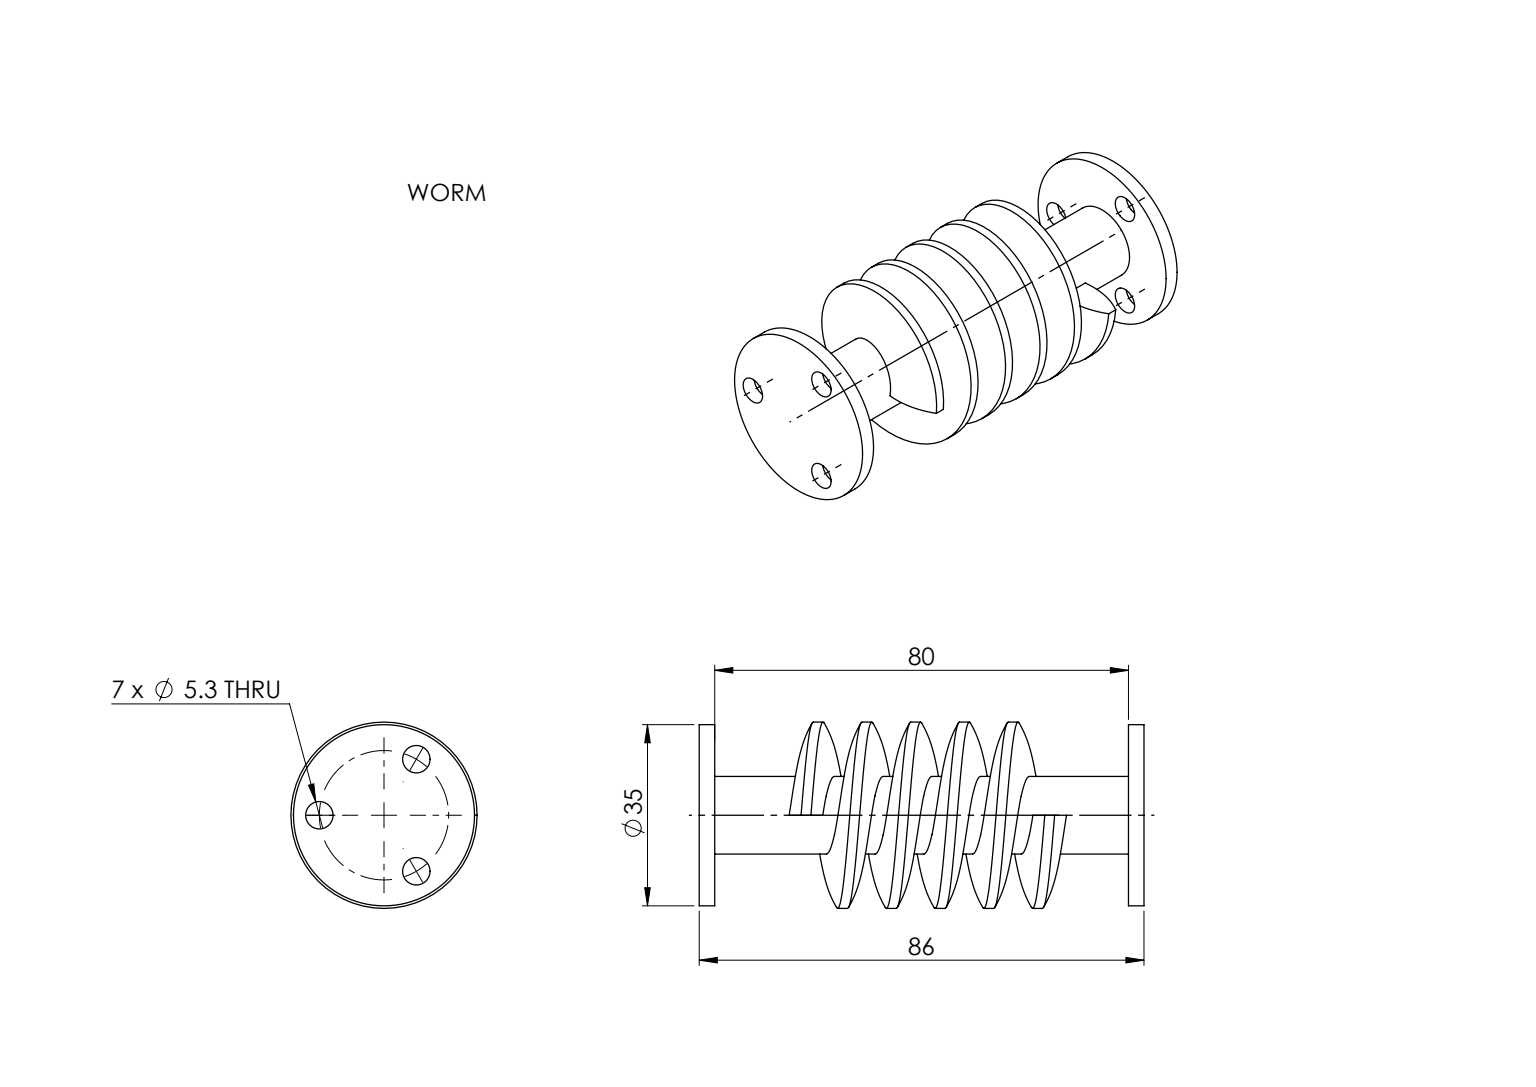
ISO-10303-21;
HEADER;
FILE_DESCRIPTION (('STEP AP214'),
    '1' );
FILE_NAME ('worm.step',
    '2026-10-03T12:29:21',
    ( '' ),
    ( '' ),
    'SwSTEP 2.0',
    'SolidWorks 2026',
    '' );
FILE_SCHEMA (( 'AUTOMOTIVE_DESIGN' ));
ENDSEC;

DATA;
#2=CARTESIAN_POINT ( 'NONE',  ( -6.358192987158596488, 4.248408730893249441, 12.23479375018031590 ) ) ;
#4=CARTESIAN_POINT ( 'NONE',  ( 11.17563879758427525, 2.222972768810836719, -0.3496410002868030609 ) ) ;
#8=DIRECTION ( 'NONE',  ( 0.000000000000000000, 0.000000000000000000, 1.000000000000000000 ) ) ;
#13=CARTESIAN_POINT ( 'NONE',  ( 16.62983158437509346, -6.888301784570739272, 14.47261250018031298 ) ) ;
#31=CARTESIAN_POINT ( 'NONE',  ( -6.358192987158591158, 4.248408730893245000, 5.969893750180312431 ) ) ;
#34=CARTESIAN_POINT ( 'NONE',  ( 6.358192987158596488, -4.248408730893249441, -1.902706249819686279 ) ) ;
#36=CARTESIAN_POINT ( 'NONE',  ( 0.000000000000000000, 0.000000000000000000, 40.00000000000000000 ) ) ;
#40=DIRECTION ( 'NONE',  ( -0.000000000000000000, -0.000000000000000000, -1.000000000000000000 ) ) ;
#43=PLANE ( 'NONE',  #3162 ) ;
#52=CARTESIAN_POINT ( 'NONE',  ( 14.79893867793684059, 2.943691925285398359, -12.82923933115845649 ) ) ;
#57=EDGE_LOOP ( 'NONE', ( #4970, #17934 ) ) ;
#61=CARTESIAN_POINT ( 'NONE',  ( -15.25966317163203279, -10.19618095047498052, 17.71245625018031689 ) ) ;
#69=ORIENTED_EDGE ( 'NONE', *, *, #783, .F. ) ;
#72=CARTESIAN_POINT ( 'NONE',  ( 1.491842756249030399, 7.499999999820669672, -4.848018749819687834 ) ) ;
#76=AXIS2_PLACEMENT_3D ( 'NONE', #4116, #10601, #17063 ) ;
#80=CARTESIAN_POINT ( 'NONE',  ( 3.580422614997669228, 17.99999999956958874, -7.028168749819693417 ) ) ;
#83=CARTESIAN_POINT ( 'NONE',  ( -13.67243654778935102, -5.663308646854334327, -4.604354418480926192 ) ) ;
#94=ORIENTED_EDGE ( 'NONE', *, *, #11160, .T. ) ;
#100=VERTEX_POINT ( 'NONE', #5055 ) ;
#108=CARTESIAN_POINT ( 'NONE',  ( 7.500000000000007994, -9.015933403756345817E-10, 16.06370000018031519 ) ) ;
#110=CARTESIAN_POINT ( 'NONE',  ( -7.902369976724391343, 7.902369978624323110, -3.589484750286802139 ) ) ;
#115=CARTESIAN_POINT ( 'NONE',  ( 3.580422614997668340, 17.99999999956958519, 21.24683125018031404 ) ) ;
#131=AXIS2_PLACEMENT_3D ( 'NONE', #20801, #1327, #6175 ) ;
#135=CARTESIAN_POINT ( 'NONE',  ( 6.358192988180013216, 4.248408729364577141, 8.915206250180313319 ) ) ;
#142=CARTESIAN_POINT ( 'NONE',  ( -10.19618095047498052, 15.25966317163203101, 18.16410625018031411 ) ) ;
#156=CARTESIAN_POINT ( 'NONE',  ( 14.79893867722910450, -2.943691928843438443, -21.66517683115846182 ) ) ;
#174=CARTESIAN_POINT ( 'NONE',  ( 3.580422610670019878, -18.00000000043040771, -23.65933124981969016 ) ) ;
#177=CARTESIAN_POINT ( 'NONE',  ( 7.500000000000005329, -1.491842755816077393, -11.91676874991220814 ) ) ;
#181=( BOUNDED_SURFACE ( )  B_SPLINE_SURFACE ( 3, 2, ( 
 ( #15242, #3787, #10269, #14938, #18223, #10163, #15145, #724, #8565, #15045, #7180, #2419, #20112, #5588, #10480, #8880, #15353, #840, #7288, #20223, #5698, #2009, #8458, #415, #19801, #11758, #3688, #525, #10588, #12389, #19166, #10700, #7396, #13983, #7499, #17264, #953, #20642, #4431, #1375, #14091, #20319, #7820, #14300, #10899, #18755, #20742, #2956, #17050, #20545, #11002, #18960, #15464, #13872, #17372, #6229, #17163, #6121, #6028, #4541, #2736, #2648, #4336, #12599, #20438, #15878, #5920, #12498, #9205, #19066, #10803, #4224, #17479, #5803, #2537, #18861, #9423, #15665, #1165, #2844, #7613, #9311, #9104, #15774, #12280, #15556, #1276, #12714, #7727, #8994, #1052, #14200, #1778, #4745, #13122, #17792, #9820, #6336, #4647, #14602, #19572, #12822, #16391, #80, #17688, #13019, #3358, #3456, #16196, #16092, #1878, #287, #1683, #5049, #19266, #9516, #3258, #6736, #8232, #9923, #14710, #4852, #20850, #11115, #182, #9728, #1583, #8130, #7931, #8037, #8336, #3157, #6430, #14732, #11212, #16287, #17985, #17586, #6534, #1483, #13219, #12913, #14814, #11512, #19365, #19471, #3054, #6637, #9629, #4953, #15981, #14408, #11323, #11423, #17896, #14513, #5561, #13532, #384, #608, #3977 ),
 ( #813, #3666, #5147, #8432, #501, #10348, #15327, #16915, #13325, #7052, #10457, #11621, #13635, #3757, #8752, #19976, #10138, #16590, #18095, #6840, #19779, #6949, #11829, #5261, #18201, #8536, #20082, #10239, #2079, #15218, #5456, #18293, #11928, #12042, #15017, #18513, #13434, #2395, #19887, #5361, #16701, #3560, #18402, #19667, #2186, #7259, #11730, #16505, #8643, #8852, #15121, #3869, #16813, #700, #2299, #7152, #10037, #14908, #1984, #9079, #2817, #5895, #2616, #7588, #15531, #1025, #5775, #20517, #15431, #8966, #17238, #2927, #2510, #4403, #20194, #10871, #12145, #17342, #4077, #1350, #12367, #15636, #921, #20616, #13847, #7370, #7471, #20291, #17454, #18833, #9397, #4307, #5674, #10777, #2710, #12248, #13953, #15857, #18723, #18614, #4197, #20408, #9287, #13740, #10978, #10675, #1136, #19036, #10557, #7700, #9177, #15748, #14066, #17133, #5999, #17023, #12471, #18935, #1247, #14176, #6092, #12569, #4512, #8205, #12891, #4722, #3337, #16172, #6407, #52, #14684, #11187, #1753, #9596, #19550, #19244, #17659, #16064, #14268, #8110, #7794, #1557, #16368, #7902, #4619, #3127, #8009, #14489, #19145, #17874, #1661, #5030, #11291, #17564, #11491, #17963, #14582, #15950, #3432, #156, #20713 ),
 ( #6506, #9900, #14384, #9797, #17766, #6609, #20929, #20825, #19339, #16266, #4822, #6203, #3232, #12688, #6307, #11091, #9703, #12992, #19445, #3031, #13094, #4926, #9491, #11395, #1450, #12798, #5539, #16678, #10008, #12017, #15197, #10434, #11807, #2272, #10215, #6715, #19644, #2167, #18484, #8411, #18375, #18270, #16784, #14991, #1960, #16568, #11902, #5237, #7127, #18175, #5339, #479, #3845, #2055, #16477, #8731, #18071, #8310, #3642, #10324, #6926, #11707, #8621, #10116, #8510, #14884, #15095, #3536, #361, #3735, #3951, #11596, #13512, #14785, #19955, #264, #5433, #13196, #1856, #13410, #583, #6814, #675, #13298, #19756, #19862, #7033, #5122, #13608, #20055, #1305, #8824, #7748, #9337, #15408, #18696, #19287, #894, #2371, #5650, #4169, #7848, #12843, #14436, #10535, #19097, #1512, #15297, #11138, #14221, #6259, #4570, #7348, #13829, #785, #18593, #16994, #10652, #15801, #2480, #20272, #5750, #17608, #20666, #12226, #12743, #11032, #6148, #9444, #3078, #17107, #9541, #2871, #7963, #12636, #17509, #2983, #7234, #15902, #1400, #19196, #14331, #20776, #4676, #16012, #20881, #6363, #4770, #16894, #13717, #20164, #12125, #4053, #8942, #11237, #13045, #19804, #11351, #8068, #14629, #8156 ),
 ( #19699, #3383, #16418, #12942, #17715, #212, #5180, #19393, #2012, #6669, #3294, #19602, #9954, #10066, #1809, #1707, #8461, #6871, #8261, #11650, #4882, #16123, #9849, #13357, #8369, #16528, #14841, #11455, #6457, #3188, #6767, #16314, #108, #14735, #14537, #6563, #14942, #9758, #19499, #4987, #17823, #1905, #3590, #9657, #13152, #2, #1615, #17923, #418, #18122, #5076, #11542, #16223, #315, #18013, #3480, #13248, #15359, #5486, #7077, #12076, #15047, #12173, #20116, #6975, #7183, #10591, #8571, #958, #528, #18226, #13667, #5700, #18546, #13777, #16624, #10379, #2321, #16844, #7398, #11965, #15244, #2216, #13464, #8674, #7294, #18435, #13556, #15147, #8775, #13876, #632, #5594, #4001, #20227, #10164, #3898, #18323, #15467, #727, #19908, #10483, #2421, #5386, #18639, #16939, #8882, #11855, #5288, #842, #4107, #3790, #17054, #2540, #10273, #8999, #11760, #3692, #2112, #16736, #20004, #15983, #10900, #20745, #13984, #4225, #12499, #1485, #17480, #19168, #2958, #20547, #15560, #20320, #15879, #18963, #10805, #17374, #2650, #17269, #11116, #12392, #1169, #15666, #20443, #11003, #12716, #5805, #9312, #17166, #7936, #7614, #3055, #7821, #14093, #4434, #4650, #9424, #5921, #2847, #1376 ) ),
 .UNSPECIFIED., .F., .F., .F. ) 
 B_SPLINE_SURFACE_WITH_KNOTS ( ( 4, 4 ),
 ( 3, 2, 2, 2, 2, 2, 2, 2, 2, 2, 2, 2, 2, 2, 2, 2, 2, 2, 2, 2, 2, 2, 2, 2, 2, 2, 2, 2, 2, 2, 2, 2, 2, 2, 2, 2, 2, 2, 2, 2, 2, 2, 2, 2, 2, 2, 2, 2, 2, 2, 2, 2, 2, 2, 2, 2, 2, 2, 2, 2, 2, 2, 2, 2, 2, 2, 2, 2, 2, 2, 2, 2, 2, 2, 2, 2, 2, 2, 2, 2, 3 ),
 ( 0.000000000000000000, 1.000000000000000000 ),
 ( 0.000000000000000000, 0.01250000000000000069, 0.02500000000000000139, 0.03749999999999999861, 0.05000000000000000278, 0.06250000000000000000, 0.07499999999999999722, 0.08749999999999999445, 0.1000000000000000056, 0.1125000000000000028, 0.1250000000000000000, 0.1375000000000000111, 0.1499999999999999944, 0.1625000000000000056, 0.1749999999999999889, 0.1875000000000000000, 0.2000000000000000111, 0.2124999999999999944, 0.2250000000000000056, 0.2374999999999999889, 0.2500000000000000000, 0.2625000000000000111, 0.2750000000000000222, 0.2874999999999999778, 0.2999999999999999889, 0.3125000000000000000, 0.3250000000000000111, 0.3375000000000000222, 0.3499999999999999778, 0.3624999999999999889, 0.3750000000000000000, 0.3875000000000000111, 0.4000000000000000222, 0.4124999999999999778, 0.4249999999999999889, 0.4375000000000000000, 0.4500000000000000111, 0.4625000000000000222, 0.4749999999999999778, 0.4874999999999999889, 0.5000000000000000000, 0.5124999999999999556, 0.5250000000000000222, 0.5374999999999999778, 0.5500000000000000444, 0.5625000000000000000, 0.5749999999999999556, 0.5875000000000000222, 0.5999999999999999778, 0.6125000000000000444, 0.6250000000000000000, 0.6374999999999999556, 0.6500000000000000222, 0.6624999999999999778, 0.6750000000000000444, 0.6875000000000000000, 0.6999999999999999556, 0.7125000000000000222, 0.7249999999999999778, 0.7375000000000000444, 0.7500000000000000000, 0.7624999999999999556, 0.7750000000000000222, 0.7874999999999999778, 0.8000000000000000444, 0.8125000000000000000, 0.8249999999999999556, 0.8375000000000000222, 0.8499999999999999778, 0.8625000000000000444, 0.8750000000000000000, 0.8874999999999999556, 0.9000000000000000222, 0.9124999999999999778, 0.9250000000000000444, 0.9375000000000000000, 0.9499999999999999556, 0.9625000000000000222, 0.9749999999999999778, 0.9875000000000000444, 1.000000000000000000 ),
 .UNSPECIFIED. ) 
 GEOMETRIC_REPRESENTATION_ITEM ( )  RATIONAL_B_SPLINE_SURFACE ( (
 ( 1.000000000000000000, 0.9807852804032304306, 1.000000000000000000, 0.9807852804032304306, 1.000000000000000000, 0.9807852804032304306, 1.000000000000000000, 0.9807852804032304306, 1.000000000000000000, 0.9807852804032304306, 1.000000000000000000, 0.9807852804032304306, 1.000000000000000000, 0.9807852804032304306, 1.000000000000000000, 0.9807852804032304306, 1.000000000000000000, 0.9807852804032304306, 1.000000000000000000, 0.9807852804032304306, 1.000000000000000000, 0.9807852804032304306, 1.000000000000000000, 0.9807852804032304306, 1.000000000000000000, 0.9807852804032304306, 1.000000000000000000, 0.9807852804032304306, 1.000000000000000000, 0.9807852804032304306, 1.000000000000000000, 0.9807852804032304306, 1.000000000000000000, 0.9807852804032304306, 1.000000000000000000, 0.9807852804032304306, 1.000000000000000000, 0.9807852804032304306, 1.000000000000000000, 0.9807852804032304306, 1.000000000000000000, 0.9807852804032304306, 1.000000000000000000, 0.9807852804032304306, 1.000000000000000000, 0.9807852804032304306, 1.000000000000000000, 0.9807852804032304306, 1.000000000000000000, 0.9807852804032304306, 1.000000000000000000, 0.9807852804032304306, 1.000000000000000000, 0.9807852804032304306, 1.000000000000000000, 0.9807852804032304306, 1.000000000000000000, 0.9807852804032304306, 1.000000000000000000, 0.9807852804032304306, 1.000000000000000000, 0.9807852804032304306, 1.000000000000000000, 0.9807852804032304306, 1.000000000000000000, 0.9807852804032304306, 1.000000000000000000, 0.9807852804032304306, 1.000000000000000000, 0.9807852804032304306, 1.000000000000000000, 0.9807852804032304306, 1.000000000000000000, 0.9807852804032304306, 1.000000000000000000, 0.9807852804032304306, 1.000000000000000000, 0.9807852804032304306, 1.000000000000000000, 0.9807852804032304306, 1.000000000000000000, 0.9807852804032304306, 1.000000000000000000, 0.9807852804032304306, 1.000000000000000000, 0.9807852804032304306, 1.000000000000000000, 0.9807852804032304306, 1.000000000000000000, 0.9807852804032304306, 1.000000000000000000, 0.9807852804032304306, 1.000000000000000000, 0.9807852804032304306, 1.000000000000000000, 0.9807852804032304306, 1.000000000000000000, 0.9807852804032304306, 1.000000000000000000, 0.9807852804032304306, 1.000000000000000000, 0.9807852804032304306, 1.000000000000000000, 0.9807852804032304306, 1.000000000000000000, 0.9807852804032304306, 1.000000000000000000, 0.9807852804032304306, 1.000000000000000000, 0.9807852804032304306, 1.000000000000000000, 0.9807852804032304306, 1.000000000000000000, 0.9807852804032304306, 1.000000000000000000, 0.9807852804032304306, 1.000000000000000000, 0.9807852804032304306, 1.000000000000000000, 0.9807852804032304306, 1.000000000000000000, 0.9807852804032304306, 1.000000000000000000, 0.9807852804032304306, 1.000000000000000000, 0.9807852804032304306, 1.000000000000000000, 0.9807852804032304306, 1.000000000000000000, 0.9807852804032304306, 1.000000000000000000, 0.9807852804032304306, 1.000000000000000000, 0.9807852804032304306, 1.000000000000000000, 0.9807852804032304306, 1.000000000000000000, 0.9807852804032304306, 1.000000000000000000, 0.9807852804032304306, 1.000000000000000000, 0.9807852804032304306, 1.000000000000000000, 0.9807852804032304306, 1.000000000000000000, 0.9807852804032304306, 1.000000000000000000, 0.9807852804032304306, 1.000000000000000000, 0.9807852804032304306, 1.000000000000000000, 0.9807852804032304306, 1.000000000000000000, 0.9807852804032304306, 1.000000000000000000, 0.9807852804032304306, 1.000000000000000000, 0.9807852804032304306, 1.000000000000000000, 0.9807852804032304306, 1.000000000000000000),
 ( 0.9659702800374152520, 0.9474094319676833464, 0.9659702800374152520, 0.9474094319676833464, 0.9659702800374152520, 0.9474094319676833464, 0.9659702800374152520, 0.9474094319676833464, 0.9659702800374152520, 0.9474094319676833464, 0.9659702800374152520, 0.9474094319676833464, 0.9659702800374152520, 0.9474094319676833464, 0.9659702800374152520, 0.9474094319676833464, 0.9659702800374152520, 0.9474094319676833464, 0.9659702800374152520, 0.9474094319676833464, 0.9659702800374152520, 0.9474094319676833464, 0.9659702800374152520, 0.9474094319676833464, 0.9659702800374152520, 0.9474094319676833464, 0.9659702800374152520, 0.9474094319676833464, 0.9659702800374152520, 0.9474094319676833464, 0.9659702800374152520, 0.9474094319676833464, 0.9659702800374152520, 0.9474094319676833464, 0.9659702800374152520, 0.9474094319676833464, 0.9659702800374152520, 0.9474094319676833464, 0.9659702800374152520, 0.9474094319676833464, 0.9659702800374152520, 0.9474094319676833464, 0.9659702800374152520, 0.9474094319676833464, 0.9659702800374152520, 0.9474094319676833464, 0.9659702800374152520, 0.9474094319676833464, 0.9659702800374152520, 0.9474094319676833464, 0.9659702800374152520, 0.9474094319676833464, 0.9659702800374152520, 0.9474094319676833464, 0.9659702800374152520, 0.9474094319676833464, 0.9659702800374152520, 0.9474094319676833464, 0.9659702800374152520, 0.9474094319676833464, 0.9659702800374152520, 0.9474094319676833464, 0.9659702800374152520, 0.9474094319676833464, 0.9659702800374152520, 0.9474094319676833464, 0.9659702800374152520, 0.9474094319676833464, 0.9659702800374152520, 0.9474094319676833464, 0.9659702800374152520, 0.9474094319676833464, 0.9659702800374152520, 0.9474094319676833464, 0.9659702800374152520, 0.9474094319676833464, 0.9659702800374152520, 0.9474094319676833464, 0.9659702800374152520, 0.9474094319676833464, 0.9659702800374152520, 0.9474094319676833464, 0.9659702800374152520, 0.9474094319676833464, 0.9659702800374152520, 0.9474094319676833464, 0.9659702800374152520, 0.9474094319676833464, 0.9659702800374152520, 0.9474094319676833464, 0.9659702800374152520, 0.9474094319676833464, 0.9659702800374152520, 0.9474094319676833464, 0.9659702800374152520, 0.9474094319676833464, 0.9659702800374152520, 0.9474094319676833464, 0.9659702800374152520, 0.9474094319676833464, 0.9659702800374152520, 0.9474094319676833464, 0.9659702800374152520, 0.9474094319676833464, 0.9659702800374152520, 0.9474094319676833464, 0.9659702800374152520, 0.9474094319676833464, 0.9659702800374152520, 0.9474094319676833464, 0.9659702800374152520, 0.9474094319676833464, 0.9659702800374152520, 0.9474094319676833464, 0.9659702800374152520, 0.9474094319676833464, 0.9659702800374152520, 0.9474094319676833464, 0.9659702800374152520, 0.9474094319676833464, 0.9659702800374152520, 0.9474094319676833464, 0.9659702800374152520, 0.9474094319676833464, 0.9659702800374152520, 0.9474094319676833464, 0.9659702800374152520, 0.9474094319676833464, 0.9659702800374152520, 0.9474094319676833464, 0.9659702800374152520, 0.9474094319676833464, 0.9659702800374152520, 0.9474094319676833464, 0.9659702800374152520, 0.9474094319676833464, 0.9659702800374152520, 0.9474094319676833464, 0.9659702800374152520, 0.9474094319676833464, 0.9659702800374152520, 0.9474094319676833464, 0.9659702800374152520, 0.9474094319676833464, 0.9659702800374152520, 0.9474094319676833464, 0.9659702800374152520, 0.9474094319676833464, 0.9659702800374152520, 0.9474094319676833464, 0.9659702800374152520, 0.9474094319676833464, 0.9659702800374152520, 0.9474094319676833464, 0.9659702800374152520, 0.9474094319676833464, 0.9659702800374152520, 0.9474094319676833464, 0.9659702800374152520, 0.9474094319676833464, 0.9659702800374152520),
 ( 0.9659702800374152520, 0.9474094319676833464, 0.9659702800374152520, 0.9474094319676833464, 0.9659702800374152520, 0.9474094319676833464, 0.9659702800374152520, 0.9474094319676833464, 0.9659702800374152520, 0.9474094319676833464, 0.9659702800374152520, 0.9474094319676833464, 0.9659702800374152520, 0.9474094319676833464, 0.9659702800374152520, 0.9474094319676833464, 0.9659702800374152520, 0.9474094319676833464, 0.9659702800374152520, 0.9474094319676833464, 0.9659702800374152520, 0.9474094319676833464, 0.9659702800374152520, 0.9474094319676833464, 0.9659702800374152520, 0.9474094319676833464, 0.9659702800374152520, 0.9474094319676833464, 0.9659702800374152520, 0.9474094319676833464, 0.9659702800374152520, 0.9474094319676833464, 0.9659702800374152520, 0.9474094319676833464, 0.9659702800374152520, 0.9474094319676833464, 0.9659702800374152520, 0.9474094319676833464, 0.9659702800374152520, 0.9474094319676833464, 0.9659702800374152520, 0.9474094319676833464, 0.9659702800374152520, 0.9474094319676833464, 0.9659702800374152520, 0.9474094319676833464, 0.9659702800374152520, 0.9474094319676833464, 0.9659702800374152520, 0.9474094319676833464, 0.9659702800374152520, 0.9474094319676833464, 0.9659702800374152520, 0.9474094319676833464, 0.9659702800374152520, 0.9474094319676833464, 0.9659702800374152520, 0.9474094319676833464, 0.9659702800374152520, 0.9474094319676833464, 0.9659702800374152520, 0.9474094319676833464, 0.9659702800374152520, 0.9474094319676833464, 0.9659702800374152520, 0.9474094319676833464, 0.9659702800374152520, 0.9474094319676833464, 0.9659702800374152520, 0.9474094319676833464, 0.9659702800374152520, 0.9474094319676833464, 0.9659702800374152520, 0.9474094319676833464, 0.9659702800374152520, 0.9474094319676833464, 0.9659702800374152520, 0.9474094319676833464, 0.9659702800374152520, 0.9474094319676833464, 0.9659702800374152520, 0.9474094319676833464, 0.9659702800374152520, 0.9474094319676833464, 0.9659702800374152520, 0.9474094319676833464, 0.9659702800374152520, 0.9474094319676833464, 0.9659702800374152520, 0.9474094319676833464, 0.9659702800374152520, 0.9474094319676833464, 0.9659702800374152520, 0.9474094319676833464, 0.9659702800374152520, 0.9474094319676833464, 0.9659702800374152520, 0.9474094319676833464, 0.9659702800374152520, 0.9474094319676833464, 0.9659702800374152520, 0.9474094319676833464, 0.9659702800374152520, 0.9474094319676833464, 0.9659702800374152520, 0.9474094319676833464, 0.9659702800374152520, 0.9474094319676833464, 0.9659702800374152520, 0.9474094319676833464, 0.9659702800374152520, 0.9474094319676833464, 0.9659702800374152520, 0.9474094319676833464, 0.9659702800374152520, 0.9474094319676833464, 0.9659702800374152520, 0.9474094319676833464, 0.9659702800374152520, 0.9474094319676833464, 0.9659702800374152520, 0.9474094319676833464, 0.9659702800374152520, 0.9474094319676833464, 0.9659702800374152520, 0.9474094319676833464, 0.9659702800374152520, 0.9474094319676833464, 0.9659702800374152520, 0.9474094319676833464, 0.9659702800374152520, 0.9474094319676833464, 0.9659702800374152520, 0.9474094319676833464, 0.9659702800374152520, 0.9474094319676833464, 0.9659702800374152520, 0.9474094319676833464, 0.9659702800374152520, 0.9474094319676833464, 0.9659702800374152520, 0.9474094319676833464, 0.9659702800374152520, 0.9474094319676833464, 0.9659702800374152520, 0.9474094319676833464, 0.9659702800374152520, 0.9474094319676833464, 0.9659702800374152520, 0.9474094319676833464, 0.9659702800374152520, 0.9474094319676833464, 0.9659702800374152520, 0.9474094319676833464, 0.9659702800374152520, 0.9474094319676833464, 0.9659702800374152520, 0.9474094319676833464, 0.9659702800374152520, 0.9474094319676833464, 0.9659702800374152520),
 ( 1.000000000000000000, 0.9807852804032304306, 1.000000000000000000, 0.9807852804032304306, 1.000000000000000000, 0.9807852804032304306, 1.000000000000000000, 0.9807852804032304306, 1.000000000000000000, 0.9807852804032304306, 1.000000000000000000, 0.9807852804032304306, 1.000000000000000000, 0.9807852804032304306, 1.000000000000000000, 0.9807852804032304306, 1.000000000000000000, 0.9807852804032304306, 1.000000000000000000, 0.9807852804032304306, 1.000000000000000000, 0.9807852804032304306, 1.000000000000000000, 0.9807852804032304306, 1.000000000000000000, 0.9807852804032304306, 1.000000000000000000, 0.9807852804032304306, 1.000000000000000000, 0.9807852804032304306, 1.000000000000000000, 0.9807852804032304306, 1.000000000000000000, 0.9807852804032304306, 1.000000000000000000, 0.9807852804032304306, 1.000000000000000000, 0.9807852804032304306, 1.000000000000000000, 0.9807852804032304306, 1.000000000000000000, 0.9807852804032304306, 1.000000000000000000, 0.9807852804032304306, 1.000000000000000000, 0.9807852804032304306, 1.000000000000000000, 0.9807852804032304306, 1.000000000000000000, 0.9807852804032304306, 1.000000000000000000, 0.9807852804032304306, 1.000000000000000000, 0.9807852804032304306, 1.000000000000000000, 0.9807852804032304306, 1.000000000000000000, 0.9807852804032304306, 1.000000000000000000, 0.9807852804032304306, 1.000000000000000000, 0.9807852804032304306, 1.000000000000000000, 0.9807852804032304306, 1.000000000000000000, 0.9807852804032304306, 1.000000000000000000, 0.9807852804032304306, 1.000000000000000000, 0.9807852804032304306, 1.000000000000000000, 0.9807852804032304306, 1.000000000000000000, 0.9807852804032304306, 1.000000000000000000, 0.9807852804032304306, 1.000000000000000000, 0.9807852804032304306, 1.000000000000000000, 0.9807852804032304306, 1.000000000000000000, 0.9807852804032304306, 1.000000000000000000, 0.9807852804032304306, 1.000000000000000000, 0.9807852804032304306, 1.000000000000000000, 0.9807852804032304306, 1.000000000000000000, 0.9807852804032304306, 1.000000000000000000, 0.9807852804032304306, 1.000000000000000000, 0.9807852804032304306, 1.000000000000000000, 0.9807852804032304306, 1.000000000000000000, 0.9807852804032304306, 1.000000000000000000, 0.9807852804032304306, 1.000000000000000000, 0.9807852804032304306, 1.000000000000000000, 0.9807852804032304306, 1.000000000000000000, 0.9807852804032304306, 1.000000000000000000, 0.9807852804032304306, 1.000000000000000000, 0.9807852804032304306, 1.000000000000000000, 0.9807852804032304306, 1.000000000000000000, 0.9807852804032304306, 1.000000000000000000, 0.9807852804032304306, 1.000000000000000000, 0.9807852804032304306, 1.000000000000000000, 0.9807852804032304306, 1.000000000000000000, 0.9807852804032304306, 1.000000000000000000, 0.9807852804032304306, 1.000000000000000000, 0.9807852804032304306, 1.000000000000000000, 0.9807852804032304306, 1.000000000000000000, 0.9807852804032304306, 1.000000000000000000, 0.9807852804032304306, 1.000000000000000000, 0.9807852804032304306, 1.000000000000000000, 0.9807852804032304306, 1.000000000000000000, 0.9807852804032304306, 1.000000000000000000, 0.9807852804032304306, 1.000000000000000000, 0.9807852804032304306, 1.000000000000000000, 0.9807852804032304306, 1.000000000000000000, 0.9807852804032304306, 1.000000000000000000, 0.9807852804032304306, 1.000000000000000000, 0.9807852804032304306, 1.000000000000000000, 0.9807852804032304306, 1.000000000000000000, 0.9807852804032304306, 1.000000000000000000, 0.9807852804032304306, 1.000000000000000000, 0.9807852804032304306, 1.000000000000000000, 0.9807852804032304306, 1.000000000000000000) ) ) 
 REPRESENTATION_ITEM ( '' )  SURFACE ( )  );
#182=CARTESIAN_POINT ( 'NONE',  ( 12.72792205982779912, -12.72792206288791483, -13.21332499981969022 ) ) ;
#185=DIRECTION ( 'NONE',  ( 1.000000000000000000, 0.000000000000000000, 0.000000000000000000 ) ) ;
#186=CARTESIAN_POINT ( 'NONE',  ( 1.779017513685135741E-09, 14.79893867758296544, -1.659041918480926858 ) ) ;
#197=VERTEX_POINT ( 'NONE', #8975 ) ;
#212=CARTESIAN_POINT ( 'NONE',  ( 4.248408730893249441, 6.358192987158595599, 24.01604375018031945 ) ) ;
#213=CARTESIAN_POINT ( 'NONE',  ( -2.222972771497743416, -11.17563879704981566, 12.02067149971319893 ) ) ;
#218=EDGE_LOOP ( 'NONE', ( #4264, #16407, #7924, #14163 ) ) ;
#221=CARTESIAN_POINT ( 'NONE',  ( 2.163825119083639534E-09, 18.00000000000000000, 11.52730000018031298 ) ) ;
#234=( LENGTH_UNIT ( ) NAMED_UNIT ( * ) SI_UNIT ( .MILLI., .METRE. ) );
#240=AXIS2_PLACEMENT_3D ( 'NONE', #14283, #9409, #6012 ) ;
#241=CARTESIAN_POINT ( 'NONE',  ( -7.499999999820661678, 1.491842756249031288, 14.80583125018031154 ) ) ;
#244=DIRECTION ( 'NONE',  ( 1.000000000000000000, 0.000000000000000000, 0.000000000000000000 ) ) ;
#264=CARTESIAN_POINT ( 'NONE',  ( -6.330490856366295382, 9.474249098604511587, 3.827766000647429667 ) ) ;
#271=DIRECTION ( 'NONE',  ( -0.000000000000000000, -0.000000000000000000, -1.000000000000000000 ) ) ;
#275=CARTESIAN_POINT ( 'NONE',  ( 10.19618095047497874, -15.25966317163203279, 15.35620625018031404 ) ) ;
#287=CARTESIAN_POINT ( 'NONE',  ( -17.99999999956958874, 3.580422614997675002, -9.384418749819689154 ) ) ;
#290=CARTESIAN_POINT ( 'NONE',  ( 1.491842756249029289, 7.499999999820664343, 7.737081250180308345 ) ) ;
#293=CARTESIAN_POINT ( 'NONE',  ( 14.79893867793683349, 2.943691925285396582, 0.4026768315190735747 ) ) ;
#294=EDGE_CURVE ( 'NONE', #19785, #7832, #9854, .T. ) ;
#300=CARTESIAN_POINT ( 'NONE',  ( 4.248408730893246776, 6.358192987158592047, 17.75114375018031154 ) ) ;
#315=CARTESIAN_POINT ( 'NONE',  ( -4.248408730893249441, -6.358192987158595599, 9.878543750180314831 ) ) ;
#317=CARTESIAN_POINT ( 'NONE',  ( 10.32494394706615637, -4.276731815070946574, 9.958952749713198216 ) ) ;
#322=CARTESIAN_POINT ( 'NONE',  ( 15.25966316918061416, -10.19618095414378622, 14.76714375018031333 ) ) ;
#330=ADVANCED_FACE ( 'NONE', ( #4521 ), #3038, .T. ) ;
#334=SURFACE_STYLE_USAGE ( .BOTH. , #6692 ) ;
#338=CARTESIAN_POINT ( 'NONE',  ( 7.500000000179339210, 1.491842754445841690, 9.504268750180312253 ) ) ;
#344=CARTESIAN_POINT ( 'NONE',  ( 2.870125743571140475, 6.929096493489632635, 4.871512500180315008 ) ) ;
#346=CARTESIAN_POINT ( 'NONE',  ( 2.163825119083639534E-09, 18.00000000000000000, 19.04770000018031340 ) ) ;
#355=EDGE_CURVE ( 'NONE', #16003, #19785, #20624, .T. ) ;
#357=AXIS2_PLACEMENT_3D ( 'NONE', #9156, #15411, #7774 ) ;
#358=CARTESIAN_POINT ( 'NONE',  ( 2.870125743571138255, 6.929096493489627306, -10.81838749981969450 ) ) ;
#361=CARTESIAN_POINT ( 'NONE',  ( 7.902369978624329327, 7.902369976724401113, 5.889484750647431710 ) ) ;
#362=ORIENTED_EDGE ( 'NONE', *, *, #16789, .T. ) ;
#369=CARTESIAN_POINT ( 'NONE',  ( 18.00000000043041126, 3.580422610670019434, 13.58901875018031369 ) ) ;
#370=CARTESIAN_POINT ( 'NONE',  ( -9.850000000000006750, 0.000000000000000000, -43.00000000000000000 ) ) ;
#384=CARTESIAN_POINT ( 'NONE',  ( 16.62983158437509701, -6.888301784570740161, -23.22738749981969519 ) ) ;
#388=EDGE_CURVE ( 'NONE', #1886, #2751, #11934, .T. ) ;
#392=CARTESIAN_POINT ( 'NONE',  ( 2.943691928843430450, 14.79893867722910095, -20.21451066848093703 ) ) ;
#403=CARTESIAN_POINT ( 'NONE',  ( 6.250000000000054179, 10.82531754730546147, 40.00000000000000000 ) ) ;
#404=CARTESIAN_POINT ( 'NONE',  ( 6.888301780572505528, -16.62983158603121581, 4.321137500180309843 ) ) ;
#415=CARTESIAN_POINT ( 'NONE',  ( -3.580422614997675890, -17.99999999956958519, 16.53433125018031191 ) ) ;
#418=CARTESIAN_POINT ( 'NONE',  ( -7.500000000000007994, 9.015942588607339023E-10, 11.35120000018031661 ) ) ;
#421=CARTESIAN_POINT ( 'NONE',  ( -4.276731815070945686, -10.32494394706615637, 2.890202749713199459 ) ) ;
#428=CARTESIAN_POINT ( 'NONE',  ( 3.580422610670020322, -18.00000000043041126, 15.94526875018031298 ) ) ;
#451=CARTESIAN_POINT ( 'NONE',  ( 4.248408730893245888, 6.358192987158590270, 17.75114375018031510 ) ) ;
#468=AXIS2_PLACEMENT_3D ( 'NONE', #13809, #3821, #7105 ) ;
#473=CARTESIAN_POINT ( 'NONE',  ( -10.19618095047497874, 15.25966317163202746, -10.11089374981968980 ) ) ;
#479=CARTESIAN_POINT ( 'NONE',  ( -9.474249098604513364, -6.330490856366295382, 10.89651600064742887 ) ) ;
#488=CARTESIAN_POINT ( 'NONE',  ( 15.25966317163202746, 10.19618095047498407, 12.99995625018031475 ) ) ;
#490=PLANE ( 'NONE',  #10357 ) ;
#498=CARTESIAN_POINT ( 'NONE',  ( 7.500000000000000000, 9.184850993605147944E-16, 40.00000000000000000 ) ) ;
#501=CARTESIAN_POINT ( 'NONE',  ( 10.46442989454075700, 10.46442989202484419, 23.98716691884155239 ) ) ;
#504=EDGE_CURVE ( 'NONE', #197, #10395, #14123, .T. ) ;
#506=( NAMED_UNIT ( * ) PLANE_ANGLE_UNIT ( ) SI_UNIT ( $, .RADIAN. ) );
#507=CARTESIAN_POINT ( 'NONE',  ( 18.00000000043040771, 3.580422610670018546, 21.10941875018031055 ) ) ;
#518=CARTESIAN_POINT ( 'NONE',  ( 17.99999999999999645, -2.163824016901520184E-09, 2.553950000180309932 ) ) ;
#522=EDGE_CURVE ( 'NONE', #9436, #1433, #1651, .T. ) ;
#523=LINE ( 'NONE', #11956, #5988 ) ;
#525=CARTESIAN_POINT ( 'NONE',  ( 10.19618095047498052, -15.25966317163203456, 15.35620625018031049 ) ) ;
#527=DIRECTION ( 'NONE',  ( -1.000000000000000000, 0.000000000000000000, 0.000000000000000000 ) ) ;
#528=CARTESIAN_POINT ( 'NONE',  ( 4.248408730893249441, 6.358192987158595599, 5.166043750180316252 ) ) ;
#530=CARTESIAN_POINT ( 'NONE',  ( -4.276731812588563386, 10.32494394809438987, -12.42542225028680214 ) ) ;
#538=CARTESIAN_POINT ( 'NONE',  ( 10.19618095414378800, 15.25966316918061416, 2.985893750180313333 ) ) ;
#555=CARTESIAN_POINT ( 'NONE',  ( -9.015947181032828388E-10, -7.500000000000000888, -6.694949999819691300 ) ) ;
#556=AXIS2_PLACEMENT_3D ( 'NONE', #16543, #2028, #19617 ) ;
#567=CARTESIAN_POINT ( 'NONE',  ( -3.580422610670018546, 18.00000000043041126, 9.328168750180314106 ) ) ;
#570=CARTESIAN_POINT ( 'NONE',  ( 0.000000000000000000, 0.000000000000000000, -40.00000000000000000 ) ) ;
#579=CARTESIAN_POINT ( 'NONE',  ( -12.72792205982779556, 12.72792206288790773, -0.9804249998196894467 ) ) ;
#583=CARTESIAN_POINT ( 'NONE',  ( -11.17563879731705789, 1.343452237168309506E-09, 2.355109750647427891 ) ) ;
#592=CARTESIAN_POINT ( 'NONE',  ( -6.888301784570738384, -16.62983158437509346, -2.021137499819688266 ) ) ;
#597=CARTESIAN_POINT ( 'NONE',  ( -6.929096493489632635, 2.870125743571140919, 11.94026250018031554 ) ) ;
#605=VECTOR ( 'NONE', #19751, 1000.000000000000000 ) ;
#608=CARTESIAN_POINT ( 'NONE',  ( 17.99999999956958519, -3.580422614997676778, -23.52191874981969733 ) ) ;
#614=CARTESIAN_POINT ( 'NONE',  ( 8.382925371439627682, 12.54593441562639988, -19.62544816848093276 ) ) ;
#623=CARTESIAN_POINT ( 'NONE',  ( 12.72792205982779379, -12.72792206288790950, 3.732075000180308688 ) ) ;
#626=ORIENTED_EDGE ( 'NONE', *, *, #13110, .T. ) ;
#632=CARTESIAN_POINT ( 'NONE',  ( 4.248408729364579806, -6.358192988180021210, -1.313643749819685347 ) ) ;
#633=CARTESIAN_POINT ( 'NONE',  ( 2.222972768810837163, -11.17563879758427525, -7.418391000286802317 ) ) ;
#637=CARTESIAN_POINT ( 'NONE',  ( -12.72792206288791128, -12.72792205982779912, -1.432074999819687333 ) ) ;
#651=CARTESIAN_POINT ( 'NONE',  ( -6.929096494179677101, -2.870125741905209527, -4.927762499819687392 ) ) ;
#660=CARTESIAN_POINT ( 'NONE',  ( -16.62983158437510056, 6.888301784570729502, -1.569487499819687049 ) ) ;
#664=ORIENTED_EDGE ( 'NONE', *, *, #16789, .F. ) ;
#667=ORIENTED_EDGE ( 'NONE', *, *, #13110, .F. ) ;
#670=CARTESIAN_POINT ( 'NONE',  ( 10.19618095047497697, -15.25966317163202923, -14.82339374981968838 ) ) ;
#675=CARTESIAN_POINT ( 'NONE',  ( -10.32494394809439875, -4.276731812588566051, 1.766047250647429845 ) ) ;
#684=CARTESIAN_POINT ( 'NONE',  ( 16.62983158437509346, -6.888301784570739272, 14.47261250018031298 ) ) ;
#693=EDGE_CURVE ( 'NONE', #6207, #18276, #2473, .T. ) ;
#696=DIRECTION ( 'NONE',  ( -1.000000000000000000, 0.000000000000000000, 0.000000000000000000 ) ) ;
#700=CARTESIAN_POINT ( 'NONE',  ( -8.382925371439629458, -12.54593441562640876, 9.555135668841547414 ) ) ;
#705=CARTESIAN_POINT ( 'NONE',  ( 13.67243654642774686, -5.663308650141536837, -17.56372941848092850 ) ) ;
#710=CARTESIAN_POINT ( 'NONE',  ( 7.500000000000000888, -9.015933403756337545E-10, 19.22380000018031154 ) ) ;
#716=CARTESIAN_POINT ( 'NONE',  ( -17.99999999956958163, 3.580422614997673669, -1.864018749819690957 ) ) ;
#724=CARTESIAN_POINT ( 'NONE',  ( 3.580422614997669228, 17.99999999956958874, 21.24683125018031049 ) ) ;
#726=CARTESIAN_POINT ( 'NONE',  ( 0.000000000000000000, 0.000000000000000000, 40.00000000000000000 ) ) ;
#727=CARTESIAN_POINT ( 'NONE',  ( 6.358192988180019434, 4.248408729364581582, -3.669893749819685969 ) ) ;
#731=CARTESIAN_POINT ( 'NONE',  ( 2.222972768810837163, -11.17563879758427525, -16.84339100028680036 ) ) ;
#733=( BOUNDED_CURVE ( )  B_SPLINE_CURVE ( 2, ( #13842, #9074, #18392, #5667, #18606, #12139, #17233, #13732, #10551, #18502, #2287, #16909, #20182, #8744, #597, #4067, #2499 ),
 .UNSPECIFIED., .F., .T. ) 
 B_SPLINE_CURVE_WITH_KNOTS ( ( 3, 2, 2, 2, 2, 2, 2, 2, 3 ),
 ( 0.2000000000038511805, 0.2125000000038511638, 0.2250000000038511749, 0.2375000000038511860, 0.2500000000038511971, 0.2625000000038512082, 0.2750000000038512193, 0.2875000000038511749, 0.3000000000038511860 ),
 .UNSPECIFIED. ) 
 CURVE ( )  GEOMETRIC_REPRESENTATION_ITEM ( )  RATIONAL_B_SPLINE_CURVE ( ( 0.9999999999940800688, 0.9807852804091503618, 1.000000000000000000, 0.9807852804032304306, 1.000000000000000000, 0.9807852804032304306, 1.000000000000000000, 0.9807852804032304306, 1.000000000000000000, 0.9807852804032304306, 1.000000000000000000, 0.9807852804032304306, 1.000000000000000000, 0.9807852804032304306, 1.000000000000000000, 0.9807852803973104994, 1.000000000005919931 ) ) 
 REPRESENTATION_ITEM ( '' )  );
#739=CARTESIAN_POINT ( 'NONE',  ( 18.00000000043041126, 3.580422610670019434, -5.260981249819686845 ) ) ;
#757=CARTESIAN_POINT ( 'NONE',  ( 6.358192987158590270, -4.248408730893245000, 1.257393750180312741 ) ) ;
#763=CARTESIAN_POINT ( 'NONE',  ( -5.303300858261589035, 5.303300859536635770, 3.104325000180315541 ) ) ;
#765=CARTESIAN_POINT ( 'NONE',  ( 15.25966316918061416, -10.19618095414378622, 12.86254375018031304 ) ) ;
#770=CIRCLE ( 'NONE', #17360, 17.00000000000004619 ) ;
#776=ORIENTED_EDGE ( 'NONE', *, *, #3954, .F. ) ;
#777=CARTESIAN_POINT ( 'NONE',  ( -7.500000000000009770, -1.491842754878800248, -17.21833124991220743 ) ) ;
#781=CARTESIAN_POINT ( 'NONE',  ( 15.25966316918061239, -10.19618095414378445, -5.987456249819691045 ) ) ;
#783=EDGE_CURVE ( 'NONE', #100, #8208, #15180, .T. ) ;
#785=CARTESIAN_POINT ( 'NONE',  ( -10.32494394809439875, -4.276731812588566051, -7.658952749352573974 ) ) ;
#794=CARTESIAN_POINT ( 'NONE',  ( -3.580422610670018546, 18.00000000043041126, 11.23276875018031440 ) ) ;
#813=CARTESIAN_POINT ( 'NONE',  ( 14.79893867758297610, -1.779016607511492805E-09, 25.16529191884155026 ) ) ;
#821=CARTESIAN_POINT ( 'NONE',  ( -2.943691928843435779, -14.79893867722909917, -15.50201066848093312 ) ) ;
#832=CARTESIAN_POINT ( 'NONE',  ( -15.25966316918061416, 10.19618095414378445, 8.150043750180310909 ) ) ;
#840=CARTESIAN_POINT ( 'NONE',  ( -18.00000000043041481, -3.580422610670022987, 18.30151875018031049 ) ) ;
#842=CARTESIAN_POINT ( 'NONE',  ( -6.358192987158596488, 4.248408730893249441, -6.615206249819684636 ) ) ;
#845=CARTESIAN_POINT ( 'NONE',  ( -11.17563879731704723, 1.343452237168308679E-09, -14.19260975028680605 ) ) ;
#849=DIRECTION ( 'NONE',  ( -0.000000000000000000, -0.000000000000000000, -1.000000000000000000 ) ) ;
#850=CARTESIAN_POINT ( 'NONE',  ( 6.888301780572507305, -16.62983158603121936, -3.199262499819687022 ) ) ;
#865=( BOUNDED_CURVE ( )  B_SPLINE_CURVE ( 2, ( #12666, #20912, #11071, #7989, #4705, #3322, #4802, #6485, #17545, #11268, #15930, #11166, #17945, #34, #9684, #9572, #19426 ),
 .UNSPECIFIED., .F., .F. ) 
 B_SPLINE_CURVE_WITH_KNOTS ( ( 3, 2, 2, 2, 2, 2, 2, 2, 3 ),
 ( 0.5000000000038511416, 0.5125000000038510972, 0.5250000000038511638, 0.5375000000038511194, 0.5500000000038511860, 0.5625000000038511416, 0.5750000000038510972, 0.5875000000038511638, 0.6000000000038511194 ),
 .UNSPECIFIED. ) 
 CURVE ( )  GEOMETRIC_REPRESENTATION_ITEM ( )  RATIONAL_B_SPLINE_CURVE ( ( 0.9999999999940800688, 0.9807852804091503618, 1.000000000000000000, 0.9807852804032304306, 1.000000000000000000, 0.9807852804032304306, 1.000000000000000000, 0.9807852804032304306, 1.000000000000000000, 0.9807852804032304306, 1.000000000000000000, 0.9807852804032304306, 1.000000000000000000, 0.9807852804032304306, 1.000000000000000000, 0.9807852803973104994, 1.000000000005919931 ) ) 
 REPRESENTATION_ITEM ( '' )  );
#866=CARTESIAN_POINT ( 'NONE',  ( 7.499999999820660790, -1.491842756249031954, -8.756668749819690234 ) ) ;
#875=CARTESIAN_POINT ( 'NONE',  ( -10.19618095414378622, -15.25966316918061416, -3.631206249819686871 ) ) ;
#882=FACE_OUTER_BOUND ( 'NONE', #5657, .T. ) ;
#889=CARTESIAN_POINT ( 'NONE',  ( -10.19618095047497874, 15.25966317163202746, -0.6858937498196888694 ) ) ;
#894=CARTESIAN_POINT ( 'NONE',  ( 11.17563879758428769, 2.222972768810838939, -2.651921499352571931 ) ) ;
#904=CARTESIAN_POINT ( 'NONE',  ( -18.00000000000000000, 2.163826221265758884E-09, -9.678949999819687733 ) ) ;
#920=VECTOR ( 'NONE', #7736, 1000.000000000000000 ) ;
#921=CARTESIAN_POINT ( 'NONE',  ( -13.67243654778936168, -5.663308646854336992, 1.013729418841546437 ) ) ;
#928=DIRECTION ( 'NONE',  ( 1.000000000000000000, 0.000000000000000000, 0.000000000000000000 ) ) ;
#930=CARTESIAN_POINT ( 'NONE',  ( 15.25966316918061239, -10.19618095414378445, 3.437543750180311442 ) ) ;
#940=CARTESIAN_POINT ( 'NONE',  ( 7.500000000000007105, -1.491842755816071175, 6.933231250087794173 ) ) ;
#942=CARTESIAN_POINT ( 'NONE',  ( 7.500000000000001776, -1.491842755816069843, 0.6683312500877865991 ) ) ;
#943=CARTESIAN_POINT ( 'NONE',  ( 2.163825119083639120E-09, 17.99999999999999645, -18.65229999981968945 ) ) ;
#953=CARTESIAN_POINT ( 'NONE',  ( 12.72792206288791128, 12.72792205982780267, 12.70542500018031085 ) ) ;
#955=UNCERTAINTY_MEASURE_WITH_UNIT (LENGTH_MEASURE( 1.000000000000000082E-05 ), #18012, 'distance_accuracy_value', 'NONE');
#958=CARTESIAN_POINT ( 'NONE',  ( 5.303300859536635770, 5.303300858261589923, 5.460575000180316607 ) ) ;
#961=CARTESIAN_POINT ( 'NONE',  ( -7.902369976724391343, 7.902369978624323110, -13.01448475028680285 ) ) ;
#980=CARTESIAN_POINT ( 'NONE',  ( -4.248408729364575365, 6.358192988180014105, -2.866043749819687569 ) ) ;
#989=CARTESIAN_POINT ( 'NONE',  ( 12.72792205982779734, -12.72792206288791128, 3.732075000180311797 ) ) ;
#998=CARTESIAN_POINT ( 'NONE',  ( -1.491842756249033286, -7.499999999820668783, -18.98551874981968624 ) ) ;
#999=( BOUNDED_CURVE ( )  B_SPLINE_CURVE ( 2, ( #12435, #18795, #1317, #19000, #10838, #9457, #6275, #7763, #12653, #3095, #17308, #2783, #7977, #14234, #7547, #20899, #2998 ),
 .UNSPECIFIED., .F., .T. ) 
 B_SPLINE_CURVE_WITH_KNOTS ( ( 3, 2, 2, 2, 2, 2, 2, 2, 3 ),
 ( 0.5000000000038511416, 0.5125000000038510972, 0.5250000000038511638, 0.5375000000038511194, 0.5500000000038511860, 0.5625000000038511416, 0.5750000000038510972, 0.5875000000038511638, 0.6000000000038511194 ),
 .UNSPECIFIED. ) 
 CURVE ( )  GEOMETRIC_REPRESENTATION_ITEM ( )  RATIONAL_B_SPLINE_CURVE ( ( 0.9999999999940800688, 0.9807852804091503618, 1.000000000000000000, 0.9807852804032304306, 1.000000000000000000, 0.9807852804032304306, 1.000000000000000000, 0.9807852804032304306, 1.000000000000000000, 0.9807852804032304306, 1.000000000000000000, 0.9807852804032304306, 1.000000000000000000, 0.9807852804032304306, 1.000000000000000000, 0.9807852803973104994, 1.000000000005919931 ) ) 
 REPRESENTATION_ITEM ( '' )  );
#1008=CARTESIAN_POINT ( 'NONE',  ( -2.870125741905213079, 6.929096494179683319, -5.731612499819686235 ) ) ;
#1012=CARTESIAN_POINT ( 'NONE',  ( 12.72792206288790950, 12.72792205982780089, -6.144574999819688799 ) ) ;
#1025=CARTESIAN_POINT ( 'NONE',  ( 14.79893867793684059, 2.943691925285398359, 6.020760668841545815 ) ) ;
#1030=CARTESIAN_POINT ( 'NONE',  ( -2.163827323447877821E-09, -17.99999999999999645, 14.33520000018031126 ) ) ;
#1042=CARTESIAN_POINT ( 'NONE',  ( -15.25966317163202923, -10.19618095047497874, -12.46714374981969264 ) ) ;
#1043=ADVANCED_FACE ( 'NONE', ( #14443 ), #12752, .T. ) ;
#1052=CARTESIAN_POINT ( 'NONE',  ( 6.888301780572508193, -16.62983158603122291, -3.199262499819690575 ) ) ;
#1056=ORIENTED_EDGE ( 'NONE', *, *, #693, .T. ) ;
#1058=CARTESIAN_POINT ( 'NONE',  ( 14.79893867722909917, -2.943691928843437111, 10.41673933151907505 ) ) ;
#1063=CARTESIAN_POINT ( 'NONE',  ( -3.580422614997675002, -17.99999999956958163, -21.16566874981968738 ) ) ;
#1084=CARTESIAN_POINT ( 'NONE',  ( -4.276731812588563386, 10.32494394809438987, 15.84957774971319822 ) ) ;
#1088=LINE ( 'NONE', #18896, #7048 ) ;
#1094=CARTESIAN_POINT ( 'NONE',  ( 6.888301784570728614, 16.62983158437510056, -18.06323749981969229 ) ) ;
#1113=ORIENTED_EDGE ( 'NONE', *, *, #20190, .F. ) ;
#1123=CARTESIAN_POINT ( 'NONE',  ( -15.25966317163203279, -10.19618095047498052, -19.98754374981969306 ) ) ;
#1126=DIRECTION ( 'NONE',  ( -0.000000000000000000, -0.000000000000000000, 1.000000000000000000 ) ) ;
#1136=CARTESIAN_POINT ( 'NONE',  ( -5.663308646854337880, 13.67243654778935991, -6.055020581158455428 ) ) ;
#1141=CARTESIAN_POINT ( 'NONE',  ( 4.248408729364576253, -6.358192988180015881, -26.42854374981969556 ) ) ;
#1143=CARTESIAN_POINT ( 'NONE',  ( 2.163825119083639120E-09, 17.99999999999999645, 0.1977000001803091989 ) ) ;
#1154=CARTESIAN_POINT ( 'NONE',  ( 6.888301780572505528, -16.62983158603121581, -5.103862499819689980 ) ) ;
#1157=CARTESIAN_POINT ( 'NONE',  ( -6.358192988180021210, -4.248408729364580694, -8.382393749819687656 ) ) ;
#1165=CARTESIAN_POINT ( 'NONE',  ( -16.62983158437510411, 6.888301784570731279, 0.3351125001803089143 ) ) ;
#1169=CARTESIAN_POINT ( 'NONE',  ( -6.929096493489632635, 2.870125743571140919, -16.33473749981968837 ) ) ;
#1174=CARTESIAN_POINT ( 'NONE',  ( 13.67243654778934925, 5.663308646854335215, 18.95814558151907647 ) ) ;
#1178=LINE ( 'NONE', #7406, #18347 ) ;
#1187=DIRECTION ( 'NONE',  ( 1.000000000000000000, 0.000000000000000000, 0.000000000000000000 ) ) ;
#1188=ORIENTED_EDGE ( 'NONE', *, *, #8973, .T. ) ;
#1191=LINE ( 'NONE', #20570, #20758 ) ;
#1194=CARTESIAN_POINT ( 'NONE',  ( -2.222972768810836275, 11.17563879758427525, 16.14410899971320035 ) ) ;
#1195=ADVANCED_FACE ( 'NONE', ( #10170 ), #2017, .T. ) ;
#1203=CARTESIAN_POINT ( 'NONE',  ( -3.580422614997675002, -17.99999999956958163, -23.07026874981968945 ) ) ;
#1210=CYLINDRICAL_SURFACE ( 'NONE', #17638, 17.50000000000000355 ) ;
#1212=CARTESIAN_POINT ( 'NONE',  ( 7.500000000000002665, 1.491842754878804689, 0.07926875008778555554 ) ) ;
#1216=CARTESIAN_POINT ( 'NONE',  ( -12.50000000000000533, 0.000000000000000000, -43.00000000000000000 ) ) ;
#1233=CARTESIAN_POINT ( 'NONE',  ( -3.580422614997675002, -17.99999999956958163, -11.74066874981969200 ) ) ;
#1247=CARTESIAN_POINT ( 'NONE',  ( -5.663308650141539502, -13.67243654642775574, -9.589395581158459692 ) ) ;
#1254=CARTESIAN_POINT ( 'NONE',  ( 15.25966316918061239, -10.19618095414378445, 12.86254375018030949 ) ) ;
#1256=CARTESIAN_POINT ( 'NONE',  ( -5.303300858261584594, 5.303300859536631329, -22.01057499981969556 ) ) ;
#1267=CARTESIAN_POINT ( 'NONE',  ( -10.19618095047497874, 15.25966317163202746, -19.53589374981969229 ) ) ;
#1276=CARTESIAN_POINT ( 'NONE',  ( -6.888301784570739272, -16.62983158437509701, -2.021137499819691818 ) ) ;
#1280=ORIENTED_EDGE ( 'NONE', *, *, #6566, .T. ) ;
#1282=CARTESIAN_POINT ( 'NONE',  ( -5.663308646854335215, 13.67243654778934925, 7.176895581519076472 ) ) ;
#1284=ORIENTED_EDGE ( 'NONE', *, *, #1358, .T. ) ;
#1296=AXIS2_PLACEMENT_3D ( 'NONE', #9806, #16273, #1763 ) ;
#1305=CARTESIAN_POINT ( 'NONE',  ( 4.276731812588570492, -10.32494394809439697, -0.5902027493525709989 ) ) ;
#1306=CARTESIAN_POINT ( 'NONE',  ( 1.491842754445842134, -7.500000000179339210, -25.83948124981969130 ) ) ;
#1311=ORIENTED_EDGE ( 'NONE', *, *, #1323, .F. ) ;
#1312=CARTESIAN_POINT ( 'NONE',  ( 17.99999999956958163, -3.580422614997676334, -6.576518749819688203 ) ) ;
#1316=VERTEX_POINT ( 'NONE', #13884 ) ;
#1317=CARTESIAN_POINT ( 'NONE',  ( -6.929096494179678878, -2.870125741905209971, -4.927762499819690944 ) ) ;
#1323=EDGE_CURVE ( 'NONE', #20518, #9271, #20328, .T. ) ;
#1327=DIRECTION ( 'NONE',  ( 0.000000000000000000, 0.000000000000000000, 1.000000000000000000 ) ) ;
#1332=VERTEX_POINT ( 'NONE', #9114 ) ;
#1336=CARTESIAN_POINT ( 'NONE',  ( 17.99999999956958163, -3.580422614997676334, -4.671918749819689687 ) ) ;
#1350=CARTESIAN_POINT ( 'NONE',  ( -14.79893867722910628, 2.943691928843437111, 1.897323168841544394 ) ) ;
#1352=CARTESIAN_POINT ( 'NONE',  ( -4.248408730893246776, -6.358192987158592047, -15.23635624981969627 ) ) ;
#1354=VERTEX_POINT ( 'NONE', #2547 ) ;
#1356=DIRECTION ( 'NONE',  ( -0.000000000000000000, -0.000000000000000000, 1.000000000000000000 ) ) ;
#1358=EDGE_CURVE ( 'NONE', #10315, #9271, #7170, .T. ) ;
#1360=VECTOR ( 'NONE', #271, 1000.000000000000000 ) ;
#1367=CARTESIAN_POINT ( 'NONE',  ( -3.580422610670017658, 18.00000000043040771, -9.521831249819690868 ) ) ;
#1375=CARTESIAN_POINT ( 'NONE',  ( 3.580422614997669228, 17.99999999956958874, 11.82183125018031156 ) ) ;
#1376=CARTESIAN_POINT ( 'NONE',  ( 7.500000000000007994, -9.015933403756345817E-10, -21.63629999981969121 ) ) ;
#1379=CARTESIAN_POINT ( 'NONE',  ( 8.382925368423265411, -12.54593441764187034, 11.59486433151907470 ) ) ;
#1381=AXIS2_PLACEMENT_3D ( 'NONE', #10449, #12141, #244 ) ;
#1384=CARTESIAN_POINT ( 'NONE',  ( 2.163825119083639534E-09, 18.00000000000000000, -16.74769999981968738 ) ) ;
#1398=EDGE_CURVE ( 'NONE', #10636, #1438, #1178, .T. ) ;
#1400=CARTESIAN_POINT ( 'NONE',  ( -6.330490856366295382, 9.474249098604511587, -15.02223399935257042 ) ) ;
#1401=CARTESIAN_POINT ( 'NONE',  ( -5.303300858261583706, 5.303300859536630441, -22.01057499981969201 ) ) ;
#1408=CARTESIAN_POINT ( 'NONE',  ( 2.163825119083639534E-09, 18.00000000000000000, -9.227299999819686960 ) ) ;
#1416=LINE ( 'NONE', #7866, #7682 ) ;
#1423=ADVANCED_FACE ( 'NONE', ( #7302 ), #20234, .T. ) ;
#1433=VERTEX_POINT ( 'NONE', #12401 ) ;
#1438=VERTEX_POINT ( 'NONE', #18872 ) ;
#1450=CARTESIAN_POINT ( 'NONE',  ( -1.343452921478824119E-09, -11.17563879731705789, 18.84885975064742425 ) ) ;
#1454=CARTESIAN_POINT ( 'NONE',  ( 2.870125741905212635, -6.929096494179677101, -16.70901249981969272 ) ) ;
#1455=FACE_BOUND ( 'NONE', #20340, .T. ) ;
#1460=CARTESIAN_POINT ( 'NONE',  ( -6.929096493489627306, 2.870125743571138699, -22.59963749981969627 ) ) ;
#1463=EDGE_LOOP ( 'NONE', ( #3145, #5922, #2992, #2618 ) ) ;
#1473=MECHANICAL_DESIGN_GEOMETRIC_PRESENTATION_REPRESENTATION('',(#5158),#7492);
#1477=CARTESIAN_POINT ( 'NONE',  ( -7.500000000000000000, 0.000000000000000000, 40.00000000000000000 ) ) ;
#1479=DIRECTION ( 'NONE',  ( -0.000000000000000000, -0.000000000000000000, 1.000000000000000000 ) ) ;
#1483=CARTESIAN_POINT ( 'NONE',  ( -10.19618095047498230, 15.25966317163203279, -17.63129374981969377 ) ) ;
#1485=CARTESIAN_POINT ( 'NONE',  ( 7.499999999820668783, -1.491842756249033508, -11.91676874981968659 ) ) ;
#1489=CARTESIAN_POINT ( 'NONE',  ( 10.46442989202483531, -10.46442989454075168, -7.549666918480926192 ) ) ;
#1494=DIRECTION ( 'NONE',  ( -0.4999999999999918954, 0.8660254037844433705, 0.000000000000000000 ) ) ;
#1496=CIRCLE ( 'NONE', #468, 2.650000000000000355 ) ;
#1502=CARTESIAN_POINT ( 'NONE',  ( -17.99999999956958163, 3.580422614997673669, 16.98598125018031268 ) ) ;
#1506=VECTOR ( 'NONE', #14655, 1000.000000000000000 ) ;
#1512=CARTESIAN_POINT ( 'NONE',  ( -4.276731812588566939, 10.32494394809439875, -5.302702749352572020 ) ) ;
#1513=CARTESIAN_POINT ( 'NONE',  ( -6.358192988180014993, -4.248408729364575365, -24.07229374981969627 ) ) ;
#1516=DIRECTION ( 'NONE',  ( -0.4999999999999918954, 0.8660254037844433705, 0.000000000000000000 ) ) ;
#1521=CARTESIAN_POINT ( 'NONE',  ( 10.19618095414378800, 15.25966316918061416, -17.76870624981969016 ) ) ;
#1527=DIRECTION ( 'NONE',  ( -1.000000000000000000, 0.000000000000000000, 0.000000000000000000 ) ) ;
#1528=CARTESIAN_POINT ( 'NONE',  ( -6.929096493489627306, 2.870125743571138699, -3.749637499819692632 ) ) ;
#1557=CARTESIAN_POINT ( 'NONE',  ( -12.54593441562641054, 8.382925371439629458, -16.36361433115845898 ) ) ;
#1563=( BOUNDED_CURVE ( )  B_SPLINE_CURVE ( 2, ( #10433, #16893, #2370, #8822, #9368, #5969, #19123, #7771, #16041, #12341, #6283, #17539, #9568, #17217, #11063, #14149, #12446 ),
 .UNSPECIFIED., .F., .T. ) 
 B_SPLINE_CURVE_WITH_KNOTS ( ( 3, 2, 2, 2, 2, 2, 2, 2, 3 ),
 ( 0.1000000000038511888, 0.1125000000038511860, 0.1250000000038511694, 0.1375000000038511805, 0.1500000000038511638, 0.1625000000038511749, 0.1750000000038511583, 0.1875000000038511694, 0.2000000000038511805 ),
 .UNSPECIFIED. ) 
 CURVE ( )  GEOMETRIC_REPRESENTATION_ITEM ( )  RATIONAL_B_SPLINE_CURVE ( ( 0.9999999999940800688, 0.9807852804091503618, 1.000000000000000000, 0.9807852804032304306, 1.000000000000000000, 0.9807852804032304306, 1.000000000000000000, 0.9807852804032304306, 1.000000000000000000, 0.9807852804032304306, 1.000000000000000000, 0.9807852804032304306, 1.000000000000000000, 0.9807852804032304306, 1.000000000000000000, 0.9807852803973104994, 1.000000000005919931 ) ) 
 REPRESENTATION_ITEM ( '' )  );
#1565=CARTESIAN_POINT ( 'NONE',  ( 15.25966317163202746, 10.19618095047498407, 22.42495625018031191 ) ) ;
#1583=CARTESIAN_POINT ( 'NONE',  ( 16.62983158437509701, -6.888301784570740161, -13.80238749981969271 ) ) ;
#1591=CARTESIAN_POINT ( 'NONE',  ( -1.779019326032424095E-09, -14.79893867758296544, 3.053458081519074163 ) ) ;
#1596=CARTESIAN_POINT ( 'NONE',  ( -2.870125741905213079, 6.929096494179683319, 22.54338750018031590 ) ) ;
#1615=CARTESIAN_POINT ( 'NONE',  ( -6.929096493489632635, 2.870125743571140919, 11.94026250018031554 ) ) ;
#1616=CARTESIAN_POINT ( 'NONE',  ( 10.32494394706615637, -4.276731815070946574, 0.5339527497131985045 ) ) ;
#1625=VERTEX_POINT ( 'NONE', #11630 ) ;
#1626=CARTESIAN_POINT ( 'NONE',  ( 18.00000000043041126, 3.580422610670019434, 23.01401875018031262 ) ) ;
#1637=ORIENTED_EDGE ( 'NONE', *, *, #18433, .F. ) ;
#1642=STYLED_ITEM ( 'NONE', ( #16647 ), #7446 ) ;
#1645=CARTESIAN_POINT ( 'NONE',  ( 9.015937996181834148E-10, 7.500000000000000888, 7.442550000180311542 ) ) ;
#1651=LINE ( 'NONE', #3327, #12576 ) ;
#1652=CARTESIAN_POINT ( 'NONE',  ( -3.580422610670018546, 18.00000000043041126, 18.75316875018031482 ) ) ;
#1655=FACE_BOUND ( 'NONE', #7489, .T. ) ;
#1661=CARTESIAN_POINT ( 'NONE',  ( -5.663308650141539502, -13.67243654642775574, -19.01439558115845685 ) ) ;
#1668=CARTESIAN_POINT ( 'NONE',  ( 6.929096493489625530, -2.870125743571142252, -27.31213749981969485 ) ) ;
#1669=CARTESIAN_POINT ( 'NONE',  ( -17.99999999956958519, 3.580422614997674113, 18.89058125018031475 ) ) ;
#1674=ORIENTED_EDGE ( 'NONE', *, *, #8973, .F. ) ;
#1677=CARTESIAN_POINT ( 'NONE',  ( 4.248408730893249441, 6.358192987158596488, -4.258956249819687123 ) ) ;
#1683=CARTESIAN_POINT ( 'NONE',  ( -18.00000000000000355, 2.163826221265759298E-09, -9.678949999819691286 ) ) ;
#1685=CARTESIAN_POINT ( 'NONE',  ( -17.50000000000000355, 0.000000000000000000, -43.00000000000000000 ) ) ;
#1687=CARTESIAN_POINT ( 'NONE',  ( 8.382925371439627682, 12.54593441562639988, -0.7754481684809252373 ) ) ;
#1707=CARTESIAN_POINT ( 'NONE',  ( -7.499999999820669672, 1.491842756249032620, 21.07073125018031945 ) ) ;
#1708=CARTESIAN_POINT ( 'NONE',  ( 1.343451552857795099E-09, 11.17563879731704723, -2.411359750286803827 ) ) ;
#1715=CARTESIAN_POINT ( 'NONE',  ( -10.19618095414378622, -15.25966316918061416, 7.698393750180313688 ) ) ;
#1753=CARTESIAN_POINT ( 'NONE',  ( 10.46442989454075700, 10.46442989202484419, -13.71283308115846111 ) ) ;
#1763=DIRECTION ( 'NONE',  ( 1.000000000000000000, 0.000000000000000000, 0.000000000000000000 ) ) ;
#1765=EDGE_LOOP ( 'NONE', ( #13180, #11942, #776, #17211 ) ) ;
#1767=EDGE_LOOP ( 'NONE', ( #5370, #1113 ) ) ;
#1770=CARTESIAN_POINT ( 'NONE',  ( 0.000000000000000000, 0.000000000000000000, -43.00000000000000000 ) ) ;
#1778=CARTESIAN_POINT ( 'NONE',  ( 12.72792205982779912, -12.72792206288791483, -3.788324999819691286 ) ) ;
#1782=CARTESIAN_POINT ( 'NONE',  ( 2.943691925285397470, -14.79893867793683349, -6.666073168480925126 ) ) ;
#1788=CARTESIAN_POINT ( 'NONE',  ( 4.248408730893249441, 6.358192987158596488, 24.01604375018031945 ) ) ;
#1799=( BOUNDED_CURVE ( )  B_SPLINE_CURVE ( 2, ( #5374, #3882, #18309, #3775, #13232, #10257, #10052, #19790, #16516, #16719, #2000, #19989, #5272, #8658, #5472, #940, #2407 ),
 .UNSPECIFIED., .F., .T. ) 
 B_SPLINE_CURVE_WITH_KNOTS ( ( 3, 2, 2, 2, 2, 2, 2, 2, 3 ),
 ( 0.3000000000038511860, 0.3125000000038511971, 0.3250000000038512082, 0.3375000000038512193, 0.3500000000038511749, 0.3625000000038511860, 0.3750000000038511971, 0.3875000000038512082, 0.4000000000038512193 ),
 .UNSPECIFIED. ) 
 CURVE ( )  GEOMETRIC_REPRESENTATION_ITEM ( )  RATIONAL_B_SPLINE_CURVE ( ( 0.9999999999940800688, 0.9807852804091503618, 1.000000000000000000, 0.9807852804032304306, 1.000000000000000000, 0.9807852804032304306, 1.000000000000000000, 0.9807852804032304306, 1.000000000000000000, 0.9807852804032304306, 1.000000000000000000, 0.9807852804032304306, 1.000000000000000000, 0.9807852804032304306, 1.000000000000000000, 0.9807852803973104994, 1.000000000005919931 ) ) 
 REPRESENTATION_ITEM ( '' )  );
#1800=ORIENTED_EDGE ( 'NONE', *, *, #5337, .F. ) ;
#1806=EDGE_CURVE ( 'NONE', #3529, #15394, #770, .T. ) ;
#1809=CARTESIAN_POINT ( 'NONE',  ( -6.929096493489632635, 2.870125743571140919, 21.36526250018031803 ) ) ;
#1810=CARTESIAN_POINT ( 'NONE',  ( -11.17563879758427525, -2.222972768810838051, -5.062141000286804804 ) ) ;
#1816=CARTESIAN_POINT ( 'NONE',  ( 16.62983158603122291, 6.888301780572502864, 13.29448750018031511 ) ) ;
#1825=VERTEX_POINT ( 'NONE', #6298 ) ;
#1832=EDGE_CURVE ( 'NONE', #1886, #19935, #4185, .T. ) ;
#1836=CARTESIAN_POINT ( 'NONE',  ( 5.303300858261582817, -5.303300859536631329, 10.97692500018031225 ) ) ;
#1856=CARTESIAN_POINT ( 'NONE',  ( -10.32494394706616703, 4.276731815070943910, 2.944172250647428601 ) ) ;
#1864=CARTESIAN_POINT ( 'NONE',  ( 6.888301780572507305, -16.62983158603121936, 15.65073750018031440 ) ) ;
#1866=CARTESIAN_POINT ( 'NONE',  ( 12.92641286132474931, -1.553915700095510638E-09, -21.87673848677710708 ) ) ;
#1871=DIRECTION ( 'NONE',  ( -0.5000000000000037748, -0.8660254037844364872, 0.000000000000000000 ) ) ;
#1878=CARTESIAN_POINT ( 'NONE',  ( -16.62983158437510411, 6.888301784570731279, -9.089887499819690575 ) ) ;
#1881=CARTESIAN_POINT ( 'NONE',  ( -2.943691928843435779, -14.79893867722909917, 3.347989331519075851 ) ) ;
#1886=VERTEX_POINT ( 'NONE', #7576 ) ;
#1894=CARTESIAN_POINT ( 'NONE',  ( 12.72792206288790773, 12.72792205982779912, 20.22582500018031482 ) ) ;
#1905=CARTESIAN_POINT ( 'NONE',  ( -1.491842754445842800, 7.500000000179346316, 13.41291875018031554 ) ) ;
#1906=CARTESIAN_POINT ( 'NONE',  ( -7.902369978624323110, -7.902369976724391343, -5.945734750286804093 ) ) ;
#1909=CYLINDRICAL_SURFACE ( 'NONE', #17185, 7.500000000000000000 ) ;
#1911=AXIS2_PLACEMENT_3D ( 'NONE', #1216, #2688, #12441 ) ;
#1915=CARTESIAN_POINT ( 'NONE',  ( -16.62983158603122291, -6.888301780572501087, 18.00698750018031546 ) ) ;
#1933=CARTESIAN_POINT ( 'NONE',  ( 4.248408729364575365, -6.358192988180014993, 11.27145625018031438 ) ) ;
#1939=ORIENTED_EDGE ( 'NONE', *, *, #522, .T. ) ;
#1942=CARTESIAN_POINT ( 'NONE',  ( 10.19618095414378800, 15.25966316918061416, 19.93129375018031268 ) ) ;
#1956=CARTESIAN_POINT ( 'NONE',  ( -5.303300858261584594, 5.303300859536631329, -12.58557499981969130 ) ) ;
#1960=CARTESIAN_POINT ( 'NONE',  ( -7.902369976724401113, 7.902369978624329327, 12.95823475064742780 ) ) ;
#1977=CARTESIAN_POINT ( 'NONE',  ( 1.491842754445843688, -7.500000000179346316, -19.57458124981968695 ) ) ;
#1979=ADVANCED_FACE ( 'NONE', ( #9791 ), #9994, .F. ) ;
#1984=CARTESIAN_POINT ( 'NONE',  ( 5.663308646854342321, -13.67243654778935635, 8.082479418841543861 ) ) ;
#1986=EDGE_CURVE ( 'NONE', #20036, #6207, #14480, .T. ) ;
#1992=CARTESIAN_POINT ( 'NONE',  ( 10.19618095414378622, 15.25966316918061239, 19.93129375018031268 ) ) ;
#2000=CARTESIAN_POINT ( 'NONE',  ( 2.870125741905214412, -6.929096494179682431, 8.405887500180314831 ) ) ;
#2003=CARTESIAN_POINT ( 'NONE',  ( 10.19618095414378622, 15.25966316918061239, 1.081293750180310820 ) ) ;
#2009=CARTESIAN_POINT ( 'NONE',  ( -10.19618095414378800, -15.25966316918061771, 17.12339375018030907 ) ) ;
#2010=UNCERTAINTY_MEASURE_WITH_UNIT (LENGTH_MEASURE( 1.000000000000000082E-05 ), #11516, 'distance_accuracy_value', 'NONE');
#2012=CARTESIAN_POINT ( 'NONE',  ( 9.015937996181842420E-10, 7.500000000000007994, 23.13245000018031661 ) ) ;
#2013=CARTESIAN_POINT ( 'NONE',  ( -11.17563879704981922, 2.222972771497742972, 4.951921499713198394 ) ) ;
#2017=CYLINDRICAL_SURFACE ( 'NONE', #19701, 17.50000000000000355 ) ;
#2018=CARTESIAN_POINT ( 'NONE',  ( -15.25966316918061771, 10.19618095414378622, 10.05464375018031475 ) ) ;
#2028=DIRECTION ( 'NONE',  ( -0.000000000000000000, -0.000000000000000000, -1.000000000000000000 ) ) ;
#2029=ADVANCED_FACE ( 'NONE', ( #4813, #3225, #16163, #1655, #14574 ), #43, .F. ) ;
#2032=CARTESIAN_POINT ( 'NONE',  ( 7.500000000179339210, 1.491842754445841690, 18.92926875018031652 ) ) ;
#2055=CARTESIAN_POINT ( 'NONE',  ( -6.330490858644140850, -9.474249097082498849, 10.30745350064742993 ) ) ;
#2059=DIRECTION ( 'NONE',  ( 0.000000000000000000, 0.000000000000000000, -1.000000000000000000 ) ) ;
#2060=EDGE_LOOP ( 'NONE', ( #7515, #17915, #1939, #1280 ) ) ;
#2063=CARTESIAN_POINT ( 'NONE',  ( 10.19618095414378800, 15.25966316918061416, 2.985893750180313777 ) ) ;
#2067=VECTOR ( 'NONE', #1356, 1000.000000000000000 ) ;
#2072=FACE_OUTER_BOUND ( 'NONE', #13430, .T. ) ;
#2079=CARTESIAN_POINT ( 'NONE',  ( 10.46442989202484064, -10.46442989454075878, 16.91841691884155452 ) ) ;
#2087=CARTESIAN_POINT ( 'NONE',  ( -1.779019326032424095E-09, -14.79893867758296544, -25.22154191848092708 ) ) ;
#2089=EDGE_CURVE ( 'NONE', #13866, #9669, #2359, .T. ) ;
#2100=CARTESIAN_POINT ( 'NONE',  ( 3.580422610670019878, -18.00000000043040771, 4.615668750180310198 ) ) ;
#2112=CARTESIAN_POINT ( 'NONE',  ( -2.870125743571144028, -6.929096493489630859, -9.265987499819688722 ) ) ;
#2114=CARTESIAN_POINT ( 'NONE',  ( -1.343452921478823292E-09, -11.17563879731704723, -7.123859750286805514 ) ) ;
#2122=CARTESIAN_POINT ( 'NONE',  ( 10.19618095047497874, -15.25966317163203279, -3.493793749819687822 ) ) ;
#2125=ORIENTED_EDGE ( 'NONE', *, *, #3539, .F. ) ;
#2140=CARTESIAN_POINT ( 'NONE',  ( 2.870125741905211747, -6.929096494179675325, 2.140987500180310921 ) ) ;
#2150=CARTESIAN_POINT ( 'NONE',  ( -3.580422614997675002, -17.99999999956958163, -4.220268749819688914 ) ) ;
#2158=ORIENTED_EDGE ( 'NONE', *, *, #783, .T. ) ;
#2161=CARTESIAN_POINT ( 'NONE',  ( -6.929096493489627306, 2.870125743571138699, -13.17463749981969201 ) ) ;
#2162=CARTESIAN_POINT ( 'NONE',  ( 12.72792205982779379, -12.72792206288790950, -5.692924999819690690 ) ) ;
#2167=CARTESIAN_POINT ( 'NONE',  ( 6.330490858644141738, 9.474249097082498849, 15.01995350064743029 ) ) ;
#2175=EDGE_CURVE ( 'NONE', #9271, #10315, #13645, .T. ) ;
#2176=CARTESIAN_POINT ( 'NONE',  ( -10.19618095047498052, 15.25966317163203101, 10.64370625018031369 ) ) ;
#2178=CARTESIAN_POINT ( 'NONE',  ( -7.500000000000000000, 0.000000000000000000, 40.00000000000000000 ) ) ;
#2186=CARTESIAN_POINT ( 'NONE',  ( -10.46442989202484242, 10.46442989454075700, 12.20591691884154528 ) ) ;
#2190=ORIENTED_EDGE ( 'NONE', *, *, #14380, .F. ) ;
#2192=CARTESIAN_POINT ( 'NONE',  ( -14.79893867722910095, 2.943691928843434891, -22.57076066848093276 ) ) ;
#2197=CARTESIAN_POINT ( 'NONE',  ( -7.500000000000002665, -4.022542205827308438E-17, 14.51130000000230602 ) ) ;
#2204=CARTESIAN_POINT ( 'NONE',  ( -16.62983158437509701, 6.888301784570728614, 7.855512500180310553 ) ) ;
#2212=CARTESIAN_POINT ( 'NONE',  ( -7.500000000000007105, 1.491842755816076505, -16.62926874991220672 ) ) ;
#2215=FACE_OUTER_BOUND ( 'NONE', #8943, .T. ) ;
#2216=CARTESIAN_POINT ( 'NONE',  ( -6.929096494179684207, -2.870125741905212635, 1.337137500180316074 ) ) ;
#2217=CIRCLE ( 'NONE', #14082, 7.500000000000000000 ) ;
#2218=CARTESIAN_POINT ( 'NONE',  ( -4.276731812588563386, 10.32494394809438987, -21.85042225028680818 ) ) ;
#2224=CARTESIAN_POINT ( 'NONE',  ( 12.72792206288790950, 12.72792205982780089, 3.280425000180314132 ) ) ;
#2242=CARTESIAN_POINT ( 'NONE',  ( 7.500000000000000888, -9.015933403756337545E-10, -9.051199999819688813 ) ) ;
#2255=CARTESIAN_POINT ( 'NONE',  ( 10.19618095047497874, -15.25966317163203279, -5.398393749819686782 ) ) ;
#2267=CARTESIAN_POINT ( 'NONE',  ( -9.850000000000006750, 0.000000000000000000, -43.00000000000000000 ) ) ;
#2268=CARTESIAN_POINT ( 'NONE',  ( 2.163825119083639120E-09, 17.99999999999999645, -9.227299999819690512 ) ) ;
#2271=CARTESIAN_POINT ( 'NONE',  ( -7.500000000000004441, 9.706494107352906755E-15, -4.338699999997692736 ) ) ;
#2272=CARTESIAN_POINT ( 'NONE',  ( 11.17563879758428769, 2.222972768810838939, 16.19807850064743349 ) ) ;
#2280=CARTESIAN_POINT ( 'NONE',  ( -3.580422614997675002, -17.99999999956958163, -2.315668749819689065 ) ) ;
#2287=CARTESIAN_POINT ( 'NONE',  ( -2.870125741905213079, 6.929096494179683319, 13.11838750018031519 ) ) ;
#2293=CYLINDRICAL_SURFACE ( 'NONE', #8724, 7.500000000000000000 ) ;
#2299=CARTESIAN_POINT ( 'NONE',  ( -5.663308650141539502, -13.67243654642775574, 9.260604418841545282 ) ) ;
#2303=CARTESIAN_POINT ( 'NONE',  ( 6.249999999999902300, -10.82531754730554496, 40.00000000000000000 ) ) ;
#2304=CARTESIAN_POINT ( 'NONE',  ( 5.663308650141530620, 13.67243654642775041, -19.91997941848093490 ) ) ;
#2308=CARTESIAN_POINT ( 'NONE',  ( 1.491842756249029289, 7.499999999820664343, 17.16208125018031083 ) ) ;
#2313=CARTESIAN_POINT ( 'NONE',  ( -3.580422610670017658, 18.00000000043040771, -0.09683124981969132294 ) ) ;
#2319=FACE_OUTER_BOUND ( 'NONE', #14479, .T. ) ;
#2321=CARTESIAN_POINT ( 'NONE',  ( -6.358192987158596488, 4.248408730893249441, 2.809793750180315186 ) ) ;
#2324=CARTESIAN_POINT ( 'NONE',  ( -10.32494394706615815, 4.276731815070940357, -13.60354725028680356 ) ) ;
#2328=CARTESIAN_POINT ( 'NONE',  ( -17.99999999956958519, 3.580422614997674113, 0.04058125018031183417 ) ) ;
#2346=CARTESIAN_POINT ( 'NONE',  ( -7.500000000000000888, 9.015942588607330751E-10, -13.76369999981968917 ) ) ;
#2353=ORIENTED_EDGE ( 'NONE', *, *, #15535, .T. ) ;
#2355=CARTESIAN_POINT ( 'NONE',  ( -10.19618095047498052, 15.25966317163203101, -0.6858937498196854277 ) ) ;
#2359=LINE ( 'NONE', #15186, #4858 ) ;
#2360=EDGE_LOOP ( 'NONE', ( #18552, #13909 ) ) ;
#2366=CARTESIAN_POINT ( 'NONE',  ( 9.015937996181835182E-10, 7.500000000000002665, -11.40744999981969166 ) ) ;
#2367=CARTESIAN_POINT ( 'NONE',  ( -12.72792206288790950, -12.72792205982779556, -3.336674999819690068 ) ) ;
#2370=CARTESIAN_POINT ( 'NONE',  ( -6.929096494179678878, -2.870125741905209971, 13.92223750018030870 ) ) ;
#2371=CARTESIAN_POINT ( 'NONE',  ( 10.32494394809439875, 4.276731812588567827, -2.946452749352572287 ) ) ;
#2379=CARTESIAN_POINT ( 'NONE',  ( -10.19618095414378622, -15.25966316918061416, 7.698393750180313688 ) ) ;
#2389=VECTOR ( 'NONE', #8302, 1000.000000000000000 ) ;
#2395=CARTESIAN_POINT ( 'NONE',  ( 8.382925371439633011, 12.54593441562640876, 14.26763566884154777 ) ) ;
#2400=CARTESIAN_POINT ( 'NONE',  ( -2.943691928843435779, -14.79893867722909917, -24.92701066848092850 ) ) ;
#2407=CARTESIAN_POINT ( 'NONE',  ( 7.500000000000007105, 4.207617034055637320E-15, 6.638700000002313750 ) ) ;
#2410=CARTESIAN_POINT ( 'NONE',  ( -2.163827323447877821E-09, -17.99999999999999645, 4.910200000180310553 ) ) ;
#2412=ORIENTED_EDGE ( 'NONE', *, *, #20065, .T. ) ;
#2419=CARTESIAN_POINT ( 'NONE',  ( -10.19618095047498230, 15.25966317163203279, 20.06870625018031262 ) ) ;
#2421=CARTESIAN_POINT ( 'NONE',  ( 2.870125743571140475, 6.929096493489632635, -4.553487499819687478 ) ) ;
#2423=CARTESIAN_POINT ( 'NONE',  ( 4.248408729364579806, -6.358192988180021210, 17.53635625018031519 ) ) ;
#2424=CARTESIAN_POINT ( 'NONE',  ( -10.32494394706615815, 4.276731815070940357, -23.02854725028680960 ) ) ;
#2429=CARTESIAN_POINT ( 'NONE',  ( -3.580422614997675002, -17.99999999956958163, -2.315668749819689065 ) ) ;
#2448=CARTESIAN_POINT ( 'NONE',  ( 1.491842756249028845, 7.499999999820661678, -1.687918749819689035 ) ) ;
#2457=CARTESIAN_POINT ( 'NONE',  ( -12.72792205982779912, 12.72792206288790950, -0.9804249998196858940 ) ) ;
#2473=( BOUNDED_CURVE ( )  B_SPLINE_CURVE ( 2, ( #20035, #8712, #16766, #10417, #13587, #5321, #344, #6797, #16877, #5519, #19841, #20142, #763, #3518, #7107, #11998, #5632 ),
 .UNSPECIFIED., .F., .F. ) 
 B_SPLINE_CURVE_WITH_KNOTS ( ( 3, 2, 2, 2, 2, 2, 2, 2, 3 ),
 ( 0.4000000000038512193, 0.4125000000038511749, 0.4250000000038511860, 0.4375000000038511971, 0.4500000000038512082, 0.4625000000038511638, 0.4750000000038511194, 0.4875000000038511305, 0.5000000000038511416 ),
 .UNSPECIFIED. ) 
 CURVE ( )  GEOMETRIC_REPRESENTATION_ITEM ( )  RATIONAL_B_SPLINE_CURVE ( ( 0.9999999999940800688, 0.9807852804091503618, 1.000000000000000000, 0.9807852804032304306, 1.000000000000000000, 0.9807852804032304306, 1.000000000000000000, 0.9807852804032304306, 1.000000000000000000, 0.9807852804032304306, 1.000000000000000000, 0.9807852804032304306, 1.000000000000000000, 0.9807852804032304306, 1.000000000000000000, 0.9807852803973104994, 1.000000000005919931 ) ) 
 REPRESENTATION_ITEM ( '' )  );
#2476=CARTESIAN_POINT ( 'NONE',  ( 18.00000000043040771, 3.580422610670018546, -7.165581249819690690 ) ) ;
#2480=CARTESIAN_POINT ( 'NONE',  ( -2.222972771497745192, -11.17563879704982632, -9.131608999352575751 ) ) ;
#2483=ORIENTED_EDGE ( 'NONE', *, *, #20515, .T. ) ;
#2490=CARTESIAN_POINT ( 'NONE',  ( -6.888301784570738384, -16.62983158437509346, 7.403862500180314221 ) ) ;
#2499=CARTESIAN_POINT ( 'NONE',  ( -7.500000000000007105, -3.289131931996631318E-15, 11.35120000000231677 ) ) ;
#2506=EDGE_CURVE ( 'NONE', #15181, #11708, #9611, .T. ) ;
#2510=CARTESIAN_POINT ( 'NONE',  ( 1.779017513685136568E-09, 14.79893867758297610, 3.959041918841544216 ) ) ;
#2517=CARTESIAN_POINT ( 'NONE',  ( -3.580422614997674557, -17.99999999956957808, 5.204731250180311797 ) ) ;
#2529=CARTESIAN_POINT ( 'NONE',  ( -12.72792206288790950, -12.72792205982779556, -12.76167499981969300 ) ) ;
#2536=CARTESIAN_POINT ( 'NONE',  ( -7.500000000000009770, 9.706494107251932559E-15, -16.92379999999768359 ) ) ;
#2537=CARTESIAN_POINT ( 'NONE',  ( -6.888301780572502864, 16.62983158603122646, 1.513237500180307560 ) ) ;
#2538=EDGE_CURVE ( 'NONE', #16575, #17634, #20790, .T. ) ;
#2540=CARTESIAN_POINT ( 'NONE',  ( -7.500000000179346316, -1.491842754445844355, -7.793331249819686057 ) ) ;
#2542=CARTESIAN_POINT ( 'NONE',  ( -6.929096494179684207, -2.870125741905212635, 20.18713750018031305 ) ) ;
#2543=CARTESIAN_POINT ( 'NONE',  ( 6.330490858644138186, 9.474249097082495297, -10.95276600028680569 ) ) ;
#2547=CARTESIAN_POINT ( 'NONE',  ( 7.500000000000007105, -2.290195989506637665E-15, 16.06370000000231357 ) ) ;
#2548=CARTESIAN_POINT ( 'NONE',  ( -10.19618095047498052, 15.25966317163203101, 1.218706250180314088 ) ) ;
#2564=CARTESIAN_POINT ( 'NONE',  ( 9.015937996181834148E-10, 7.500000000000000888, -11.40744999981968810 ) ) ;
#2573=CARTESIAN_POINT ( 'NONE',  ( -6.888301780572501976, 16.62983158603122291, -0.3913624998196884031 ) ) ;
#2575=ORIENTED_EDGE ( 'NONE', *, *, #9724, .F. ) ;
#2583=CARTESIAN_POINT ( 'NONE',  ( 2.870125741905214412, -6.929096494179682431, -19.86911249981968552 ) ) ;
#2585=CARTESIAN_POINT ( 'NONE',  ( 15.25966316918061239, -10.19618095414378445, -24.83745624981969513 ) ) ;
#2588=AXIS2_PLACEMENT_3D ( 'NONE', #13797, #12303, #20341 ) ;
#2596=CARTESIAN_POINT ( 'NONE',  ( -7.500000000000007105, 1.491842755816076505, -7.204268749912206893 ) ) ;
#2601=CARTESIAN_POINT ( 'NONE',  ( 17.99999999956958163, -3.580422614997676334, -14.09691874981968951 ) ) ;
#2607=AXIS2_PLACEMENT_3D ( 'NONE', #17816, #13039, #3379 ) ;
#2611=EDGE_LOOP ( 'NONE', ( #8358, #15861, #18578, #20131 ) ) ;
#2616=CARTESIAN_POINT ( 'NONE',  ( 13.67243654642775574, -5.663308650141541278, 6.904354418841546881 ) ) ;
#2618=ORIENTED_EDGE ( 'NONE', *, *, #522, .F. ) ;
#2619=VECTOR ( 'NONE', #13322, 1000.000000000000000 ) ;
#2625=CARTESIAN_POINT ( 'NONE',  ( 17.99999999956957808, -3.580422614997675446, 12.27348125018031055 ) ) ;
#2638=CARTESIAN_POINT ( 'NONE',  ( 16.62983158603121936, 6.888301780572501976, -7.460112499819690157 ) ) ;
#2648=CARTESIAN_POINT ( 'NONE',  ( 15.25966316918061771, -10.19618095414378800, 5.342143750180310846 ) ) ;
#2650=CARTESIAN_POINT ( 'NONE',  ( -2.870125741905213079, 6.929096494179683319, -15.15661249981968517 ) ) ;
#2653=CARTESIAN_POINT ( 'NONE',  ( -14.79893867758296544, 1.779018419858780125E-09, 14.83470808151907683 ) ) ;
#2658=CARTESIAN_POINT ( 'NONE',  ( -6.888301784570738384, -16.62983158437509346, -20.87113749981968880 ) ) ;
#2660=ORIENTED_EDGE ( 'NONE', *, *, #20515, .F. ) ;
#2670=CARTESIAN_POINT ( 'NONE',  ( -1.491842756249031510, -7.499999999820660790, -25.25041874981968704 ) ) ;
#2677=CARTESIAN_POINT ( 'NONE',  ( -10.19618095047498052, 15.25966317163203101, -10.11089374981968625 ) ) ;
#2684=CARTESIAN_POINT ( 'NONE',  ( 6.358192988180014993, 4.248408729364578917, -0.5097937498196938311 ) ) ;
#2687=CARTESIAN_POINT ( 'NONE',  ( -2.870125743571144028, -6.929096493489630859, -18.69098749981968410 ) ) ;
#2688=DIRECTION ( 'NONE',  ( 0.000000000000000000, 0.000000000000000000, -1.000000000000000000 ) ) ;
#2689=CARTESIAN_POINT ( 'NONE',  ( 17.99999999999999645, -2.163824016901520184E-09, -25.72104999981969442 ) ) ;
#2698=CARTESIAN_POINT ( 'NONE',  ( 3.580422610670020322, -18.00000000043041126, -12.32973124981968560 ) ) ;
#2710=CARTESIAN_POINT ( 'NONE',  ( 13.67243654642775574, -5.663308650141541278, -2.520645581158456938 ) ) ;
#2714=CARTESIAN_POINT ( 'NONE',  ( 2.870125741905212635, -6.929096494179677101, -26.13401249981969343 ) ) ;
#2715=CARTESIAN_POINT ( 'NONE',  ( 12.72792206288790773, 12.72792205982779912, 1.375825000180311175 ) ) ;
#2726=CARTESIAN_POINT ( 'NONE',  ( 15.25966317163202568, 10.19618095047498230, -17.17964374981969300 ) ) ;
#2736=CARTESIAN_POINT ( 'NONE',  ( 12.72792205982779912, -12.72792206288791483, 5.636675000180307649 ) ) ;
#2737=AXIS2_PLACEMENT_3D ( 'NONE', #16873, #20253, #19933 ) ;
#2745=CARTESIAN_POINT ( 'NONE',  ( 10.32494394706615637, -4.276731815070946574, -27.74104725028680463 ) ) ;
#2749=CARTESIAN_POINT ( 'NONE',  ( 16.62983158603122291, 6.888301780572502864, -14.98051249981969058 ) ) ;
#2751=VERTEX_POINT ( 'NONE', #6039 ) ;
#2763=CIRCLE ( 'NONE', #4454, 2.650000000000000355 ) ;
#2769=CARTESIAN_POINT ( 'NONE',  ( 7.500000000000000888, -9.015933403756337545E-10, -18.47619999981969130 ) ) ;
#2776=CARTESIAN_POINT ( 'NONE',  ( 3.580422614997668340, 17.99999999956958519, -8.932768749819690157 ) ) ;
#2779=ORIENTED_EDGE ( 'NONE', *, *, #6739, .T. ) ;
#2783=CARTESIAN_POINT ( 'NONE',  ( 4.248408729364576253, -6.358192988180015881, -7.578543749819692366 ) ) ;
#2801=LINE ( 'NONE', #6291, #11609 ) ;
#2804=CARTESIAN_POINT ( 'NONE',  ( 10.19618095047497874, -15.25966317163203279, -22.34379374981968880 ) ) ;
#2806=DIRECTION ( 'NONE',  ( -0.000000000000000000, -0.000000000000000000, 1.000000000000000000 ) ) ;
#2817=CARTESIAN_POINT ( 'NONE',  ( 10.46442989202484064, -10.46442989454075878, 7.493416918841544927 ) ) ;
#2818=VERTEX_POINT ( 'NONE', #17280 ) ;
#2824=CARTESIAN_POINT ( 'NONE',  ( 17.99999999999999645, -2.163824016901520184E-09, 11.97895000018031020 ) ) ;
#2825=CARTESIAN_POINT ( 'NONE',  ( -17.50000000000000355, 0.000000000000000000, -43.00000000000000000 ) ) ;
#2835=CARTESIAN_POINT ( 'NONE',  ( -3.580422610670017658, 18.00000000043040771, -18.94683124981969158 ) ) ;
#2838=CARTESIAN_POINT ( 'NONE',  ( -7.500000000000009770, 9.706494115329868228E-15, -7.498799999997683763 ) ) ;
#2841=FACE_BOUND ( 'NONE', #19630, .T. ) ;
#2844=CARTESIAN_POINT ( 'NONE',  ( -17.99999999956958874, 3.580422614997675002, 0.04058125018030836473 ) ) ;
#2847=CARTESIAN_POINT ( 'NONE',  ( 7.499999999820668783, -1.491842756249033508, -21.34176874981968908 ) ) ;
#2850=CARTESIAN_POINT ( 'NONE',  ( 5.663308650141530620, 13.67243654642775041, 8.355020581519076117 ) ) ;
#2853=ORIENTED_EDGE ( 'NONE', *, *, #6566, .F. ) ;
#2856=CARTESIAN_POINT ( 'NONE',  ( -12.72792205982779912, 12.72792206288790950, -17.92582499981968880 ) ) ;
#2857=LINE ( 'NONE', #13886, #920 ) ;
#2871=CARTESIAN_POINT ( 'NONE',  ( 7.902369978624329327, 7.902369976724401113, -12.96051524935257682 ) ) ;
#2874=CARTESIAN_POINT ( 'NONE',  ( -6.330490858644137298, -9.474249097082495297, 12.60973399971320141 ) ) ;
#2883=CARTESIAN_POINT ( 'NONE',  ( -3.580422610670018546, 18.00000000043041126, -9.521831249819687315 ) ) ;
#2897=CARTESIAN_POINT ( 'NONE',  ( -6.888301780572500199, 16.62983158603121936, -19.24136249981969016 ) ) ;
#2911=CARTESIAN_POINT ( 'NONE',  ( -10.19618095414378622, -15.25966316918061416, -11.15160624981969129 ) ) ;
#2927=CARTESIAN_POINT ( 'NONE',  ( 2.943691928843431782, 14.79893867722910628, 4.253573168841545460 ) ) ;
#2929=CARTESIAN_POINT ( 'NONE',  ( -6.929096494179678878, -2.870125741905209971, -14.35276249981969343 ) ) ;
#2935=CARTESIAN_POINT ( 'NONE',  ( -6.358192987158592047, 4.248408730893246776, -22.30510624981969414 ) ) ;
#2946=CARTESIAN_POINT ( 'NONE',  ( 1.491842754445842578, -7.500000000179340987, 2.435518750180307723 ) ) ;
#2947=CARTESIAN_POINT ( 'NONE',  ( -12.72792206288790950, -12.72792205982779556, -22.18667499981969726 ) ) ;
#2950=CARTESIAN_POINT ( 'NONE',  ( -9.015947181032835626E-10, -7.500000000000007994, -9.855049999819689432 ) ) ;
#2953=DIRECTION ( 'NONE',  ( 0.000000000000000000, 0.000000000000000000, -1.000000000000000000 ) ) ;
#2954=DIRECTION ( 'NONE',  ( -1.384478184788908018E-16, 1.611744734445712550E-26, 1.000000000000000000 ) ) ;
#2956=CARTESIAN_POINT ( 'NONE',  ( -17.99999999956958874, 3.580422614997675002, 9.465581250180308714 ) ) ;
#2958=CARTESIAN_POINT ( 'NONE',  ( 6.929096494179683319, 2.870125741905213079, -12.80036249981968766 ) ) ;
#2961=CARTESIAN_POINT ( 'NONE',  ( 2.943691925285397470, -14.79893867793683349, 12.18392683151907718 ) ) ;
#2983=CARTESIAN_POINT ( 'NONE',  ( 1.343451552857795926E-09, 11.17563879731705789, -14.13864024935257291 ) ) ;
#2984=CARTESIAN_POINT ( 'NONE',  ( -1.491842754445841246, 7.500000000179339210, -21.12698124981968917 ) ) ;
#2985=DIRECTION ( 'NONE',  ( 1.000000000000000000, 0.000000000000000000, 0.000000000000000000 ) ) ;
#2992=ORIENTED_EDGE ( 'NONE', *, *, #14380, .T. ) ;
#2993=CARTESIAN_POINT ( 'NONE',  ( 16.62983158603122291, 6.888301780572502864, -7.460112499819686604 ) ) ;
#2998=CARTESIAN_POINT ( 'NONE',  ( 7.500000000000004441, -8.788009017158368372E-15, -9.051199999997692203 ) ) ;
#3031=CARTESIAN_POINT ( 'NONE',  ( -9.474249098604513364, -6.330490856366295382, 20.32151600064743846 ) ) ;
#3038=CYLINDRICAL_SURFACE ( 'NONE', #14947, 7.500000000000000000 ) ;
#3054=CARTESIAN_POINT ( 'NONE',  ( -16.62983158603122646, -6.888301780572501976, -19.69301249981969448 ) ) ;
#3055=CARTESIAN_POINT ( 'NONE',  ( -9.015947181032835626E-10, -7.500000000000007994, -19.28004999981968481 ) ) ;
#3057=CARTESIAN_POINT ( 'NONE',  ( 13.67243654778934925, 5.663308646854335215, 9.533145581519077538 ) ) ;
#3062=CARTESIAN_POINT ( 'NONE',  ( 15.25966317163202746, 10.19618095047498407, -15.27504374981969093 ) ) ;
#3078=CARTESIAN_POINT ( 'NONE',  ( 11.17563879758428769, 2.222972768810838939, -12.07692149935257397 ) ) ;
#3079=CARTESIAN_POINT ( 'NONE',  ( 2.222972771497739419, 11.17563879704981922, 16.73317149971319751 ) ) ;
#3082=DIRECTION ( 'NONE',  ( -0.000000000000000000, -0.000000000000000000, -1.000000000000000000 ) ) ;
#3087=CARTESIAN_POINT ( 'NONE',  ( -3.580422614997675002, -17.99999999956958163, -13.64526874981969229 ) ) ;
#3094=EDGE_LOOP ( 'NONE', ( #5989, #19536 ) ) ;
#3095=CARTESIAN_POINT ( 'NONE',  ( 1.491842754445842578, -7.500000000179340987, -6.989481249819691655 ) ) ;
#3101=DIRECTION ( 'NONE',  ( -0.5000000000000037748, -0.8660254037844364872, 0.000000000000000000 ) ) ;
#3126=DIRECTION ( 'NONE',  ( -0.000000000000000000, -0.000000000000000000, 1.000000000000000000 ) ) ;
#3127=CARTESIAN_POINT ( 'NONE',  ( -14.79893867793684059, -2.943691925285399691, -17.54173933115846040 ) ) ;
#3144=CARTESIAN_POINT ( 'NONE',  ( 8.899999999999902656, -10.82531754730554496, 43.00000000000000000 ) ) ;
#3145=ORIENTED_EDGE ( 'NONE', *, *, #13625, .F. ) ;
#3157=CARTESIAN_POINT ( 'NONE',  ( 15.25966317163203101, 10.19618095047498585, -15.27504374981969448 ) ) ;
#3162=AXIS2_PLACEMENT_3D ( 'NONE', #6497, #13703, #6914 ) ;
#3164=CARTESIAN_POINT ( 'NONE',  ( -1.779019326032424095E-09, -14.79893867758296544, -6.371541918480928324 ) ) ;
#3165=EDGE_CURVE ( 'NONE', #9669, #6207, #1799, .T. ) ;
#3172=FACE_OUTER_BOUND ( 'NONE', #9902, .T. ) ;
#3187=SURFACE_SIDE_STYLE ('',( #11454 ) ) ;
#3188=CARTESIAN_POINT ( 'NONE',  ( 6.358192987158595599, -4.248408730893249441, 16.94729375018031803 ) ) ;
#3189=AXIS2_PLACEMENT_3D ( 'NONE', #11060, #4380, #6174 ) ;
#3190=CARTESIAN_POINT ( 'NONE',  ( 7.902369976724389566, -7.902369978624323110, 1.123015249713196217 ) ) ;
#3193=CARTESIAN_POINT ( 'NONE',  ( 0.000000000000000000, 0.000000000000000000, 40.00000000000000000 ) ) ;
#3198=CARTESIAN_POINT ( 'NONE',  ( 6.888301784570728614, 16.62983158437510056, 21.54136250018031618 ) ) ;
#3214=ORIENTED_EDGE ( 'NONE', *, *, #5337, .T. ) ;
#3217=CARTESIAN_POINT ( 'NONE',  ( -7.500000000000009770, 9.706494107251932559E-15, 1.926200000002316060 ) ) ;
#3225=FACE_BOUND ( 'NONE', #10330, .T. ) ;
#3227=AXIS2_PLACEMENT_3D ( 'NONE', #726, #3589, #527 ) ;
#3232=CARTESIAN_POINT ( 'NONE',  ( -7.902369976724401113, 7.902369978624329327, 22.38323475064743562 ) ) ;
#3240=CARTESIAN_POINT ( 'NONE',  ( -12.72792205982779912, 12.72792206288790950, 19.77417500018031404 ) ) ;
#3252=CARTESIAN_POINT ( 'NONE',  ( 5.303300859536635770, 5.303300858261589923, -3.964424999819686324 ) ) ;
#3258=CARTESIAN_POINT ( 'NONE',  ( -12.72792206288791483, -12.72792205982780089, -10.85707499981969448 ) ) ;
#3263=DIRECTION ( 'NONE',  ( 1.000000000000000000, 0.000000000000000000, 0.000000000000000000 ) ) ;
#3267=CARTESIAN_POINT ( 'NONE',  ( -12.54593441764187034, -8.382925368423267187, -4.898885668480925659 ) ) ;
#3281=CARTESIAN_POINT ( 'NONE',  ( -16.62983158603121936, -6.888301780572499311, 16.10238750018030984 ) ) ;
#3294=CARTESIAN_POINT ( 'NONE',  ( -2.870125741905213079, 6.929096494179683319, 22.54338750018031590 ) ) ;
#3296=CARTESIAN_POINT ( 'NONE',  ( 6.330490858644138186, 9.474249097082495297, -1.527766000286801873 ) ) ;
#3297=CIRCLE ( 'NONE', #13102, 17.50000000000000355 ) ;
#3304=CARTESIAN_POINT ( 'NONE',  ( 0.000000000000000000, 0.000000000000000000, 40.00000000000000000 ) ) ;
#3305=CARTESIAN_POINT ( 'NONE',  ( -17.99999999956958519, 3.580422614997674113, 18.89058125018031120 ) ) ;
#3318=COLOUR_RGB ( '', 0.31764706, 0.68627451, 0.89019608) ;
#3321=CARTESIAN_POINT ( 'NONE',  ( -2.870125743571140919, -6.929096493489624642, 12.74411250018031261 ) ) ;
#3322=CARTESIAN_POINT ( 'NONE',  ( -4.248408730893249441, -6.358192987158596488, 0.4535437501803143978 ) ) ;
#3327=CARTESIAN_POINT ( 'NONE',  ( -7.500000000000000000, 0.000000000000000000, 40.00000000000000000 ) ) ;
#3337=CARTESIAN_POINT ( 'NONE',  ( 13.67243654642775574, -5.663308650141541278, -11.94564558115845898 ) ) ;
#3346=FACE_OUTER_BOUND ( 'NONE', #4811, .T. ) ;
#3349=ORIENTED_EDGE ( 'NONE', *, *, #14687, .T. ) ;
#3358=CARTESIAN_POINT ( 'NONE',  ( -6.888301780572502864, 16.62983158603122646, -7.911762499819691818 ) ) ;
#3360=CARTESIAN_POINT ( 'NONE',  ( 6.929096494179677990, 2.870125741905210859, 9.209737500180310121 ) ) ;
#3361=DIRECTION ( 'NONE',  ( 0.000000000000000000, 0.000000000000000000, 1.000000000000000000 ) ) ;
#3362=CARTESIAN_POINT ( 'NONE',  ( -8.382925371439625906, -12.54593441562639988, 3.937051831519074341 ) ) ;
#3379=DIRECTION ( 'NONE',  ( 1.000000000000000000, 0.000000000000000000, 0.000000000000000000 ) ) ;
#3383=CARTESIAN_POINT ( 'NONE',  ( 7.500000000179346316, 1.491842754445843244, 25.19416875018031732 ) ) ;
#3385=CARTESIAN_POINT ( 'NONE',  ( -9.474249097082497073, 6.330490858644137298, 5.540983999713199992 ) ) ;
#3392=CARTESIAN_POINT ( 'NONE',  ( 6.888301780572507305, -16.62983158603121936, 15.65073750018031440 ) ) ;
#3410=CARTESIAN_POINT ( 'NONE',  ( -6.358192988180014993, -4.248408729364575365, 4.202706250180310299 ) ) ;
#3415=ADVANCED_FACE ( 'NONE', ( #2072 ), #13113, .F. ) ;
#3422=CARTESIAN_POINT ( 'NONE',  ( -12.50000000000000533, 0.000000000000000000, 43.00000000000000000 ) ) ;
#3432=CARTESIAN_POINT ( 'NONE',  ( 13.67243654642775574, -5.663308650141541278, -21.37064558115845614 ) ) ;
#3438=CARTESIAN_POINT ( 'NONE',  ( 7.499999999820663454, -1.491842756249032398, -27.60666874981969698 ) ) ;
#3441=CARTESIAN_POINT ( 'NONE',  ( 3.580422614997668340, 17.99999999956958519, 21.24683125018031404 ) ) ;
#3456=CARTESIAN_POINT ( 'NONE',  ( -10.19618095047498230, 15.25966317163203279, -8.206293749819689509 ) ) ;
#3458=CARTESIAN_POINT ( 'NONE',  ( -4.248408729364577141, 6.358192988180014993, 6.558956250180307812 ) ) ;
#3459=CARTESIAN_POINT ( 'NONE',  ( 10.46442989202483531, -10.46442989454075168, 1.875333081519072742 ) ) ;
#3480=CARTESIAN_POINT ( 'NONE',  ( -1.491842756249033064, -7.499999999820668783, 9.289481250180317673 ) ) ;
#3482=CARTESIAN_POINT ( 'NONE',  ( -10.32494394706615815, 4.276731815070940357, -4.178547250286804626 ) ) ;
#3490=CARTESIAN_POINT ( 'NONE',  ( -3.580422614997675002, -17.99999999956958163, 16.53433125018031191 ) ) ;
#3509=ORIENTED_EDGE ( 'NONE', *, *, #20613, .F. ) ;
#3511=CARTESIAN_POINT ( 'NONE',  ( 5.303300859536630441, 5.303300858261584594, 18.04567500018031367 ) ) ;
#3518=CARTESIAN_POINT ( 'NONE',  ( -6.358192987158597376, 4.248408730893249441, 2.809793750180315186 ) ) ;
#3529=VERTEX_POINT ( 'NONE', #18506 ) ;
#3536=CARTESIAN_POINT ( 'NONE',  ( 9.474249098604511587, 6.330490856366296271, 6.184016000647427624 ) ) ;
#3539=EDGE_CURVE ( 'NONE', #10636, #13652, #17953, .T. ) ;
#3556=CARTESIAN_POINT ( 'NONE',  ( 2.870125741905214412, -6.929096494179682431, -10.44411249981968481 ) ) ;
#3560=CARTESIAN_POINT ( 'NONE',  ( -2.943691925285397470, 14.79893867793684059, 13.08951066884154635 ) ) ;
#3564=CARTESIAN_POINT ( 'NONE',  ( -5.663308650141535949, -13.67243654642774686, -5.782479418480926725 ) ) ;
#3573=CARTESIAN_POINT ( 'NONE',  ( 9.015937996181835182E-10, 7.500000000000002665, 16.86755000018030870 ) ) ;
#3581=CARTESIAN_POINT ( 'NONE',  ( 7.500000000000007105, 4.207617034055637320E-15, 6.638700000002313750 ) ) ;
#3589=DIRECTION ( 'NONE',  ( -0.000000000000000000, -0.000000000000000000, -1.000000000000000000 ) ) ;
#3590=CARTESIAN_POINT ( 'NONE',  ( -2.870125741905213079, 6.929096494179683319, 13.11838750018031519 ) ) ;
#3591=CARTESIAN_POINT ( 'NONE',  ( -10.32494394706615815, 4.276731815070940357, 5.246452749713198749 ) ) ;
#3600=CARTESIAN_POINT ( 'NONE',  ( 10.19618095414378800, 15.25966316918061416, 12.41089375018031227 ) ) ;
#3602=ORIENTED_EDGE ( 'NONE', *, *, #388, .T. ) ;
#3617=CARTESIAN_POINT ( 'NONE',  ( -6.358192987158591158, 4.248408730893245000, 15.39489375018031403 ) ) ;
#3642=CARTESIAN_POINT ( 'NONE',  ( 4.276731812588570492, -10.32494394809439697, 8.834797250647429934 ) ) ;
#3650=CARTESIAN_POINT ( 'NONE',  ( 10.19618095414378800, 15.25966316918061416, 12.41089375018031227 ) ) ;
#3666=CARTESIAN_POINT ( 'NONE',  ( 14.79893867793684059, 2.943691925285398359, 24.87076066884155168 ) ) ;
#3667=ORIENTED_EDGE ( 'NONE', *, *, #12868, .T. ) ;
#3670=CARTESIAN_POINT ( 'NONE',  ( 13.67243654642774686, -5.663308650141536837, -26.98872941848093276 ) ) ;
#3674=ORIENTED_EDGE ( 'NONE', *, *, #10485, .T. ) ;
#3681=CARTESIAN_POINT ( 'NONE',  ( 10.19618095414378622, 15.25966316918061239, 10.50629375018031020 ) ) ;
#3688=CARTESIAN_POINT ( 'NONE',  ( 6.888301780572508193, -16.62983158603122291, 15.65073750018031262 ) ) ;
#3692=CARTESIAN_POINT ( 'NONE',  ( -4.248408730893249441, -6.358192987158595599, -8.971456249819688367 ) ) ;
#3693=CARTESIAN_POINT ( 'NONE',  ( -2.222972771497743416, -11.17563879704981566, -16.25432850028680676 ) ) ;
#3698=CARTESIAN_POINT ( 'NONE',  ( -6.888301780572501976, 16.62983158603122291, 1.513237500180310890 ) ) ;
#3712=CARTESIAN_POINT ( 'NONE',  ( -6.929096494179677101, -2.870125741905209527, 13.92223750018031225 ) ) ;
#3720=CARTESIAN_POINT ( 'NONE',  ( -6.888301784570738384, -16.62983158437509346, -3.925737499819687670 ) ) ;
#3732=CARTESIAN_POINT ( 'NONE',  ( -16.62983158603121936, -6.888301780572499311, -2.747612499819688914 ) ) ;
#3735=CARTESIAN_POINT ( 'NONE',  ( 6.330490858644141738, 9.474249097082498849, 5.594953500647431355 ) ) ;
#3744=CARTESIAN_POINT ( 'NONE',  ( 2.163825119083639534E-09, 18.00000000000000000, 11.52730000018031298 ) ) ;
#3754=CARTESIAN_POINT ( 'NONE',  ( 17.99999999999999645, -2.163824016901520184E-09, -25.72104999981969442 ) ) ;
#3757=CARTESIAN_POINT ( 'NONE',  ( -12.54593441562641054, 8.382925371439629458, 21.33638566884155097 ) ) ;
#3766=CARTESIAN_POINT ( 'NONE',  ( 1.779017513685135741E-09, 14.79893867758296544, -20.50904191848093205 ) ) ;
#3775=CARTESIAN_POINT ( 'NONE',  ( -6.358192988180021210, -4.248408729364580694, 10.46760625018031554 ) ) ;
#3776=VECTOR ( 'NONE', #16946, 1000.000000000000000 ) ;
#3777=ORIENTED_EDGE ( 'NONE', *, *, #14687, .F. ) ;
#3779=CARTESIAN_POINT ( 'NONE',  ( 17.99999999999999645, -2.163824016901520184E-09, 11.97895000018031020 ) ) ;
#3787=CARTESIAN_POINT ( 'NONE',  ( 18.00000000043041481, 3.580422610670020322, 23.01401875018030907 ) ) ;
#3790=CARTESIAN_POINT ( 'NONE',  ( -7.499999999820669672, 1.491842756249032620, -7.204268749819685347 ) ) ;
#3793=CARTESIAN_POINT ( 'NONE',  ( 11.17563879704981566, -2.222972771497744304, -18.61057850028680605 ) ) ;
#3797=ORIENTED_EDGE ( 'NONE', *, *, #11190, .F. ) ;
#3799=CARTESIAN_POINT ( 'NONE',  ( 18.00000000000000000, -2.163824016901520184E-09, 4.458550000180312445 ) ) ;
#3814=( BOUNDED_CURVE ( )  B_SPLINE_CURVE ( 2, ( #15292, #7122, #10210, #11897, #16470, #13405, #358, #16565, #2366, #5427, #8727, #16674, #1956, #6810, #2161, #8616, #13295 ),
 .UNSPECIFIED., .F., .F. ) 
 B_SPLINE_CURVE_WITH_KNOTS ( ( 3, 2, 2, 2, 2, 2, 2, 2, 3 ),
 ( 0.6000000000038511194, 0.6125000000038511860, 0.6250000000038511416, 0.6375000000038510972, 0.6500000000038511638, 0.6625000000038511194, 0.6750000000038511860, 0.6875000000038511416, 0.7000000000038510972 ),
 .UNSPECIFIED. ) 
 CURVE ( )  GEOMETRIC_REPRESENTATION_ITEM ( )  RATIONAL_B_SPLINE_CURVE ( ( 0.9999999999940800688, 0.9807852804091503618, 1.000000000000000000, 0.9807852804032304306, 1.000000000000000000, 0.9807852804032304306, 1.000000000000000000, 0.9807852804032304306, 1.000000000000000000, 0.9807852804032304306, 1.000000000000000000, 0.9807852804032304306, 1.000000000000000000, 0.9807852804032304306, 1.000000000000000000, 0.9807852803973104994, 1.000000000005919931 ) ) 
 REPRESENTATION_ITEM ( '' )  );
#3816=CARTESIAN_POINT ( 'NONE',  ( -2.870125741905209971, 6.929096494179676213, -2.571512499819690767 ) ) ;
#3821=DIRECTION ( 'NONE',  ( -0.000000000000000000, -0.000000000000000000, 1.000000000000000000 ) ) ;
#3826=CARTESIAN_POINT ( 'NONE',  ( 6.888301780572507305, -16.62983158603121936, -5.103862499819686427 ) ) ;
#3840=CARTESIAN_POINT ( 'NONE',  ( 3.580422610670019878, -18.00000000043040771, -4.809331249819688736 ) ) ;
#3845=CARTESIAN_POINT ( 'NONE',  ( -7.902369978624331104, -7.902369976724401113, 10.60198475064743029 ) ) ;
#3854=CARTESIAN_POINT ( 'NONE',  ( 10.19618095047497874, -15.25966317163203279, -3.493793749819687378 ) ) ;
#3860=EDGE_LOOP ( 'NONE', ( #4153, #19449 ) ) ;
#3869=CARTESIAN_POINT ( 'NONE',  ( -12.54593441764187745, -8.382925368423274293, 10.14419816884154457 ) ) ;
#3875=CARTESIAN_POINT ( 'NONE',  ( 3.580422614997667896, 17.99999999956958163, 19.34223125018031197 ) ) ;
#3877=PRODUCT_DEFINITION_FORMATION_WITH_SPECIFIED_SOURCE ( 'ANY', '', #5599, .NOT_KNOWN. ) ;
#3882=CARTESIAN_POINT ( 'NONE',  ( -7.500000000000007994, -1.491842754878806687, 11.05666875008779471 ) ) ;
#3883=EDGE_LOOP ( 'NONE', ( #5778, #20322, #19894, #20334 ) ) ;
#3886=CARTESIAN_POINT ( 'NONE',  ( 12.72792205982779379, -12.72792206288790950, 13.15707500018031162 ) ) ;
#3894=CARTESIAN_POINT ( 'NONE',  ( 7.500000000000009770, -8.788009009181406898E-15, -12.21129999999768501 ) ) ;
#3898=CARTESIAN_POINT ( 'NONE',  ( 7.500000000000007994, -9.015933403756345817E-10, -2.786299999819684459 ) ) ;
#3899=CARTESIAN_POINT ( 'NONE',  ( 6.358192987158596488, -4.248408730893249441, 16.94729375018031448 ) ) ;
#3901=CARTESIAN_POINT ( 'NONE',  ( 6.330490858644138186, 9.474249097082495297, -20.37776600028680818 ) ) ;
#3906=CARTESIAN_POINT ( 'NONE',  ( 16.62983158437509346, -6.888301784570739272, 5.047612500180314044 ) ) ;
#3924=CARTESIAN_POINT ( 'NONE',  ( -2.870125743571140919, -6.929096493489624642, -15.53088749981969308 ) ) ;
#3933=CARTESIAN_POINT ( 'NONE',  ( -6.888301784570738384, -16.62983158437509346, 5.499262500180314817 ) ) ;
#3935=ORIENTED_EDGE ( 'NONE', *, *, #17793, .T. ) ;
#3944=( BOUNDED_CURVE ( )  B_SPLINE_CURVE ( 2, ( #4637, #777, #19661, #13824, #13210, #10031, #2687, #998, #5141, #1977, #2583, #7442, #17212, #16496, #9148, #5530, #20372 ),
 .UNSPECIFIED., .F., .T. ) 
 B_SPLINE_CURVE_WITH_KNOTS ( ( 3, 2, 2, 2, 2, 2, 2, 2, 3 ),
 ( 0.9000000000038511638, 0.9125000000033697267, 0.9250000000028884006, 0.9375000000024069635, 0.9500000000019255264, 0.9625000000014442003, 0.9750000000009627632, 0.9875000000004814371, 1.000000000000000000 ),
 .UNSPECIFIED. ) 
 CURVE ( )  GEOMETRIC_REPRESENTATION_ITEM ( )  RATIONAL_B_SPLINE_CURVE ( ( 0.9999999999940800688, 0.9807852804091503618, 1.000000000000000000, 0.9807852804032304306, 1.000000000000000000, 0.9807852804032304306, 1.000000000000000000, 0.9807852804032304306, 1.000000000000000000, 0.9807852804032304306, 1.000000000000000000, 0.9807852804032304306, 1.000000000000000000, 0.9807852804032304306, 1.000000000000000000, 0.9807852804032304306, 1.000000000000000000 ) ) 
 REPRESENTATION_ITEM ( '' )  );
#3946=CARTESIAN_POINT ( 'NONE',  ( -2.163827323447877821E-09, -17.99999999999999645, -4.514799999819691934 ) ) ;
#3951=CARTESIAN_POINT ( 'NONE',  ( 4.276731815070943910, 10.32494394706616703, 5.300422250647430111 ) ) ;
#3954=EDGE_CURVE ( 'NONE', #10395, #6717, #6916, .T. ) ;
#3955=PLANE ( 'NONE',  #15253 ) ;
#3961=CARTESIAN_POINT ( 'NONE',  ( 18.00000000000000000, -2.163824016901520184E-09, 13.88355000018031404 ) ) ;
#3977=CARTESIAN_POINT ( 'NONE',  ( 18.00000000000000355, -2.163824016901520597E-09, -23.81644999981969590 ) ) ;
#3983=CARTESIAN_POINT ( 'NONE',  ( -13.67243654778935102, -5.663308646854334327, -23.45435441848093561 ) ) ;
#3993=CARTESIAN_POINT ( 'NONE',  ( 16.62983158603121936, 6.888301780572501976, 11.38988750018031126 ) ) ;
#3999=CARTESIAN_POINT ( 'NONE',  ( 6.358192988180019434, 4.248408729364581582, -13.09489374981968801 ) ) ;
#4001=CARTESIAN_POINT ( 'NONE',  ( 6.358192987158595599, -4.248408730893249441, -1.902706249819686279 ) ) ;
#4003=CARTESIAN_POINT ( 'NONE',  ( -11.17563879758427525, -2.222972768810838051, -14.48714100028680463 ) ) ;
#4004=DIRECTION ( 'NONE',  ( -1.000000000000000000, 0.000000000000000000, 0.000000000000000000 ) ) ;
#4010=CARTESIAN_POINT ( 'NONE',  ( -10.19618095047498052, 15.25966317163203101, -8.206293749819685956 ) ) ;
#4012=ORIENTED_EDGE ( 'NONE', *, *, #14999, .F. ) ;
#4026=DIRECTION ( 'NONE',  ( -0.000000000000000000, -0.000000000000000000, 1.000000000000000000 ) ) ;
#4028=CARTESIAN_POINT ( 'NONE',  ( -4.248408730893245000, -6.358192987158590270, -5.811356249819689346 ) ) ;
#4039=CARTESIAN_POINT ( 'NONE',  ( -16.62983158603122291, -6.888301780572501087, -2.747612499819685805 ) ) ;
#4050=CARTESIAN_POINT ( 'NONE',  ( -6.888301784570736608, -16.62983158437509346, -3.925737499819691223 ) ) ;
#4053=CARTESIAN_POINT ( 'NONE',  ( -1.343452921478824119E-09, -11.17563879731705789, -18.85114024935257149 ) ) ;
#4058=EDGE_LOOP ( 'NONE', ( #8111, #19918 ) ) ;
#4059=DIRECTION ( 'NONE',  ( 0.000000000000000000, 0.000000000000000000, -1.000000000000000000 ) ) ;
#4061=CARTESIAN_POINT ( 'NONE',  ( -18.00000000000000000, 2.163826221265758884E-09, -0.2539499998196886876 ) ) ;
#4067=CARTESIAN_POINT ( 'NONE',  ( -7.500000000000007994, 1.491842755816070287, 11.64573125008779186 ) ) ;
#4077=CARTESIAN_POINT ( 'NONE',  ( -13.67243654642775574, 5.663308650141533285, 2.191854418841544749 ) ) ;
#4082=CARTESIAN_POINT ( 'NONE',  ( 15.25966317163202568, 10.19618095047498230, 20.52035625018031340 ) ) ;
#4091=CARTESIAN_POINT ( 'NONE',  ( -2.870125743571141808, -6.929096493489625530, 3.319112500180309233 ) ) ;
#4092=CARTESIAN_POINT ( 'NONE',  ( 16.62983158437509346, -6.888301784570737496, -15.70698749981969122 ) ) ;
#4097=AXIS2_PLACEMENT_3D ( 'NONE', #13900, #19096, #20573 ) ;
#4107=CARTESIAN_POINT ( 'NONE',  ( -6.929096493489632635, 2.870125743571140919, -6.909737499819684992 ) ) ;
#4111=CARTESIAN_POINT ( 'NONE',  ( -6.330490858644137298, -9.474249097082495297, -25.09026600028681031 ) ) ;
#4116=CARTESIAN_POINT ( 'NONE',  ( 0.000000000000000000, 0.000000000000000000, 40.00000000000000000 ) ) ;
#4117=CARTESIAN_POINT ( 'NONE',  ( 6.888301780572507305, -16.62983158603121936, -12.62426249981968596 ) ) ;
#4132=ADVANCED_FACE ( 'NONE', ( #882 ), #7022, .F. ) ;
#4135=CARTESIAN_POINT ( 'NONE',  ( -1.491842754445841246, 7.500000000179339210, -2.276981249819689967 ) ) ;
#4147=CARTESIAN_POINT ( 'NONE',  ( 12.72792206288790950, 12.72792205982780089, 1.375825000180314728 ) ) ;
#4149=CIRCLE ( 'NONE', #8544, 2.649999999999999467 ) ;
#4153=ORIENTED_EDGE ( 'NONE', *, *, #11160, .F. ) ;
#4163=CARTESIAN_POINT ( 'NONE',  ( 17.99999999956957808, -3.580422614997675446, -6.576518749819691756 ) ) ;
#4167=EDGE_CURVE ( 'NONE', #9436, #10849, #999, .T. ) ;
#4169=CARTESIAN_POINT ( 'NONE',  ( 7.902369978624329327, 7.902369976724401113, -3.535515249352572997 ) ) ;
#4178=CARTESIAN_POINT ( 'NONE',  ( -6.888301780572501976, 16.62983158603122291, -17.33676249981968809 ) ) ;
#4185=LINE ( 'NONE', #5885, #12633 ) ;
#4197=CARTESIAN_POINT ( 'NONE',  ( 10.46442989454075700, 10.46442989202484419, -4.287833081158456849 ) ) ;
#4203=CARTESIAN_POINT ( 'NONE',  ( 12.72792205982779379, -12.72792206288790950, 3.732075000180308688 ) ) ;
#4215=CARTESIAN_POINT ( 'NONE',  ( -17.99999999956958163, 3.580422614997673669, -20.71401874981969371 ) ) ;
#4224=CARTESIAN_POINT ( 'NONE',  ( 3.580422614997669228, 17.99999999956958874, 2.396831250180309070 ) ) ;
#4225=CARTESIAN_POINT ( 'NONE',  ( 6.358192987158595599, -4.248408730893249441, -11.32770624981968588 ) ) ;
#4229=CARTESIAN_POINT ( 'NONE',  ( -10.46442989202483709, 10.46442989454075168, 6.587833081519073986 ) ) ;
#4250=CARTESIAN_POINT ( 'NONE',  ( -1.491842756249031510, -7.499999999820660790, -15.82541874981969343 ) ) ;
#4251=ADVANCED_FACE ( 'NONE', ( #4474 ), #1210, .T. ) ;
#4259=CARTESIAN_POINT ( 'NONE',  ( 3.580422610670020322, -18.00000000043041126, -23.65933124981968660 ) ) ;
#4264=ORIENTED_EDGE ( 'NONE', *, *, #17633, .F. ) ;
#4267=CARTESIAN_POINT ( 'NONE',  ( 0.000000000000000000, 0.000000000000000000, 43.00000000000000000 ) ) ;
#4287=CARTESIAN_POINT ( 'NONE',  ( -16.62983158603122291, -6.888301780572501087, -19.69301249981969093 ) ) ;
#4290=CARTESIAN_POINT ( 'NONE',  ( 0.000000000000000000, 0.000000000000000000, -43.00000000000000000 ) ) ;
#4295=ORIENTED_EDGE ( 'NONE', *, *, #9485, .F. ) ;
#4307=CARTESIAN_POINT ( 'NONE',  ( 8.382925368423272516, -12.54593441764187745, -1.637051831158454984 ) ) ;
#4315=CARTESIAN_POINT ( 'NONE',  ( 16.62983158437509346, -6.888301784570737496, 12.56801250018031091 ) ) ;
#4317=DIRECTION ( 'NONE',  ( -0.000000000000000000, -0.000000000000000000, -1.000000000000000000 ) ) ;
#4327=CARTESIAN_POINT ( 'NONE',  ( 6.888301780572505528, -16.62983158603121581, -14.52886249981968980 ) ) ;
#4329=ORIENTED_EDGE ( 'NONE', *, *, #2538, .F. ) ;
#4333=FACE_BOUND ( 'NONE', #8946, .T. ) ;
#4336=CARTESIAN_POINT ( 'NONE',  ( 16.62983158437509701, -6.888301784570740161, 5.047612500180310491 ) ) ;
#4341=EDGE_CURVE ( 'NONE', #8208, #9811, #9174, .T. ) ;
#4342=CARTESIAN_POINT ( 'NONE',  ( -14.79893867758296544, 1.779018419858780125E-09, 5.409708081519076117 ) ) ;
#4346=CARTESIAN_POINT ( 'NONE',  ( 10.19618095047497874, -15.25966317163203279, -22.34379374981968880 ) ) ;
#4350=ORIENTED_EDGE ( 'NONE', *, *, #17358, .T. ) ;
#4360=CARTESIAN_POINT ( 'NONE',  ( 6.358192987158590270, -4.248408730893245000, -27.01760624981969272 ) ) ;
#4362=DIRECTION ( 'NONE',  ( 0.000000000000000000, 0.000000000000000000, 1.000000000000000000 ) ) ;
#4367=CARTESIAN_POINT ( 'NONE',  ( -15.25966317163203279, -10.19618095047498052, -12.46714374981968909 ) ) ;
#4380=DIRECTION ( 'NONE',  ( -0.000000000000000000, -0.000000000000000000, 1.000000000000000000 ) ) ;
#4389=CARTESIAN_POINT ( 'NONE',  ( 6.888301780572507305, -16.62983158603121936, -22.04926249981969022 ) ) ;
#4393=EDGE_LOOP ( 'NONE', ( #9013, #20128 ) ) ;
#4403=CARTESIAN_POINT ( 'NONE',  ( -2.943691925285397470, 14.79893867793684059, 3.664510668841544305 ) ) ;
#4410=CARTESIAN_POINT ( 'NONE',  ( 15.25966317163202568, 10.19618095047498230, 11.09535625018031091 ) ) ;
#4421=CARTESIAN_POINT ( 'NONE',  ( 7.500000000000000888, 4.207617034106124418E-15, 0.3738000000023073421 ) ) ;
#4422=CARTESIAN_POINT ( 'NONE',  ( 17.99999999956957808, -3.580422614997675446, -6.576518749819692644 ) ) ;
#4428=CYLINDRICAL_SURFACE ( 'NONE', #11238, 7.500000000000000000 ) ;
#4431=CARTESIAN_POINT ( 'NONE',  ( 6.888301784570730391, 16.62983158437510411, 12.11636250018031014 ) ) ;
#4434=CARTESIAN_POINT ( 'NONE',  ( 4.248408729364579806, -6.358192988180021210, -20.16364374981968766 ) ) ;
#4438=CARTESIAN_POINT ( 'NONE',  ( -14.79893867793683349, -2.943691925285398359, 14.54017683151907647 ) ) ;
#4442=CARTESIAN_POINT ( 'NONE',  ( -18.00000000000000000, 2.163826221265758884E-09, -19.10394999981969022 ) ) ;
#4454=AXIS2_PLACEMENT_3D ( 'NONE', #11035, #17514, #2985 ) ;
#4460=CARTESIAN_POINT ( 'NONE',  ( 1.491842754445842134, -7.500000000179339210, -16.41448124981968704 ) ) ;
#4468=CARTESIAN_POINT ( 'NONE',  ( -10.19618095414378622, -15.25966316918061416, -13.05620624981969158 ) ) ;
#4474=FACE_OUTER_BOUND ( 'NONE', #17581, .T. ) ;
#4484=CARTESIAN_POINT ( 'NONE',  ( 10.19618095047497697, -15.25966317163202923, -24.24839374981969087 ) ) ;
#4498=CARTESIAN_POINT ( 'NONE',  ( 3.580422614997668340, 17.99999999956958519, -7.028168749819689864 ) ) ;
#4503=CARTESIAN_POINT ( 'NONE',  ( 9.470358143689555419, -1.138454911109683768E-09, 36.10922829754954932 ) ) ;
#4512=CARTESIAN_POINT ( 'NONE',  ( 5.663308646854342321, -13.67243654778935635, -10.76752058115845223 ) ) ;
#4517=( BOUNDED_CURVE ( )  B_SPLINE_CURVE ( 2, ( #19040, #10980, #2929, #15859, #8011, #1352, #7796, #14270, #12690, #15952, #1454, #19147, #14492, #4621, #11093, #17566, #20931 ),
 .UNSPECIFIED., .F., .T. ) 
 B_SPLINE_CURVE_WITH_KNOTS ( ( 3, 2, 2, 2, 2, 2, 2, 2, 3 ),
 ( 0.7000000000038510972, 0.7125000000038511638, 0.7250000000038511194, 0.7375000000038511860, 0.7500000000038511416, 0.7625000000038510972, 0.7750000000038511638, 0.7875000000038511194, 0.8000000000038511860 ),
 .UNSPECIFIED. ) 
 CURVE ( )  GEOMETRIC_REPRESENTATION_ITEM ( )  RATIONAL_B_SPLINE_CURVE ( ( 0.9999999999940800688, 0.9807852804091503618, 1.000000000000000000, 0.9807852804032304306, 1.000000000000000000, 0.9807852804032304306, 1.000000000000000000, 0.9807852804032304306, 1.000000000000000000, 0.9807852804032304306, 1.000000000000000000, 0.9807852804032304306, 1.000000000000000000, 0.9807852804032304306, 1.000000000000000000, 0.9807852803973104994, 1.000000000005919931 ) ) 
 REPRESENTATION_ITEM ( '' )  );
#4520=CARTESIAN_POINT ( 'NONE',  ( -17.99999999999999645, 2.163826221265758470E-09, 7.266450000180311619 ) ) ;
#4521=FACE_OUTER_BOUND ( 'NONE', #18629, .T. ) ;
#4531=CARTESIAN_POINT ( 'NONE',  ( -18.00000000043040771, -3.580422610670021211, -21.30308124981969442 ) ) ;
#4534=CARTESIAN_POINT ( 'NONE',  ( -4.248408730893249441, -6.358192987158596488, -8.971456249819688367 ) ) ;
#4538=LINE ( 'NONE', #17477, #8883 ) ;
#4541=CARTESIAN_POINT ( 'NONE',  ( 10.19618095047498052, -15.25966317163203456, 5.931206250180308004 ) ) ;
#4548=CARTESIAN_POINT ( 'NONE',  ( 10.46442989202483531, -10.46442989454075168, 11.30033308151907789 ) ) ;
#4570=CARTESIAN_POINT ( 'NONE',  ( -11.17563879704982988, 2.222972771497744748, -6.775358999352572908 ) ) ;
#4572=CARTESIAN_POINT ( 'NONE',  ( -5.303300859536631329, -5.303300858261583706, -24.36682499981969485 ) ) ;
#4579=DIRECTION ( 'NONE',  ( -1.000000000000000000, 0.000000000000000000, 0.000000000000000000 ) ) ;
#4581=CARTESIAN_POINT ( 'NONE',  ( -6.888301780572501976, 16.62983158603122291, -9.816362499819687670 ) ) ;
#4583=CARTESIAN_POINT ( 'NONE',  ( 17.99999999999999645, -2.163824016901520184E-09, 21.40395000018031268 ) ) ;
#4589=CARTESIAN_POINT ( 'NONE',  ( -5.303300858261584594, 5.303300859536631329, -3.160574999819691477 ) ) ;
#4605=CARTESIAN_POINT ( 'NONE',  ( 12.72792206288790950, 12.72792205982780089, -15.56957499981969129 ) ) ;
#4619=CARTESIAN_POINT ( 'NONE',  ( -14.79893867758297610, 1.779018419858781159E-09, -17.24720808115845827 ) ) ;
#4621=CARTESIAN_POINT ( 'NONE',  ( 6.358192987158592047, -4.248408730893246776, -17.59260624981969912 ) ) ;
#4637=CARTESIAN_POINT ( 'NONE',  ( -7.500000000000009770, 9.706494107251932559E-15, -16.92379999999768359 ) ) ;
#4638=CARTESIAN_POINT ( 'NONE',  ( 17.99999999999999645, -2.163824016901520184E-09, -25.72104999981969442 ) ) ;
#4646=( BOUNDED_CURVE ( )  B_SPLINE_CURVE ( 2, ( #6217, #17150, #10993, #12488, #18951, #17470, #4091, #18743, #10577, #2946, #17040, #20534, #19054, #6111, #8985, #942, #4421 ),
 .UNSPECIFIED., .F., .T. ) 
 B_SPLINE_CURVE_WITH_KNOTS ( ( 3, 2, 2, 2, 2, 2, 2, 2, 3 ),
 ( 0.3000000000038511860, 0.3125000000038511971, 0.3250000000038512082, 0.3375000000038512193, 0.3500000000038511749, 0.3625000000038511860, 0.3750000000038511971, 0.3875000000038512082, 0.4000000000038512193 ),
 .UNSPECIFIED. ) 
 CURVE ( )  GEOMETRIC_REPRESENTATION_ITEM ( )  RATIONAL_B_SPLINE_CURVE ( ( 0.9999999999940800688, 0.9807852804091503618, 1.000000000000000000, 0.9807852804032304306, 1.000000000000000000, 0.9807852804032304306, 1.000000000000000000, 0.9807852804032304306, 1.000000000000000000, 0.9807852804032304306, 1.000000000000000000, 0.9807852804032304306, 1.000000000000000000, 0.9807852804032304306, 1.000000000000000000, 0.9807852803973104994, 1.000000000005919931 ) ) 
 REPRESENTATION_ITEM ( '' )  );
#4647=CARTESIAN_POINT ( 'NONE',  ( 16.62983158603122646, 6.888301780572504640, -5.555512499819690753 ) ) ;
#4650=CARTESIAN_POINT ( 'NONE',  ( 5.303300858261588147, -5.303300859536636658, -20.45817499981968624 ) ) ;
#4655=CARTESIAN_POINT ( 'NONE',  ( 9.474249097082495297, -6.330490858644137298, -27.44651600028680960 ) ) ;
#4662=CARTESIAN_POINT ( 'NONE',  ( 12.72792205982779734, -12.72792206288791128, -13.21332499981968667 ) ) ;
#4676=CARTESIAN_POINT ( 'NONE',  ( -11.17563879704982988, 2.222972771497744748, -16.20035899935257362 ) ) ;
#4678=CARTESIAN_POINT ( 'NONE',  ( 4.276731815070940357, 10.32494394706615815, 17.02770274971319964 ) ) ;
#4682=DIRECTION ( 'NONE',  ( -1.000000000000000000, 0.000000000000000000, 0.000000000000000000 ) ) ;
#4686=CARTESIAN_POINT ( 'NONE',  ( -15.25966316918061771, 10.19618095414378622, -20.12495624981968945 ) ) ;
#4705=CARTESIAN_POINT ( 'NONE',  ( -5.303300859536636658, -5.303300858261589035, 0.7480750001803149196 ) ) ;
#4716=ORIENTED_EDGE ( 'NONE', *, *, #388, .F. ) ;
#4722=CARTESIAN_POINT ( 'NONE',  ( 12.54593441562640876, -8.382925371439629458, -11.65111433115845863 ) ) ;
#4729=CARTESIAN_POINT ( 'NONE',  ( -3.580422610670018546, 18.00000000043041126, 20.65776875018031333 ) ) ;
#4740=CARTESIAN_POINT ( 'NONE',  ( -3.580422614997674557, -17.99999999956957808, -23.07026874981968945 ) ) ;
#4742=DIRECTION ( 'NONE',  ( 1.202124453834178339E-10, 1.000000000000000000, -4.318160619762183323E-26 ) ) ;
#4745=CARTESIAN_POINT ( 'NONE',  ( 15.25966316918061771, -10.19618095414378800, -4.082856249819691641 ) ) ;
#4748=CARTESIAN_POINT ( 'NONE',  ( 8.382925368423265411, -12.54593441764187034, -7.255135668480925837 ) ) ;
#4755=CARTESIAN_POINT ( 'NONE',  ( 6.249999999999902300, -10.82531754730554496, -43.00000000000000000 ) ) ;
#4770=CARTESIAN_POINT ( 'NONE',  ( -9.474249098604513364, -6.330490856366295382, -17.37848399935257859 ) ) ;
#4772=CARTESIAN_POINT ( 'NONE',  ( -10.32494394809439164, -4.276731812588563386, 4.068327749713199104 ) ) ;
#4780=CARTESIAN_POINT ( 'NONE',  ( 12.72792206288790950, 12.72792205982780089, 22.13042500018031689 ) ) ;
#4793=DIRECTION ( 'NONE',  ( -0.5000000000000037748, -0.8660254037844364872, 0.000000000000000000 ) ) ;
#4796=VECTOR ( 'NONE', #11789, 1000.000000000000000 ) ;
#4802=CARTESIAN_POINT ( 'NONE',  ( -2.870125743571144028, -6.929096493489630859, 0.1590125001803138760 ) ) ;
#4811=EDGE_LOOP ( 'NONE', ( #7573, #362, #19048, #4329 ) ) ;
#4813=FACE_BOUND ( 'NONE', #3094, .T. ) ;
#4814=ORIENTED_EDGE ( 'NONE', *, *, #15573, .F. ) ;
#4816=EDGE_LOOP ( 'NONE', ( #13117, #15122, #2483, #11721 ) ) ;
#4822=CARTESIAN_POINT ( 'NONE',  ( -4.276731812588566939, 10.32494394809439875, 22.97229725064743278 ) ) ;
#4823=AXIS2_PLACEMENT_3D ( 'NONE', #9309, #1479, #19063 ) ;
#4844=CARTESIAN_POINT ( 'NONE',  ( 7.500000000000009770, 1.491842754878799138, -3.080831249912204584 ) ) ;
#4847=DIRECTION ( 'NONE',  ( 1.000000000000000000, 0.000000000000000000, 0.000000000000000000 ) ) ;
#4852=CARTESIAN_POINT ( 'NONE',  ( 3.580422610670021211, -18.00000000043041481, -12.32973124981968915 ) ) ;
#4854=ORIENTED_EDGE ( 'NONE', *, *, #1986, .F. ) ;
#4858=VECTOR ( 'NONE', #12114, 1000.000000000000000 ) ;
#4859=CARTESIAN_POINT ( 'NONE',  ( -10.46442989202483709, 10.46442989454075168, -12.26216691848092744 ) ) ;
#4862=CARTESIAN_POINT ( 'NONE',  ( 7.500000000000000000, -9.015933403756343749E-10, 25.48870000018031590 ) ) ;
#4871=CARTESIAN_POINT ( 'NONE',  ( -15.25966316918061416, 10.19618095414378445, 17.57504375018031340 ) ) ;
#4875=CIRCLE ( 'NONE', #131, 17.50000000000000355 ) ;
#4882=CARTESIAN_POINT ( 'NONE',  ( -5.303300859536636658, -5.303300858261589035, 19.59807500018031590 ) ) ;
#4884=CARTESIAN_POINT ( 'NONE',  ( -2.222972768810836275, 11.17563879758427525, 6.719108999713199637 ) ) ;
#4888=DIRECTION ( 'NONE',  ( -0.000000000000000000, -0.000000000000000000, -1.000000000000000000 ) ) ;
#4892=CARTESIAN_POINT ( 'NONE',  ( 12.72792206288790950, 12.72792205982780089, 12.70542500018031262 ) ) ;
#4907=CARTESIAN_POINT ( 'NONE',  ( 7.500000000000000888, -9.015933403756337545E-10, 19.22380000018031154 ) ) ;
#4915=CARTESIAN_POINT ( 'NONE',  ( -15.25966317163203279, -10.19618095047498052, 15.80785625018031659 ) ) ;
#4926=CARTESIAN_POINT ( 'NONE',  ( -6.330490858644140850, -9.474249097082498849, 19.73245350064743420 ) ) ;
#4933=EDGE_CURVE ( 'NONE', #20492, #16575, #10897, .T. ) ;
#4935=CARTESIAN_POINT ( 'NONE',  ( 2.163825119083639534E-09, 18.00000000000000000, 20.95230000018031546 ) ) ;
#4948=CARTESIAN_POINT ( 'NONE',  ( 6.888301780572505528, -16.62983158603121581, -23.95386249981969229 ) ) ;
#4950=DIRECTION ( 'NONE',  ( -0.000000000000000000, -0.000000000000000000, 1.000000000000000000 ) ) ;
#4953=CARTESIAN_POINT ( 'NONE',  ( -10.19618095414378800, -15.25966316918061771, -20.57660624981969733 ) ) ;
#4961=CARTESIAN_POINT ( 'NONE',  ( 5.663308650141530620, 13.67243654642775041, -10.49497941848093063 ) ) ;
#4968=CARTESIAN_POINT ( 'NONE',  ( -4.248408729364580694, 6.358192988180020322, 22.24885625018031732 ) ) ;
#4970=ORIENTED_EDGE ( 'NONE', *, *, #14140, .F. ) ;
#4987=CARTESIAN_POINT ( 'NONE',  ( 1.491842756249030622, 7.499999999820669672, 14.00198125018031625 ) ) ;
#4989=CARTESIAN_POINT ( 'NONE',  ( 1.343451552857795099E-09, 11.17563879731704723, 7.013640249713197328 ) ) ;
#4994=CIRCLE ( 'NONE', #1296, 2.649999999999999467 ) ;
#4996=CARTESIAN_POINT ( 'NONE',  ( 6.888301780572507305, -16.62983158603121936, 6.225737500180312800 ) ) ;
#5013=CARTESIAN_POINT ( 'NONE',  ( -6.929096494179677101, -2.870125741905209527, 4.497237500180311542 ) ) ;
#5020=CARTESIAN_POINT ( 'NONE',  ( -2.163827323447878234E-09, -18.00000000000000000, 14.33520000018031482 ) ) ;
#5030=CARTESIAN_POINT ( 'NONE',  ( -2.943691928843437999, -14.79893867722910450, -19.30892683115845543 ) ) ;
#5035=CARTESIAN_POINT ( 'NONE',  ( -18.00000000000000000, 2.163826221265758884E-09, 18.59605000018031262 ) ) ;
#5049=CARTESIAN_POINT ( 'NONE',  ( -18.00000000043041481, -3.580422610670022987, -9.973481249819691641 ) ) ;
#5054=CARTESIAN_POINT ( 'NONE',  ( -12.54593441562640166, 8.382925371439625906, -12.55669816848092779 ) ) ;
#5055=CARTESIAN_POINT ( 'NONE',  ( -17.50000000000000355, 0.000000000000000000, 43.00000000000000000 ) ) ;
#5058=CARTESIAN_POINT ( 'NONE',  ( -6.929096493489632635, 2.870125743571140919, 21.36526250018031803 ) ) ;
#5065=CARTESIAN_POINT ( 'NONE',  ( 10.19618095414378622, 15.25966316918061239, 19.93129375018031268 ) ) ;
#5075=EDGE_CURVE ( 'NONE', #9398, #10361, #4646, .T. ) ;
#5076=CARTESIAN_POINT ( 'NONE',  ( -6.929096494179684207, -2.870125741905212635, 10.76213750018031590 ) ) ;
#5078=CARTESIAN_POINT ( 'NONE',  ( -9.474249098604506258, -6.330490856366290053, 3.773796499713198305 ) ) ;
#5085=CARTESIAN_POINT ( 'NONE',  ( -18.00000000043041126, -3.580422610670022543, 18.30151875018031760 ) ) ;
#5098=CARTESIAN_POINT ( 'NONE',  ( -15.15000000000000568, -3.245314017740485469E-16, -40.00000000000000000 ) ) ;
#5101=CARTESIAN_POINT ( 'NONE',  ( -5.303300859536631329, -5.303300858261583706, 13.33317500018031332 ) ) ;
#5107=CARTESIAN_POINT ( 'NONE',  ( 16.62983158437509346, -6.888301784570739272, -23.22738749981969164 ) ) ;
#5109=CARTESIAN_POINT ( 'NONE',  ( 18.00000000043041126, 3.580422610670019434, 21.10941875018031411 ) ) ;
#5122=CARTESIAN_POINT ( 'NONE',  ( -2.222972771497745192, -11.17563879704982632, 0.2933910006474270693 ) ) ;
#5127=CARTESIAN_POINT ( 'NONE',  ( 8.900000000000053646, 10.82531754730546147, 40.00000000000000000 ) ) ;
#5141=CARTESIAN_POINT ( 'NONE',  ( -9.015947181032835626E-10, -7.500000000000007994, -19.28004999981968481 ) ) ;
#5147=CARTESIAN_POINT ( 'NONE',  ( 13.67243654778935991, 5.663308646854338768, 24.57622941884154955 ) ) ;
#5152=CARTESIAN_POINT ( 'NONE',  ( -12.54593441562640166, 8.382925371439625906, -3.131698168480926192 ) ) ;
#5158=STYLED_ITEM ( 'NONE', ( #17714 ), #10096 ) ;
#5160=CYLINDRICAL_SURFACE ( 'NONE', #17836, 2.649999999999999467 ) ;
#5167=CARTESIAN_POINT ( 'NONE',  ( -10.19618095047497874, 15.25966317163202746, 18.16410625018031411 ) ) ;
#5180=CARTESIAN_POINT ( 'NONE',  ( 2.870125743571140475, 6.929096493489632635, 23.72151250018031732 ) ) ;
#5181=CARTESIAN_POINT ( 'NONE',  ( 11.17563879731704723, -1.343450868547281106E-09, 9.369890249713199282 ) ) ;
#5185=AXIS2_PLACEMENT_3D ( 'NONE', #14817, #19473, #3263 ) ;
#5190=CARTESIAN_POINT ( 'NONE',  ( 18.00000000043041126, 3.580422610670019434, 13.58901875018031369 ) ) ;
#5211=AXIS2_PLACEMENT_3D ( 'NONE', #16868, #15071, #10619 ) ;
#5214=CARTESIAN_POINT ( 'NONE',  ( -5.303300858261583706, 5.303300859536630441, 6.264425000180311010 ) ) ;
#5223=CARTESIAN_POINT ( 'NONE',  ( 6.888301780572507305, -16.62983158603121936, 13.74613750018031588 ) ) ;
#5237=CARTESIAN_POINT ( 'NONE',  ( -11.17563879704982988, 2.222972771497744748, 12.07464100064743029 ) ) ;
#5244=AXIS2_PLACEMENT_3D ( 'NONE', #17966, #19447, #9903 ) ;
#5246=CARTESIAN_POINT ( 'NONE',  ( -15.25966316918061771, 10.19618095414378622, 10.05464375018031475 ) ) ;
#5248=FACE_OUTER_BOUND ( 'NONE', #18113, .T. ) ;
#5261=CARTESIAN_POINT ( 'NONE',  ( -2.943691928843437999, -14.79893867722910450, 18.39107316884155097 ) ) ;
#5264=CARTESIAN_POINT ( 'NONE',  ( 10.46442989202483531, -10.46442989454075168, -16.97466691848093134 ) ) ;
#5270=CARTESIAN_POINT ( 'NONE',  ( 7.500000000179340987, 1.491842754445842134, 18.92926875018030941 ) ) ;
#5272=CARTESIAN_POINT ( 'NONE',  ( 5.303300858261588147, -5.303300859536636658, 7.816825000180313232 ) ) ;
#5275=CARTESIAN_POINT ( 'NONE',  ( 6.888301780572505528, -16.62983158603121581, 13.74613750018031233 ) ) ;
#5283=CARTESIAN_POINT ( 'NONE',  ( -5.303300858261589035, 5.303300859536635770, -15.74567499981968588 ) ) ;
#5288=CARTESIAN_POINT ( 'NONE',  ( -5.303300858261589035, 5.303300859536635770, -6.320674999819683393 ) ) ;
#5289=CARTESIAN_POINT ( 'NONE',  ( -1.343452921478823292E-09, -11.17563879731704723, -16.54885975028680889 ) ) ;
#5297=CARTESIAN_POINT ( 'NONE',  ( -12.72792205982779912, 12.72792206288790950, -8.500824999819686312 ) ) ;
#5314=CARTESIAN_POINT ( 'NONE',  ( 4.248408730893245888, 6.358192987158590270, 8.326143750180312608 ) ) ;
#5321=CARTESIAN_POINT ( 'NONE',  ( 4.248408730893249441, 6.358192987158596488, 5.166043750180316252 ) ) ;
#5335=CARTESIAN_POINT ( 'NONE',  ( -17.99999999956958163, 3.580422614997673669, -1.864018749819690957 ) ) ;
#5337=EDGE_CURVE ( 'NONE', #8415, #19935, #3944, .T. ) ;
#5339=CARTESIAN_POINT ( 'NONE',  ( -10.32494394809439875, -4.276731812588566051, 11.19104725064742745 ) ) ;
#5347=CARTESIAN_POINT ( 'NONE',  ( 3.580422610670020322, -18.00000000043041126, 6.520268750180314932 ) ) ;
#5357=LINE ( 'NONE', #498, #2619 ) ;
#5361=CARTESIAN_POINT ( 'NONE',  ( 2.943691928843431782, 14.79893867722910628, 13.67857316884154706 ) ) ;
#5366=CARTESIAN_POINT ( 'NONE',  ( -16.62983158437509701, 6.888301784570728614, 17.28051250018031126 ) ) ;
#5369=AXIS2_PLACEMENT_3D ( 'NONE', #20468, #5946, #7426 ) ;
#5370=ORIENTED_EDGE ( 'NONE', *, *, #8651, .F. ) ;
#5374=CARTESIAN_POINT ( 'NONE',  ( -7.500000000000007105, -3.289131931996631318E-15, 11.35120000000231677 ) ) ;
#5377=CARTESIAN_POINT ( 'NONE',  ( -15.25966317163202923, -10.19618095047497874, -3.042143749819689713 ) ) ;
#5386=CARTESIAN_POINT ( 'NONE',  ( 1.491842756249030622, 7.499999999820669672, -4.848018749819687834 ) ) ;
#5388=CARTESIAN_POINT ( 'NONE',  ( -9.474249097082497073, 6.330490858644137298, -13.30901600028680321 ) ) ;
#5394=CARTESIAN_POINT ( 'NONE',  ( 12.72792206288790950, 12.72792205982780089, -6.144574999819688799 ) ) ;
#5407=CARTESIAN_POINT ( 'NONE',  ( 4.248408730893245888, 6.358192987158590270, -1.098856249819687880 ) ) ;
#5416=CARTESIAN_POINT ( 'NONE',  ( -17.99999999956958519, 3.580422614997674113, -1.864018749819687404 ) ) ;
#5426=ORIENTED_EDGE ( 'NONE', *, *, #9500, .T. ) ;
#5427=CARTESIAN_POINT ( 'NONE',  ( -1.491842754445841690, 7.500000000179340987, -11.70198124981969201 ) ) ;
#5428=CARTESIAN_POINT ( 'NONE',  ( -2.163827323447877821E-09, -17.99999999999999645, -13.93979999981969442 ) ) ;
#5433=CARTESIAN_POINT ( 'NONE',  ( -7.902369976724401113, 7.902369978624329327, 3.533234750647429312 ) ) ;
#5440=CARTESIAN_POINT ( 'NONE',  ( 16.62983158437509346, -6.888301784570739272, 5.047612500180314044 ) ) ;
#5450=DIRECTION ( 'NONE',  ( 0.000000000000000000, 0.000000000000000000, -1.000000000000000000 ) ) ;
#5456=CARTESIAN_POINT ( 'NONE',  ( 13.67243654642775574, -5.663308650141541278, 16.32935441884154315 ) ) ;
#5464=CARTESIAN_POINT ( 'NONE',  ( -8.382925371439625906, -12.54593441562639988, -14.91294816848093063 ) ) ;
#5470=CARTESIAN_POINT ( 'NONE',  ( 6.358192988180014993, 4.248408729364578917, 18.34020625018030870 ) ) ;
#5472=CARTESIAN_POINT ( 'NONE',  ( 6.929096493489630859, -2.870125743571144472, 7.227762500180316074 ) ) ;
#5476=CARTESIAN_POINT ( 'NONE',  ( 6.888301784570727726, 16.62983158437509701, 0.7867625001803102425 ) ) ;
#5484=CARTESIAN_POINT ( 'NONE',  ( -2.870125741905213079, 6.929096494179683319, -15.15661249981968517 ) ) ;
#5486=CARTESIAN_POINT ( 'NONE',  ( 2.870125741905214412, -6.929096494179682431, 8.405887500180314831 ) ) ;
#5489=CARTESIAN_POINT ( 'NONE',  ( 4.276731815070940357, 10.32494394706615815, -20.67229725028680676 ) ) ;
#5494=CARTESIAN_POINT ( 'NONE',  ( 12.72792205982779734, -12.72792206288791128, 5.636675000180311201 ) ) ;
#5511=CARTESIAN_POINT ( 'NONE',  ( -6.358192988180014993, -4.248408729364575365, -14.64729374981969023 ) ) ;
#5519=CARTESIAN_POINT ( 'NONE',  ( -1.491842754445842800, 7.500000000179346316, 3.987918750180313943 ) ) ;
#5521=CARTESIAN_POINT ( 'NONE',  ( 16.62983158603122291, 6.888301780572502864, 11.38988750018031482 ) ) ;
#5530=CARTESIAN_POINT ( 'NONE',  ( 7.499999999820668783, -1.491842756249033508, -21.34176874981968908 ) ) ;
#5534=CARTESIAN_POINT ( 'NONE',  ( 10.19618095047497697, -15.25966317163202923, -5.398393749819690335 ) ) ;
#5539=CARTESIAN_POINT ( 'NONE',  ( 4.276731812588570492, -10.32494394809439697, 18.25979725064743064 ) ) ;
#5548=CARTESIAN_POINT ( 'NONE',  ( 12.72792205982779734, -12.72792206288791128, 5.636675000180311201 ) ) ;
#5551=AXIS2_PLACEMENT_3D ( 'NONE', #36, #14866, #13073 ) ;
#5561=CARTESIAN_POINT ( 'NONE',  ( 12.72792205982779912, -12.72792206288791483, -22.63832499981969448 ) ) ;
#5562=CLOSED_SHELL ( 'NONE', ( #9857, #3415, #19859, #1195, #9801, #11703, #1979, #4251, #5743, #1423, #330, #11161, #20489, #10250, #1043, #18198, #7805, #6852, #9105, #18806, #10004, #13453, #2029, #16698, #11565, #15940, #19724, #10764, #19551, #13006, #17137, #7800, #14299, #16582, #4132, #8187, #7374 ) ) ;
#5568=CARTESIAN_POINT ( 'NONE',  ( 5.663308646854338768, -13.67243654778934747, -25.81060441848093134 ) ) ;
#5574=CARTESIAN_POINT ( 'NONE',  ( 0.000000000000000000, 0.000000000000000000, 43.00000000000000000 ) ) ;
#5581=CARTESIAN_POINT ( 'NONE',  ( 16.62983158437509346, -6.888301784570737496, 12.56801250018031091 ) ) ;
#5588=CARTESIAN_POINT ( 'NONE',  ( -15.25966316918061949, 10.19618095414378800, 19.47964375018031191 ) ) ;
#5594=CARTESIAN_POINT ( 'NONE',  ( 5.303300858261588147, -5.303300859536636658, -1.608174999819685702 ) ) ;
#5595=CARTESIAN_POINT ( 'NONE',  ( -6.358192988180021210, -4.248408729364580694, 19.89260625018031803 ) ) ;
#5597=CARTESIAN_POINT ( 'NONE',  ( 9.474249098604504482, 6.330490856366291830, -10.36370350028680321 ) ) ;
#5599=PRODUCT ( 'worm', 'worm', '', ( #12144 ) ) ;
#5603=CARTESIAN_POINT ( 'NONE',  ( -15.25966317163203279, -10.19618095047498052, -10.56254374981969058 ) ) ;
#5622=CARTESIAN_POINT ( 'NONE',  ( -5.303300859536631329, -5.303300858261583706, -5.516824999819688990 ) ) ;
#5628=VECTOR ( 'NONE', #8952, 1000.000000000000000 ) ;
#5632=CARTESIAN_POINT ( 'NONE',  ( -7.500000000000009770, 9.706494107251932559E-15, 1.926200000002316060 ) ) ;
#5634=CARTESIAN_POINT ( 'NONE',  ( 15.25966316918061416, -10.19618095414378622, 3.437543750180314994 ) ) ;
#5636=ORIENTED_EDGE ( 'NONE', *, *, #4933, .T. ) ;
#5646=CARTESIAN_POINT ( 'NONE',  ( 10.19618095414378622, 15.25966316918061239, -17.76870624981969371 ) ) ;
#5647=LINE ( 'NONE', #12123, #6896 ) ;
#5650=CARTESIAN_POINT ( 'NONE',  ( 9.474249098604511587, 6.330490856366296271, -3.240983999352573086 ) ) ;
#5657=EDGE_LOOP ( 'NONE', ( #20578, #2412, #16192, #17829 ) ) ;
#5660=CARTESIAN_POINT ( 'NONE',  ( 6.888301784570728614, 16.62983158437510056, 2.691362500180312978 ) ) ;
#5667=CARTESIAN_POINT ( 'NONE',  ( 6.358192988180019434, 4.248408729364581582, 15.18010625018031590 ) ) ;
#5674=CARTESIAN_POINT ( 'NONE',  ( 10.46442989202484064, -10.46442989454075878, -1.931583081158455562 ) ) ;
#5679=CARTESIAN_POINT ( 'NONE',  ( 5.663308646854338768, -13.67243654778934747, -16.38560441848093063 ) ) ;
#5689=CARTESIAN_POINT ( 'NONE',  ( -3.580422614997674557, -17.99999999956957808, 5.204731250180310909 ) ) ;
#5698=CARTESIAN_POINT ( 'NONE',  ( -12.72792206288791483, -12.72792205982780089, 17.41792500018031120 ) ) ;
#5700=CARTESIAN_POINT ( 'NONE',  ( 9.015937996181842420E-10, 7.500000000000007994, 4.282450000180314298 ) ) ;
#5702=CARTESIAN_POINT ( 'NONE',  ( 6.330490856366289165, -9.474249098604506258, -17.43245350028680107 ) ) ;
#5707=CARTESIAN_POINT ( 'NONE',  ( -18.00000000043041126, -3.580422610670022543, -0.5484812498196892649 ) ) ;
#5723=CARTESIAN_POINT ( 'NONE',  ( 5.303300859536630441, 5.303300858261584594, -0.8043249998196875250 ) ) ;
#5735=CARTESIAN_POINT ( 'NONE',  ( -18.00000000043041126, -3.580422610670022543, -2.453081249819689003 ) ) ;
#5743=ADVANCED_FACE ( 'NONE', ( #16336 ), #8088, .T. ) ;
#5747=CARTESIAN_POINT ( 'NONE',  ( 2.163825119083639120E-09, 17.99999999999999645, -18.65229999981968945 ) ) ;
#5750=CARTESIAN_POINT ( 'NONE',  ( 2.222972768810839383, -11.17563879758428769, -9.720671499352569356 ) ) ;
#5758=CARTESIAN_POINT ( 'NONE',  ( -3.580422610670018546, 18.00000000043041126, -7.617231249819687910 ) ) ;
#5775=CARTESIAN_POINT ( 'NONE',  ( 13.67243654778935991, 5.663308646854338768, 5.726229418841543684 ) ) ;
#5778=ORIENTED_EDGE ( 'NONE', *, *, #15573, .T. ) ;
#5780=CARTESIAN_POINT ( 'NONE',  ( -15.25966317163202923, -10.19618095047497874, 6.382856250180309665 ) ) ;
#5781=CARTESIAN_POINT ( 'NONE',  ( -7.500000000000000888, 1.491842755816075172, -22.89416874991221462 ) ) ;
#5790=EDGE_LOOP ( 'NONE', ( #2125, #17938, #8399, #2575 ) ) ;
#5792=CARTESIAN_POINT ( 'NONE',  ( -10.19618095414378445, -15.25966316918061239, -13.05620624981969335 ) ) ;
#5803=CARTESIAN_POINT ( 'NONE',  ( -3.580422610670018990, 18.00000000043041481, 1.807768750180308137 ) ) ;
#5805=CARTESIAN_POINT ( 'NONE',  ( -6.358192988180021210, -4.248408729364580694, -17.80739374981969192 ) ) ;
#5807=CIRCLE ( 'NONE', #17675, 2.649999999999998579 ) ;
#5810=CARTESIAN_POINT ( 'NONE',  ( -14.79893867722910095, 2.943691928843434891, 15.12923933151907718 ) ) ;
#5816=CARTESIAN_POINT ( 'NONE',  ( -10.19618095414378622, -15.25966316918061416, -20.57660624981969377 ) ) ;
#5824=CARTESIAN_POINT ( 'NONE',  ( -12.50000000000000533, 0.000000000000000000, 43.00000000000000000 ) ) ;
#5834=EDGE_CURVE ( 'NONE', #14416, #14958, #20162, .T. ) ;
#5835=CARTESIAN_POINT ( 'NONE',  ( 5.303300859536630441, 5.303300858261584594, -10.22932499981969023 ) ) ;
#5845=CARTESIAN_POINT ( 'NONE',  ( 16.62983158437509346, -6.888301784570739272, 3.143012500180314639 ) ) ;
#5862=CARTESIAN_POINT ( 'NONE',  ( 7.500000000000004441, -8.788009017158368372E-15, -9.051199999997692203 ) ) ;
#5878=CARTESIAN_POINT ( 'NONE',  ( 18.00000000000000000, -2.163824016901520184E-09, -14.39144999981968986 ) ) ;
#5885=CARTESIAN_POINT ( 'NONE',  ( 7.500000000000000000, 9.184850993605147944E-16, 40.00000000000000000 ) ) ;
#5895=CARTESIAN_POINT ( 'NONE',  ( 12.54593441562640876, -8.382925371439629458, 7.198885668841548124 ) ) ;
#5900=CARTESIAN_POINT ( 'NONE',  ( 3.580422610670019878, -18.00000000043040771, 4.615668750180310198 ) ) ;
#5911=CARTESIAN_POINT ( 'NONE',  ( -2.163827323447877821E-09, -17.99999999999999645, -4.514799999819691934 ) ) ;
#5917=CARTESIAN_POINT ( 'NONE',  ( 0.000000000000000000, 0.000000000000000000, -43.00000000000000000 ) ) ;
#5920=CARTESIAN_POINT ( 'NONE',  ( 16.62983158603122646, 6.888301780572504640, 3.869487500180308182 ) ) ;
#5921=CARTESIAN_POINT ( 'NONE',  ( 6.929096493489630859, -2.870125743571144472, -21.04723749981969050 ) ) ;
#5922=ORIENTED_EDGE ( 'NONE', *, *, #13166, .T. ) ;
#5925=CARTESIAN_POINT ( 'NONE',  ( -12.54593441562640166, 8.382925371439625906, 6.293301831519076295 ) ) ;
#5931=CARTESIAN_POINT ( 'NONE',  ( 12.72792206288790950, 12.72792205982780089, -15.56957499981969129 ) ) ;
#5944=CARTESIAN_POINT ( 'NONE',  ( -9.015947181032828388E-10, -7.500000000000000888, -25.54494999981968917 ) ) ;
#5946=DIRECTION ( 'NONE',  ( 1.202124453834178339E-10, 1.000000000000000000, -1.511356216916759083E-25 ) ) ;
#5951=CARTESIAN_POINT ( 'NONE',  ( 2.163825119083639534E-09, 18.00000000000000000, -18.65229999981968589 ) ) ;
#5960=CARTESIAN_POINT ( 'NONE',  ( -2.870125741905210415, 6.929096494179677990, -2.571512499819693875 ) ) ;
#5969=CARTESIAN_POINT ( 'NONE',  ( -4.248408730893246776, -6.358192987158592047, 13.03864375018031119 ) ) ;
#5970=EDGE_CURVE ( 'NONE', #15394, #197, #6144, .T. ) ;
#5974=DIRECTION ( 'NONE',  ( -0.000000000000000000, -0.000000000000000000, 1.000000000000000000 ) ) ;
#5981=CARTESIAN_POINT ( 'NONE',  ( 6.888301784570728614, 16.62983158437510056, -16.15863749981969377 ) ) ;
#5988=VECTOR ( 'NONE', #10698, 1000.000000000000000 ) ;
#5989=ORIENTED_EDGE ( 'NONE', *, *, #14052, .T. ) ;
#5999=CARTESIAN_POINT ( 'NONE',  ( -13.67243654778936168, -5.663308646854336992, -8.411270581158460047 ) ) ;
#6005=CARTESIAN_POINT ( 'NONE',  ( 6.888301780572505528, -16.62983158603121581, 4.321137500180309843 ) ) ;
#6007=CARTESIAN_POINT ( 'NONE',  ( 2.870125743571138255, 6.929096493489627306, -20.24338749981969698 ) ) ;
#6012=DIRECTION ( 'NONE',  ( -0.4999999999999918954, 0.8660254037844433705, 0.000000000000000000 ) ) ;
#6018=CARTESIAN_POINT ( 'NONE',  ( -10.19618095047497874, 15.25966317163202746, -10.11089374981968803 ) ) ;
#6028=CARTESIAN_POINT ( 'NONE',  ( 6.888301780572508193, -16.62983158603122291, 6.225737500180309247 ) ) ;
#6032=CARTESIAN_POINT ( 'NONE',  ( -10.46442989454075168, -10.46442989202483709, 4.231583081519074696 ) ) ;
#6036=CARTESIAN_POINT ( 'NONE',  ( 15.25966316918061416, -10.19618095414378622, -13.50785624981968880 ) ) ;
#6039=CARTESIAN_POINT ( 'NONE',  ( -7.500000000000004441, 9.706494107352906755E-15, -23.18869999999769860 ) ) ;
#6050=CARTESIAN_POINT ( 'NONE',  ( -7.902369978624323110, -7.902369976724391343, 12.90426524971319999 ) ) ;
#6057=CARTESIAN_POINT ( 'NONE',  ( 6.888301784570728614, 16.62983158437510056, -8.638237499819689802 ) ) ;
#6080=CARTESIAN_POINT ( 'NONE',  ( 12.72792205982779734, -12.72792206288791128, -22.63832499981969093 ) ) ;
#6083=VERTEX_POINT ( 'NONE', #15897 ) ;
#6092=CARTESIAN_POINT ( 'NONE',  ( -1.779019326032424922E-09, -14.79893867758297610, -10.17845808115846218 ) ) ;
#6099=CARTESIAN_POINT ( 'NONE',  ( -3.580422614997674557, -17.99999999956957808, 14.62973125018031162 ) ) ;
#6106=DIRECTION ( 'NONE',  ( -0.000000000000000000, -0.000000000000000000, 1.000000000000000000 ) ) ;
#6111=CARTESIAN_POINT ( 'NONE',  ( 6.358192987158592047, -4.248408730893246776, 1.257393750180309189 ) ) ;
#6112=CARTESIAN_POINT ( 'NONE',  ( -6.888301784570736608, -16.62983158437509346, -3.925737499819691223 ) ) ;
#6121=CARTESIAN_POINT ( 'NONE',  ( 3.580422610670021211, -18.00000000043041481, 6.520268750180309603 ) ) ;
#6127=CARTESIAN_POINT ( 'NONE',  ( 12.54593441764186679, 8.382925368423272516, 18.66361433151907079 ) ) ;
#6141=ORIENTED_EDGE ( 'NONE', *, *, #14421, .T. ) ;
#6142=AXIS2_PLACEMENT_3D ( 'NONE', #403, #15135, #7066 ) ;
#6144=LINE ( 'NONE', #12736, #20524 ) ;
#6148=CARTESIAN_POINT ( 'NONE',  ( 11.17563879704982632, -2.222972771497745637, -11.48785899935257504 ) ) ;
#6150=CARTESIAN_POINT ( 'NONE',  ( 2.870125741905211747, -6.929096494179675325, -26.13401249981968988 ) ) ;
#6158=CARTESIAN_POINT ( 'NONE',  ( -6.888301780572501976, 16.62983158603122291, -19.24136249981968660 ) ) ;
#6164=CARTESIAN_POINT ( 'NONE',  ( 0.000000000000000000, 0.000000000000000000, 40.00000000000000000 ) ) ;
#6173=CARTESIAN_POINT ( 'NONE',  ( -16.62983158603121936, -6.888301780572499311, -21.59761249981969300 ) ) ;
#6174=DIRECTION ( 'NONE',  ( -0.5000000000000037748, -0.8660254037844364872, 0.000000000000000000 ) ) ;
#6175=DIRECTION ( 'NONE',  ( 1.000000000000000000, 0.000000000000000000, 0.000000000000000000 ) ) ;
#6178=LINE ( 'NONE', #17746, #17456 ) ;
#6187=CARTESIAN_POINT ( 'NONE',  ( -17.99999999956958519, 3.580422614997674113, -18.80941874981969164 ) ) ;
#6202=DIRECTION ( 'NONE',  ( -0.000000000000000000, -0.000000000000000000, -1.000000000000000000 ) ) ;
#6203=CARTESIAN_POINT ( 'NONE',  ( -6.330490856366295382, 9.474249098604511587, 22.67776600064743064 ) ) ;
#6207=VERTEX_POINT ( 'NONE', #3581 ) ;
#6217=CARTESIAN_POINT ( 'NONE',  ( -7.500000000000000888, -3.289131931895657122E-15, 5.086300000002307087 ) ) ;
#6218=CARTESIAN_POINT ( 'NONE',  ( 2.163825119083639120E-09, 17.99999999999999645, -9.227299999819690512 ) ) ;
#6229=CARTESIAN_POINT ( 'NONE',  ( -3.580422614997675890, -17.99999999956958519, 7.109331250180310313 ) ) ;
#6236=CARTESIAN_POINT ( 'NONE',  ( 7.902369976724389566, -7.902369978624323110, -27.15198475028680392 ) ) ;
#6238=CIRCLE ( 'NONE', #3189, 2.650000000000000355 ) ;
#6241=CARTESIAN_POINT ( 'NONE',  ( -15.25966316918061771, 10.19618095414378622, -18.22035624981968738 ) ) ;
#6259=CARTESIAN_POINT ( 'NONE',  ( -10.32494394706616703, 4.276731815070943910, -6.480827749352571665 ) ) ;
#6261=CARTESIAN_POINT ( 'NONE',  ( -9.474249097082497073, 6.330490858644137298, 14.96598399971320070 ) ) ;
#6268=CARTESIAN_POINT ( 'NONE',  ( -12.72792206288791128, -12.72792205982779912, -12.76167499981968945 ) ) ;
#6273=CARTESIAN_POINT ( 'NONE',  ( 8.900000000000053646, 10.82531754730546147, 43.00000000000000000 ) ) ;
#6275=CARTESIAN_POINT ( 'NONE',  ( -2.870125743571141808, -6.929096493489625530, -6.105887499819693254 ) ) ;
#6277=CARTESIAN_POINT ( 'NONE',  ( 2.870125743571138255, 6.929096493489627306, -1.393387499819692010 ) ) ;
#6281=CARTESIAN_POINT ( 'NONE',  ( -3.580422614997674557, -17.99999999956957808, -23.07026874981969300 ) ) ;
#6283=CARTESIAN_POINT ( 'NONE',  ( 2.870125741905212635, -6.929096494179677101, 11.56598750018030941 ) ) ;
#6291=CARTESIAN_POINT ( 'NONE',  ( -15.15000000000000568, 3.245314017740485469E-16, 43.00000000000000000 ) ) ;
#6298=CARTESIAN_POINT ( 'NONE',  ( 17.50000000000000355, 2.143131898507868643E-15, 43.00000000000000000 ) ) ;
#6307=CARTESIAN_POINT ( 'NONE',  ( -10.32494394706616703, 4.276731815070943910, 21.79417225064743135 ) ) ;
#6315=CARTESIAN_POINT ( 'NONE',  ( -9.015947181032828388E-10, -7.500000000000002665, -25.54494999981969272 ) ) ;
#6318=CARTESIAN_POINT ( 'NONE',  ( -16.62983158437510056, 6.888301784570729502, 19.18511250018031333 ) ) ;
#6336=CARTESIAN_POINT ( 'NONE',  ( 18.00000000043041481, 3.580422610670020322, -5.260981249819691286 ) ) ;
#6341=CARTESIAN_POINT ( 'NONE',  ( 2.943691928843430450, 14.79893867722910095, -10.78951066848092921 ) ) ;
#6363=CARTESIAN_POINT ( 'NONE',  ( -10.32494394809439875, -4.276731812588566051, -17.08395274935258001 ) ) ;
#6365=CARTESIAN_POINT ( 'NONE',  ( 4.248408730893245888, 6.358192987158590270, -19.94885624981969485 ) ) ;
#6374=CARTESIAN_POINT ( 'NONE',  ( 3.580422614997668340, 17.99999999956958519, -18.35776874981969087 ) ) ;
#6407=CARTESIAN_POINT ( 'NONE',  ( 14.79893867758297610, -1.779016607511492805E-09, -12.53470808115845969 ) ) ;
#6430=CARTESIAN_POINT ( 'NONE',  ( 12.72792206288791128, 12.72792205982780267, -15.56957499981969484 ) ) ;
#6434=CARTESIAN_POINT ( 'NONE',  ( -14.79893867722910095, 2.943691928843434891, -13.14576066848092673 ) ) ;
#6439=CARTESIAN_POINT ( 'NONE',  ( -6.358192987158597376, 4.248408730893249441, 21.65979375018031661 ) ) ;
#6440=CARTESIAN_POINT ( 'NONE',  ( 6.250000000000054179, 10.82531754730546147, 43.00000000000000000 ) ) ;
#6445=CARTESIAN_POINT ( 'NONE',  ( 3.580422614997667896, 17.99999999956958163, 19.34223125018031197 ) ) ;
#6449=ORIENTED_EDGE ( 'NONE', *, *, #8651, .T. ) ;
#6457=CARTESIAN_POINT ( 'NONE',  ( 5.303300858261588147, -5.303300859536636658, 17.24182500018031661 ) ) ;
#6458=CARTESIAN_POINT ( 'NONE',  ( 10.32494394809438987, 4.276731812588564274, -0.6441722502868038047 ) ) ;
#6461=DIRECTION ( 'NONE',  ( -0.000000000000000000, -0.000000000000000000, 1.000000000000000000 ) ) ;
#6465=CARTESIAN_POINT ( 'NONE',  ( 17.99999999956958163, -3.580422614997676334, 14.17808125018031440 ) ) ;
#6472=CARTESIAN_POINT ( 'NONE',  ( -7.500000000000002665, -4.022542205827308438E-17, 14.51130000000230602 ) ) ;
#6483=CARTESIAN_POINT ( 'NONE',  ( -6.929096493489625530, 2.870125743571138255, 15.10036250018031367 ) ) ;
#6484=EDGE_CURVE ( 'NONE', #9398, #18276, #9512, .T. ) ;
#6485=CARTESIAN_POINT ( 'NONE',  ( -1.491842756249033286, -7.499999999820668783, -0.1355187498196866458 ) ) ;
#6492=CARTESIAN_POINT ( 'NONE',  ( -15.25966316918061771, 10.19618095414378622, 17.57504375018031695 ) ) ;
#6497=CARTESIAN_POINT ( 'NONE',  ( 0.000000000000000000, 0.000000000000000000, 40.00000000000000000 ) ) ;
#6498=ORIENTED_EDGE ( 'NONE', *, *, #18557, .T. ) ;
#6506=CARTESIAN_POINT ( 'NONE',  ( 11.17563879731705789, -1.343450868547281933E-09, 25.91760975064743278 ) ) ;
#6516=CARTESIAN_POINT ( 'NONE',  ( -10.19618095414378622, -15.25966316918061416, 17.12339375018031262 ) ) ;
#6528=CARTESIAN_POINT ( 'NONE',  ( 9.015937996181842420E-10, 7.500000000000007994, -5.142549999819685524 ) ) ;
#6534=CARTESIAN_POINT ( 'NONE',  ( -6.888301780572502864, 16.62983158603122646, -17.33676249981969164 ) ) ;
#6541=CARTESIAN_POINT ( 'NONE',  ( -8.382925368423267187, 12.54593441764186856, -2.542635668480925037 ) ) ;
#6553=CARTESIAN_POINT ( 'NONE',  ( -18.00000000043040771, -3.580422610670021211, 16.39691875018030842 ) ) ;
#6563=CARTESIAN_POINT ( 'NONE',  ( 6.358192988180019434, 4.248408729364581582, 15.18010625018031590 ) ) ;
#6565=CARTESIAN_POINT ( 'NONE',  ( -7.902369976724391343, 7.902369978624323110, 5.835515249713198571 ) ) ;
#6566=EDGE_CURVE ( 'NONE', #1433, #18811, #17402, .T. ) ;
#6573=CARTESIAN_POINT ( 'NONE',  ( 10.19618095414378800, 15.25966316918061416, 21.83589375018031831 ) ) ;
#6576=DIRECTION ( 'NONE',  ( -0.000000000000000000, -0.000000000000000000, 1.000000000000000000 ) ) ;
#6587=CARTESIAN_POINT ( 'NONE',  ( 5.303300859536630441, 5.303300858261584594, 8.620675000180311187 ) ) ;
#6592=ORIENTED_EDGE ( 'NONE', *, *, #20613, .T. ) ;
#6595=CARTESIAN_POINT ( 'NONE',  ( -18.00000000000000000, 2.163826221265758884E-09, 16.69145000018031411 ) ) ;
#6609=CARTESIAN_POINT ( 'NONE',  ( 6.330490858644141738, 9.474249097082498849, 24.44495350064742922 ) ) ;
#6637=CARTESIAN_POINT ( 'NONE',  ( -15.25966317163203456, -10.19618095047498230, -19.98754374981969661 ) ) ;
#6643=EDGE_CURVE ( 'NONE', #17243, #16003, #3297, .T. ) ;
#6646=CARTESIAN_POINT ( 'NONE',  ( 14.79893867793683349, 2.943691925285396582, -9.022323168480927080 ) ) ;
#6669=CARTESIAN_POINT ( 'NONE',  ( -1.491842754445842800, 7.500000000179346316, 22.83791875018031803 ) ) ;
#6670=CARTESIAN_POINT ( 'NONE',  ( 10.32494394809438987, 4.276731812588564274, 8.780827749713202124 ) ) ;
#6672=( BOUNDED_CURVE ( )  B_SPLINE_CURVE ( 2, ( #18908, #1212, #19002, #2684, #14349, #14034, #6277, #11054, #7765, #12764, #5960, #9559, #4589, #14236, #1528, #18797, #19215 ),
 .UNSPECIFIED., .F., .T. ) 
 B_SPLINE_CURVE_WITH_KNOTS ( ( 3, 2, 2, 2, 2, 2, 2, 2, 3 ),
 ( 0.4000000000038512193, 0.4125000000038511749, 0.4250000000038511860, 0.4375000000038511971, 0.4500000000038512082, 0.4625000000038511638, 0.4750000000038511194, 0.4875000000038511305, 0.5000000000038511416 ),
 .UNSPECIFIED. ) 
 CURVE ( )  GEOMETRIC_REPRESENTATION_ITEM ( )  RATIONAL_B_SPLINE_CURVE ( ( 0.9999999999940800688, 0.9807852804091503618, 1.000000000000000000, 0.9807852804032304306, 1.000000000000000000, 0.9807852804032304306, 1.000000000000000000, 0.9807852804032304306, 1.000000000000000000, 0.9807852804032304306, 1.000000000000000000, 0.9807852804032304306, 1.000000000000000000, 0.9807852804032304306, 1.000000000000000000, 0.9807852803973104994, 1.000000000005919931 ) ) 
 REPRESENTATION_ITEM ( '' )  );
#6679=CARTESIAN_POINT ( 'NONE',  ( 17.99999999956958163, -3.580422614997676334, -25.42651874981968874 ) ) ;
#6690=EDGE_CURVE ( 'NONE', #19935, #10395, #15137, .T. ) ;
#6692=SURFACE_SIDE_STYLE ('',( #13170 ) ) ;
#6704=FACE_OUTER_BOUND ( 'NONE', #1765, .T. ) ;
#6713=CARTESIAN_POINT ( 'NONE',  ( 4.925000000000044231, 8.530350227276702668, -43.00000000000000000 ) ) ;
#6715=CARTESIAN_POINT ( 'NONE',  ( 9.474249098604511587, 6.330490856366296271, 15.60901600064742922 ) ) ;
#6717=VERTEX_POINT ( 'NONE', #3754 ) ;
#6723=CARTESIAN_POINT ( 'NONE',  ( 12.72792205982779734, -12.72792206288791128, 15.06167500018031369 ) ) ;
#6736=CARTESIAN_POINT ( 'NONE',  ( -10.19618095414378800, -15.25966316918061771, -11.15160624981969306 ) ) ;
#6739=EDGE_CURVE ( 'NONE', #10849, #18811, #5357, .T. ) ;
#6743=CARTESIAN_POINT ( 'NONE',  ( -10.46442989202483709, 10.46442989454075168, -2.837166918480924949 ) ) ;
#6751=CARTESIAN_POINT ( 'NONE',  ( -4.248408729364577141, 6.358192988180014993, 15.98395625018030763 ) ) ;
#6767=CARTESIAN_POINT ( 'NONE',  ( 6.929096493489630859, -2.870125743571144472, 16.65276250018031590 ) ) ;
#6769=CARTESIAN_POINT ( 'NONE',  ( 11.17563879704981566, -2.222972771497744304, 9.664421499713199637 ) ) ;
#6776=CARTESIAN_POINT ( 'NONE',  ( 15.25966317163202746, 10.19618095047498407, 12.99995625018031475 ) ) ;
#6783=ORIENTED_EDGE ( 'NONE', *, *, #4341, .T. ) ;
#6789=CARTESIAN_POINT ( 'NONE',  ( 6.929096493489624642, -2.870125743571141363, 10.38786250018031154 ) ) ;
#6797=CARTESIAN_POINT ( 'NONE',  ( 1.491842756249030399, 7.499999999820669672, 4.576981250180313765 ) ) ;
#6799=CARTESIAN_POINT ( 'NONE',  ( -16.62983158437510056, 6.888301784570729502, 17.28051250018031482 ) ) ;
#6805=FACE_OUTER_BOUND ( 'NONE', #19252, .T. ) ;
#6810=CARTESIAN_POINT ( 'NONE',  ( -6.358192987158592047, 4.248408730893246776, -12.88010624981969166 ) ) ;
#6814=CARTESIAN_POINT ( 'NONE',  ( -11.17563879758428769, -2.222972768810840272, 2.060578500647426647 ) ) ;
#6819=LINE ( 'NONE', #14587, #1360 ) ;
#6823=CARTESIAN_POINT ( 'NONE',  ( -15.25966317163203279, -10.19618095047498052, 8.287456250180312622 ) ) ;
#6840=CARTESIAN_POINT ( 'NONE',  ( -12.54593441764187745, -8.382925368423274293, 19.56919816884154528 ) ) ;
#6844=CARTESIAN_POINT ( 'NONE',  ( 2.943691925285397470, -14.79893867793683349, -25.51607316848092921 ) ) ;
#6852=ADVANCED_FACE ( 'NONE', ( #16809 ), #2293, .T. ) ;
#6857=CARTESIAN_POINT ( 'NONE',  ( -3.580422614997674557, -17.99999999956957808, 14.62973125018030984 ) ) ;
#6866=CARTESIAN_POINT ( 'NONE',  ( 5.303300859536635770, 5.303300858261589923, -13.38942499981969014 ) ) ;
#6871=CARTESIAN_POINT ( 'NONE',  ( -7.500000000179346316, -1.491842754445844355, 20.48166875018031519 ) ) ;
#6872=CARTESIAN_POINT ( 'NONE',  ( -2.222972771497743416, -11.17563879704981566, 2.595671499713198660 ) ) ;
#6881=CARTESIAN_POINT ( 'NONE',  ( 10.19618095047497874, -15.25966317163203279, -12.91879374981968631 ) ) ;
#6896=VECTOR ( 'NONE', #20799, 1000.000000000000000 ) ;
#6897=FILL_AREA_STYLE_COLOUR ( '', #3318 ) ;
#6901=CARTESIAN_POINT ( 'NONE',  ( 6.929096494179676213, 2.870125741905210415, 9.209737500180313674 ) ) ;
#6908=CARTESIAN_POINT ( 'NONE',  ( -17.50000000000000355, 0.000000000000000000, 43.00000000000000000 ) ) ;
#6914=DIRECTION ( 'NONE',  ( 1.000000000000000000, 0.000000000000000000, -0.000000000000000000 ) ) ;
#6916=LINE ( 'NONE', #18261, #2389 ) ;
#6922=CARTESIAN_POINT ( 'NONE',  ( -17.99999999956958163, 3.580422614997673669, -11.28901874981968945 ) ) ;
#6926=CARTESIAN_POINT ( 'NONE',  ( 7.902369976724399336, -7.902369978624331104, 8.245734750647425670 ) ) ;
#6934=CARTESIAN_POINT ( 'NONE',  ( 3.580422614997668340, 17.99999999956958519, 11.82183125018031333 ) ) ;
#6949=CARTESIAN_POINT ( 'NONE',  ( -8.382925371439629458, -12.54593441562640876, 18.98013566884154812 ) ) ;
#6953=CARTESIAN_POINT ( 'NONE',  ( -5.663308646854335215, 13.67243654778934925, -21.09810441848092566 ) ) ;
#6964=CARTESIAN_POINT ( 'NONE',  ( 2.163825119083639120E-09, 17.99999999999999645, 0.1977000001803091989 ) ) ;
#6970=CARTESIAN_POINT ( 'NONE',  ( 6.250000000000054179, 10.82531754730546147, -43.00000000000000000 ) ) ;
#6975=CARTESIAN_POINT ( 'NONE',  ( 7.500000000000007994, -9.015933403756345817E-10, 6.638700000180315364 ) ) ;
#6977=CARTESIAN_POINT ( 'NONE',  ( 10.32494394809438987, 4.276731812588564274, -10.06917225028680463 ) ) ;
#6985=CARTESIAN_POINT ( 'NONE',  ( 6.888301784570728614, 16.62983158437510056, -6.733637499819689509 ) ) ;
#7005=CARTESIAN_POINT ( 'NONE',  ( -4.248408729364575365, 6.358192988180014105, -12.29104374981968739 ) ) ;
#7016=CARTESIAN_POINT ( 'NONE',  ( 16.62983158437509346, -6.888301784570739272, 12.56801250018031446 ) ) ;
#7018=VECTOR ( 'NONE', #7600, 1000.000000000000000 ) ;
#7020=DIRECTION ( 'NONE',  ( 0.000000000000000000, 0.000000000000000000, 1.000000000000000000 ) ) ;
#7022=CYLINDRICAL_SURFACE ( 'NONE', #11519, 2.649999999999999467 ) ;
#7023=CARTESIAN_POINT ( 'NONE',  ( -15.15000000000000568, 3.245314017740485469E-16, 43.00000000000000000 ) ) ;
#7026=( GEOMETRIC_REPRESENTATION_CONTEXT ( 3 ) GLOBAL_UNCERTAINTY_ASSIGNED_CONTEXT ( ( #2010 ) ) GLOBAL_UNIT_ASSIGNED_CONTEXT ( ( #11516, #506, #8541 ) ) REPRESENTATION_CONTEXT ( 'NONE', 'WORKASPACE' ) );
#7029=CARTESIAN_POINT ( 'NONE',  ( -3.580422614997674557, -17.99999999956957808, -4.220268749819692466 ) ) ;
#7033=CARTESIAN_POINT ( 'NONE',  ( -4.276731815070949239, -10.32494394706616347, 0.5879222506474277576 ) ) ;
#7040=CARTESIAN_POINT ( 'NONE',  ( -2.163827323447878234E-09, -18.00000000000000000, -2.610199999819689420 ) ) ;
#7048=VECTOR ( 'NONE', #17409, 1000.000000000000000 ) ;
#7052=CARTESIAN_POINT ( 'NONE',  ( -2.943691925285397470, 14.79893867793684059, 22.51451066884154528 ) ) ;
#7057=CARTESIAN_POINT ( 'NONE',  ( -10.46442989454075168, -10.46442989202483709, -24.04341691848093632 ) ) ;
#7066=DIRECTION ( 'NONE',  ( 1.000000000000000000, 0.000000000000000000, 0.000000000000000000 ) ) ;
#7067=CARTESIAN_POINT ( 'NONE',  ( 12.72792206288790773, 12.72792205982779912, 10.80082500018031055 ) ) ;
#7074=CARTESIAN_POINT ( 'NONE',  ( 4.248408730893249441, 6.358192987158596488, -13.68395624981969050 ) ) ;
#7077=CARTESIAN_POINT ( 'NONE',  ( 4.248408729364579806, -6.358192988180021210, 8.111356250180314476 ) ) ;
#7079=CARTESIAN_POINT ( 'NONE',  ( 1.343451552857795099E-09, 11.17563879731704723, -21.26135975028680036 ) ) ;
#7084=CARTESIAN_POINT ( 'NONE',  ( -2.163827323447878234E-09, -18.00000000000000000, -2.610199999819689420 ) ) ;
#7100=CARTESIAN_POINT ( 'NONE',  ( -7.500000000179339210, -1.491842754445842800, -14.05823124981969130 ) ) ;
#7105=DIRECTION ( 'NONE',  ( -0.5000000000000037748, -0.8660254037844364872, 0.000000000000000000 ) ) ;
#7107=CARTESIAN_POINT ( 'NONE',  ( -6.929096493489632635, 2.870125743571140919, 2.515262500180314387 ) ) ;
#7109=CARTESIAN_POINT ( 'NONE',  ( -18.00000000000000000, 2.163826221265758884E-09, -2.158549999819688203 ) ) ;
#7122=CARTESIAN_POINT ( 'NONE',  ( 7.500000000000004441, 1.491842754878798027, -9.345731249912210714 ) ) ;
#7123=CARTESIAN_POINT ( 'NONE',  ( 17.99999999956957808, -3.580422614997675446, -16.00151874981969158 ) ) ;
#7127=CARTESIAN_POINT ( 'NONE',  ( -11.17563879731705789, 1.343452237168309506E-09, 11.78010975064742816 ) ) ;
#7129=PLANE ( 'NONE',  #15588 ) ;
#7133=CARTESIAN_POINT ( 'NONE',  ( -3.580422614997675002, -17.99999999956958163, 7.109331250180313866 ) ) ;
#7136=VERTEX_POINT ( 'NONE', #6713 ) ;
#7152=CARTESIAN_POINT ( 'NONE',  ( -2.943691928843437999, -14.79893867722910450, 8.966073168841550256 ) ) ;
#7155=ORIENTED_EDGE ( 'NONE', *, *, #15116, .F. ) ;
#7160=CARTESIAN_POINT ( 'NONE',  ( 10.46442989454075168, 10.46442989202483886, -19.33091691848093419 ) ) ;
#7170=CIRCLE ( 'NONE', #19038, 7.500000000000000000 ) ;
#7173=CARTESIAN_POINT ( 'NONE',  ( -18.00000000043040771, -3.580422610670021211, -2.453081249819692111 ) ) ;
#7180=CARTESIAN_POINT ( 'NONE',  ( -6.888301780572502864, 16.62983158603122646, 20.36323750018031120 ) ) ;
#7183=CARTESIAN_POINT ( 'NONE',  ( 7.500000000179346316, 1.491842754445843244, 6.344168750180314120 ) ) ;
#7185=CARTESIAN_POINT ( 'NONE',  ( 6.929096493489630859, -2.870125743571144472, 16.65276250018031590 ) ) ;
#7186=CARTESIAN_POINT ( 'NONE',  ( 4.276731812588566939, -10.32494394809438809, -7.712922250286803560 ) ) ;
#7191=CARTESIAN_POINT ( 'NONE',  ( 2.163825119083639534E-09, 18.00000000000000000, -7.322699999819687555 ) ) ;
#7207=CARTESIAN_POINT ( 'NONE',  ( 5.303300858261582817, -5.303300859536631329, 1.551925000180309766 ) ) ;
#7210=EDGE_CURVE ( 'NONE', #10849, #16910, #3814, .T. ) ;
#7215=ORIENTED_EDGE ( 'NONE', *, *, #16745, .T. ) ;
#7218=CARTESIAN_POINT ( 'NONE',  ( 2.163825119083639534E-09, 18.00000000000000000, 0.1977000001803126683 ) ) ;
#7229=CARTESIAN_POINT ( 'NONE',  ( -6.888301780572500199, 16.62983158603121936, -9.816362499819691223 ) ) ;
#7234=CARTESIAN_POINT ( 'NONE',  ( -2.222972768810837607, 11.17563879758428769, -14.43317149935257326 ) ) ;
#7244=CARTESIAN_POINT ( 'NONE',  ( 16.62983158603122291, 6.888301780572502864, 13.29448750018031511 ) ) ;
#7259=CARTESIAN_POINT ( 'NONE',  ( -12.54593441562641054, 8.382925371439629458, 11.91138566884154848 ) ) ;
#7266=EDGE_CURVE ( 'NONE', #11708, #19185, #16779, .T. ) ;
#7267=CARTESIAN_POINT ( 'NONE',  ( -10.46442989202483709, 10.46442989454075168, -21.68716691848092992 ) ) ;
#7280=CARTESIAN_POINT ( 'NONE',  ( -16.62983158603121936, -6.888301780572499311, -2.747612499819688914 ) ) ;
#7288=CARTESIAN_POINT ( 'NONE',  ( -16.62983158603122646, -6.888301780572501976, 18.00698750018030836 ) ) ;
#7294=CARTESIAN_POINT ( 'NONE',  ( -4.248408730893249441, -6.358192987158595599, 0.4535437501803143978 ) ) ;
#7297=CARTESIAN_POINT ( 'NONE',  ( 2.222972771497739419, 11.17563879704981922, -11.54182850028680640 ) ) ;
#7302=FACE_OUTER_BOUND ( 'NONE', #11821, .T. ) ;
#7303=CARTESIAN_POINT ( 'NONE',  ( -3.580422614997675002, -17.99999999956958163, -11.74066874981969200 ) ) ;
#7318=CARTESIAN_POINT ( 'NONE',  ( 1.491842756249028845, 7.499999999820661678, -11.11291874981969308 ) ) ;
#7329=CARTESIAN_POINT ( 'NONE',  ( -12.72792206288791128, -12.72792205982779912, 6.088325000180314639 ) ) ;
#7335=DIRECTION ( 'NONE',  ( 0.000000000000000000, 0.000000000000000000, -1.000000000000000000 ) ) ;
#7343=CARTESIAN_POINT ( 'NONE',  ( 16.62983158437509346, -6.888301784570737496, -15.70698749981969122 ) ) ;
#7347=CARTESIAN_POINT ( 'NONE',  ( 3.599999999999902833, -10.82531754730554496, 40.00000000000000000 ) ) ;
#7348=CARTESIAN_POINT ( 'NONE',  ( -11.17563879731705789, 1.343452237168309506E-09, -7.069890249352571487 ) ) ;
#7356=CARTESIAN_POINT ( 'NONE',  ( 15.25966317163202746, 10.19618095047498407, -5.850043749819688443 ) ) ;
#7370=CARTESIAN_POINT ( 'NONE',  ( -8.382925371439629458, -12.54593441562640876, 0.1301356688415446494 ) ) ;
#7374=ADVANCED_FACE ( 'NONE', ( #15825 ), #7768, .F. ) ;
#7376=CARTESIAN_POINT ( 'NONE',  ( 6.888301780572505528, -16.62983158603121581, 13.74613750018031233 ) ) ;
#7386=CARTESIAN_POINT ( 'NONE',  ( -16.62983158437509701, 6.888301784570728614, -20.41948749981969158 ) ) ;
#7396=CARTESIAN_POINT ( 'NONE',  ( 18.00000000000000355, -2.163824016901520597E-09, 13.88355000018031049 ) ) ;
#7398=CARTESIAN_POINT ( 'NONE',  ( -7.499999999820669672, 1.491842756249032620, 2.220731250180314476 ) ) ;
#7402=CARTESIAN_POINT ( 'NONE',  ( -5.303300859536636658, -5.303300858261589035, 19.59807500018031590 ) ) ;
#7403=CARTESIAN_POINT ( 'NONE',  ( 8.382925371439627682, 12.54593441562639988, 18.07455183151907363 ) ) ;
#7406=CARTESIAN_POINT ( 'NONE',  ( 7.500000000000000000, 9.184850993605147944E-16, 40.00000000000000000 ) ) ;
#7407=CARTESIAN_POINT ( 'NONE',  ( 10.19618095414378800, 15.25966316918061416, -15.86410624981969342 ) ) ;
#7422=CYLINDRICAL_SURFACE ( 'NONE', #4097, 17.50000000000000355 ) ;
#7423=CARTESIAN_POINT ( 'NONE',  ( -6.358192988180014993, -4.248408729364575365, -5.222293749819688635 ) ) ;
#7426=DIRECTION ( 'NONE',  ( -0.1159034202170342726, 1.393303357259140646E-11, -0.9932604880805404601 ) ) ;
#7432=CARTESIAN_POINT ( 'NONE',  ( -12.72792205982779912, 12.72792206288790950, 8.444575000180313040 ) ) ;
#7441=ORIENTED_EDGE ( 'NONE', *, *, #1986, .T. ) ;
#7442=CARTESIAN_POINT ( 'NONE',  ( 4.248408729364579806, -6.358192988180021210, -20.16364374981968766 ) ) ;
#7446=ADVANCED_BREP_SHAPE_REPRESENTATION ( '', ( #10096, #12461 ), #7026 ) ;
#7448=DIRECTION ( 'NONE',  ( 1.000000000000000000, 0.000000000000000000, 0.000000000000000000 ) ) ;
#7456=CARTESIAN_POINT ( 'NONE',  ( -12.72792205982779912, 12.72792206288790950, -17.92582499981968880 ) ) ;
#7463=CIRCLE ( 'NONE', #357, 2.649999999999999467 ) ;
#7471=CARTESIAN_POINT ( 'NONE',  ( -5.663308650141539502, -13.67243654642775574, -0.1643955811584559001 ) ) ;
#7478=CARTESIAN_POINT ( 'NONE',  ( 3.580422614997667896, 17.99999999956958163, 9.917231250180309488 ) ) ;
#7488=CARTESIAN_POINT ( 'NONE',  ( -10.19618095414378445, -15.25966316918061239, -3.631206249819690868 ) ) ;
#7489=EDGE_LOOP ( 'NONE', ( #9666, #20715 ) ) ;
#7491=DIRECTION ( 'NONE',  ( -0.000000000000000000, -0.000000000000000000, -1.000000000000000000 ) ) ;
#7492=( GEOMETRIC_REPRESENTATION_CONTEXT ( 3 ) GLOBAL_UNCERTAINTY_ASSIGNED_CONTEXT ( ( #955 ) ) GLOBAL_UNIT_ASSIGNED_CONTEXT ( ( #18012, #7962, #16122 ) ) REPRESENTATION_CONTEXT ( 'NONE', 'WORKASPACE' ) );
#7499=CARTESIAN_POINT ( 'NONE',  ( 16.62983158603122646, 6.888301780572504640, 13.29448750018031156 ) ) ;
#7503=CARTESIAN_POINT ( 'NONE',  ( -8.382925371439625906, -12.54593441562639988, 13.36205183151907505 ) ) ;
#7510=CARTESIAN_POINT ( 'NONE',  ( 6.888301780572507305, -16.62983158603121936, -22.04926249981969022 ) ) ;
#7515=ORIENTED_EDGE ( 'NONE', *, *, #6739, .F. ) ;
#7519=EDGE_CURVE ( 'NONE', #16575, #20492, #9027, .T. ) ;
#7529=CARTESIAN_POINT ( 'NONE',  ( -11.17563879758427525, -2.222972768810838051, 13.78785899971320106 ) ) ;
#7539=CARTESIAN_POINT ( 'NONE',  ( 18.00000000000000000, -2.163824016901520184E-09, -6.871049999819685894 ) ) ;
#7547=CARTESIAN_POINT ( 'NONE',  ( 6.929096493489625530, -2.870125743571142252, -8.462137499819693431 ) ) ;
#7555=CARTESIAN_POINT ( 'NONE',  ( -12.50000000000000533, 0.000000000000000000, 40.00000000000000000 ) ) ;
#7569=CARTESIAN_POINT ( 'NONE',  ( -6.888301784570738384, -16.62983158437509346, -20.87113749981968880 ) ) ;
#7571=DIRECTION ( 'NONE',  ( 1.000000000000000000, 0.000000000000000000, 0.000000000000000000 ) ) ;
#7573=ORIENTED_EDGE ( 'NONE', *, *, #4933, .F. ) ;
#7576=CARTESIAN_POINT ( 'NONE',  ( 7.500000000000004441, -8.788009009181406898E-15, -18.47619999999769647 ) ) ;
#7588=CARTESIAN_POINT ( 'NONE',  ( 14.79893867722910450, -2.943691928843438443, 6.609823168841544749 ) ) ;
#7594=CARTESIAN_POINT ( 'NONE',  ( 10.19618095414378622, 15.25966316918061239, 10.50629375018031020 ) ) ;
#7596=CARTESIAN_POINT ( 'NONE',  ( 6.929096494179677990, 2.870125741905210859, -19.06526249981969556 ) ) ;
#7600=DIRECTION ( 'NONE',  ( -0.000000000000000000, -0.000000000000000000, -1.000000000000000000 ) ) ;
#7605=CARTESIAN_POINT ( 'NONE',  ( 12.72792206288790773, 12.72792205982779912, -8.049174999819690868 ) ) ;
#7608=CARTESIAN_POINT ( 'NONE',  ( -5.303300859536636658, -5.303300858261589035, -8.676924999819688011 ) ) ;
#7610=FACE_BOUND ( 'NONE', #12126, .T. ) ;
#7613=CARTESIAN_POINT ( 'NONE',  ( -18.00000000000000355, 2.163826221265759298E-09, -0.2539499998196921293 ) ) ;
#7614=CARTESIAN_POINT ( 'NONE',  ( -1.491842756249033064, -7.499999999820668783, -18.98551874981968268 ) ) ;
#7618=CARTESIAN_POINT ( 'NONE',  ( -2.943691928843435779, -14.79893867722909917, 12.77298933151907612 ) ) ;
#7640=FILL_AREA_STYLE_COLOUR ( '', #10207 ) ;
#7641=CARTESIAN_POINT ( 'NONE',  ( 6.929096493489624642, -2.870125743571141363, -27.31213749981969130 ) ) ;
#7645=EDGE_CURVE ( 'NONE', #1438, #3529, #523, .T. ) ;
#7649=CARTESIAN_POINT ( 'NONE',  ( 10.19618095047497874, -15.25966317163203279, -24.24839374981968732 ) ) ;
#7656=DIRECTION ( 'NONE',  ( -0.000000000000000000, -0.000000000000000000, -1.000000000000000000 ) ) ;
#7657=FACE_OUTER_BOUND ( 'NONE', #11930, .T. ) ;
#7681=CARTESIAN_POINT ( 'NONE',  ( 10.19618095414378800, 15.25966316918061416, -6.439106249819689154 ) ) ;
#7682=VECTOR ( 'NONE', #20794, 1000.000000000000000 ) ;
#7700=CARTESIAN_POINT ( 'NONE',  ( -12.54593441562641054, 8.382925371439629458, -6.938614331158453830 ) ) ;
#7708=CARTESIAN_POINT ( 'NONE',  ( -6.888301784570736608, -16.62983158437509346, 14.92426250018031020 ) ) ;
#7713=CARTESIAN_POINT ( 'NONE',  ( 6.250000000000054179, 10.82531754730546147, 43.00000000000000000 ) ) ;
#7719=CARTESIAN_POINT ( 'NONE',  ( 10.19618095414378622, 15.25966316918061239, -17.76870624981969371 ) ) ;
#7721=VERTEX_POINT ( 'NONE', #15460 ) ;
#7727=CARTESIAN_POINT ( 'NONE',  ( -2.163827323447878648E-09, -18.00000000000000355, -2.610199999819692973 ) ) ;
#7731=CARTESIAN_POINT ( 'NONE',  ( -10.46442989202483709, 10.46442989454075168, 16.01283308151908003 ) ) ;
#7735=CARTESIAN_POINT ( 'NONE',  ( 3.580422614997668340, 17.99999999956958519, -16.45316874981969235 ) ) ;
#7736=DIRECTION ( 'NONE',  ( 0.000000000000000000, 0.000000000000000000, -1.000000000000000000 ) ) ;
#7748=CARTESIAN_POINT ( 'NONE',  ( 7.902369976724399336, -7.902369978624331104, -1.179265249352571931 ) ) ;
#7749=CARTESIAN_POINT ( 'NONE',  ( -9.015947181032828388E-10, -7.500000000000000888, -16.11994999981969556 ) ) ;
#7757=CARTESIAN_POINT ( 'NONE',  ( 18.00000000043041126, 3.580422610670019434, -16.59058124981968874 ) ) ;
#7759=ORIENTED_EDGE ( 'NONE', *, *, #8645, .F. ) ;
#7763=CARTESIAN_POINT ( 'NONE',  ( -1.491842756249031954, -7.499999999820663454, -6.400418749819693609 ) ) ;
#7764=CARTESIAN_POINT ( 'NONE',  ( 4.924999999999924327, -8.530350227276771946, -40.00000000000000000 ) ) ;
#7765=CARTESIAN_POINT ( 'NONE',  ( 9.015937996181835182E-10, 7.500000000000002665, -1.982449999819692943 ) ) ;
#7768=CYLINDRICAL_SURFACE ( 'NONE', #1911, 2.649999999999999467 ) ;
#7769=CARTESIAN_POINT ( 'NONE',  ( 17.99999999956957808, -3.580422614997675446, -25.42651874981969229 ) ) ;
#7771=CARTESIAN_POINT ( 'NONE',  ( -1.491842756249031954, -7.499999999820663454, 12.44958125018030870 ) ) ;
#7774=DIRECTION ( 'NONE',  ( 1.000000000000000000, 0.000000000000000000, 0.000000000000000000 ) ) ;
#7777=CARTESIAN_POINT ( 'NONE',  ( -6.929096493489632635, 2.870125743571140919, -6.909737499819684992 ) ) ;
#7780=CARTESIAN_POINT ( 'NONE',  ( -10.19618095047498052, 15.25966317163203101, -8.206293749819685956 ) ) ;
#7785=DIRECTION ( 'NONE',  ( -1.202124453834178598E-10, -1.000000000000000000, 1.727264247904875625E-25 ) ) ;
#7794=CARTESIAN_POINT ( 'NONE',  ( -10.46442989202484242, 10.46442989454075700, -16.06908308115845685 ) ) ;
#7796=CARTESIAN_POINT ( 'NONE',  ( -2.870125743571141808, -6.929096493489625530, -15.53088749981969663 ) ) ;
#7800=ADVANCED_FACE ( 'NONE', ( #4333, #2841, #7610, #15771 ), #9308, .T. ) ;
#7805=ADVANCED_FACE ( 'NONE', ( #15875 ), #4428, .T. ) ;
#7813=CARTESIAN_POINT ( 'NONE',  ( -6.888301784570736608, -16.62983158437509346, -13.35073749981969371 ) ) ;
#7820=CARTESIAN_POINT ( 'NONE',  ( -6.888301780572502864, 16.62983158603122646, 10.93823750018031049 ) ) ;
#7821=CARTESIAN_POINT ( 'NONE',  ( 1.491842754445843688, -7.500000000179346316, -19.57458124981968695 ) ) ;
#7826=CARTESIAN_POINT ( 'NONE',  ( 13.67243654642774686, -5.663308650141536837, 10.71127058151907718 ) ) ;
#7830=CARTESIAN_POINT ( 'NONE',  ( 15.25966316918061416, -10.19618095414378622, -22.93285624981968951 ) ) ;
#7832=VERTEX_POINT ( 'NONE', #14197 ) ;
#7848=CARTESIAN_POINT ( 'NONE',  ( 6.330490858644141738, 9.474249097082498849, -3.830046499352573797 ) ) ;
#7851=CARTESIAN_POINT ( 'NONE',  ( -4.248408730893245000, -6.358192987158590270, -24.66135624981969698 ) ) ;
#7859=CARTESIAN_POINT ( 'NONE',  ( -18.00000000043041126, -3.580422610670022543, -11.87808124981968838 ) ) ;
#7866=CARTESIAN_POINT ( 'NONE',  ( 8.899999999999900879, -10.82531754730554496, 43.00000000000000000 ) ) ;
#7899=CARTESIAN_POINT ( 'NONE',  ( -9.850000000000006750, 0.000000000000000000, 40.00000000000000000 ) ) ;
#7902=CARTESIAN_POINT ( 'NONE',  ( -14.79893867722910628, 2.943691928843437111, -16.95267683115846324 ) ) ;
#7908=FACE_BOUND ( 'NONE', #13315, .T. ) ;
#7910=CARTESIAN_POINT ( 'NONE',  ( -6.929096494179678878, -2.870125741905209971, -23.77776249981969769 ) ) ;
#7924=ORIENTED_EDGE ( 'NONE', *, *, #9370, .T. ) ;
#7929=DIRECTION ( 'NONE',  ( -0.000000000000000000, -0.000000000000000000, 1.000000000000000000 ) ) ;
#7931=CARTESIAN_POINT ( 'NONE',  ( 18.00000000000000355, -2.163824016901520597E-09, -14.39144999981969342 ) ) ;
#7936=CARTESIAN_POINT ( 'NONE',  ( -2.870125743571144028, -6.929096493489630859, -18.69098749981968410 ) ) ;
#7938=CARTESIAN_POINT ( 'NONE',  ( 14.79893867758296544, -1.779016607511491977E-09, -8.727791918480926725 ) ) ;
#7940=EDGE_CURVE ( 'NONE', #1354, #9669, #733, .T. ) ;
#7962=( NAMED_UNIT ( * ) PLANE_ANGLE_UNIT ( ) SI_UNIT ( $, .RADIAN. ) );
#7963=CARTESIAN_POINT ( 'NONE',  ( 6.330490858644141738, 9.474249097082498849, -13.25504649935257895 ) ) ;
#7964=CARTESIAN_POINT ( 'NONE',  ( 7.902369978624323110, 7.902369976724394895, 17.61676524971320390 ) ) ;
#7971=CARTESIAN_POINT ( 'NONE',  ( 16.62983158437509346, -6.888301784570739272, -6.281987499819688736 ) ) ;
#7977=CARTESIAN_POINT ( 'NONE',  ( 5.303300858261583706, -5.303300859536632217, -7.873074999819692721 ) ) ;
#7978=LINE ( 'NONE', #12654, #12805 ) ;
#7989=CARTESIAN_POINT ( 'NONE',  ( -6.358192988180021210, -4.248408729364580694, 1.042606250180315497 ) ) ;
#8009=CARTESIAN_POINT ( 'NONE',  ( -13.67243654778936168, -5.663308646854336992, -17.83627058115845898 ) ) ;
#8011=CARTESIAN_POINT ( 'NONE',  ( -5.303300859536632217, -5.303300858261584594, -14.94182499981969592 ) ) ;
#8037=CARTESIAN_POINT ( 'NONE',  ( 18.00000000043041481, 3.580422610670020322, -14.68598124981969377 ) ) ;
#8044=CARTESIAN_POINT ( 'NONE',  ( 2.943691928843430450, 14.79893867722910095, -1.364510668480926281 ) ) ;
#8050=CARTESIAN_POINT ( 'NONE',  ( -1.491842754445842800, 7.500000000179346316, 22.83791875018031448 ) ) ;
#8056=ORIENTED_EDGE ( 'NONE', *, *, #19310, .T. ) ;
#8068=CARTESIAN_POINT ( 'NONE',  ( 10.32494394706616347, -4.276731815070950127, -20.61832774935258072 ) ) ;
#8069=CARTESIAN_POINT ( 'NONE',  ( 7.902369978624323110, 7.902369976724394895, 8.191765249713197861 ) ) ;
#8078=CARTESIAN_POINT ( 'NONE',  ( -16.62983158437510056, 6.888301784570729502, 19.18511250018031333 ) ) ;
#8088=CYLINDRICAL_SURFACE ( 'NONE', #556, 7.500000000000000000 ) ;
#8093=CARTESIAN_POINT ( 'NONE',  ( -1.491842754445841246, 7.500000000179339210, 16.57301875018031012 ) ) ;
#8100=CARTESIAN_POINT ( 'NONE',  ( -12.72792205982779912, 12.72792206288790950, 17.86957500018031553 ) ) ;
#8109=CARTESIAN_POINT ( 'NONE',  ( -7.500000000000007994, -4.022542210876018231E-17, 20.77620000000231570 ) ) ;
#8110=CARTESIAN_POINT ( 'NONE',  ( -8.382925368423274293, 12.54593441764187745, -15.77455183115845649 ) ) ;
#8111=ORIENTED_EDGE ( 'NONE', *, *, #11938, .F. ) ;
#8113=CARTESIAN_POINT ( 'NONE',  ( 3.599999999999902389, -10.82531754730554496, 43.00000000000000000 ) ) ;
#8116=CARTESIAN_POINT ( 'NONE',  ( -16.62983158603122291, -6.888301780572501087, 18.00698750018031546 ) ) ;
#8124=DIRECTION ( 'NONE',  ( -1.000000000000000000, 0.000000000000000000, 0.000000000000000000 ) ) ;
#8130=CARTESIAN_POINT ( 'NONE',  ( 17.99999999956958519, -3.580422614997676778, -14.09691874981969129 ) ) ;
#8135=CARTESIAN_POINT ( 'NONE',  ( 5.663308650141530620, 13.67243654642775041, -1.069979418480925926 ) ) ;
#8156=CARTESIAN_POINT ( 'NONE',  ( 11.17563879731705789, -1.343450868547281933E-09, -21.20739024935257788 ) ) ;
#8158=CARTESIAN_POINT ( 'NONE',  ( -4.276731812588563386, 10.32494394809438987, -3.000422250286804093 ) ) ;
#8166=CARTESIAN_POINT ( 'NONE',  ( 16.62983158437509346, -6.888301784570739272, -25.13198749981969016 ) ) ;
#8182=CARTESIAN_POINT ( 'NONE',  ( -7.500000000000007105, -3.289131931996631318E-15, 11.35120000000231677 ) ) ;
#8187=ADVANCED_FACE ( 'NONE', ( #18117 ), #19308, .F. ) ;
#8192=ORIENTED_EDGE ( 'NONE', *, *, #10651, .F. ) ;
#8205=CARTESIAN_POINT ( 'NONE',  ( 8.382925368423272516, -12.54593441764187745, -11.06205183115845614 ) ) ;
#8208=VERTEX_POINT ( 'NONE', #8457 ) ;
#8215=CARTESIAN_POINT ( 'NONE',  ( 18.00000000000000000, -2.163824016901520184E-09, 23.30855000018031475 ) ) ;
#8232=CARTESIAN_POINT ( 'NONE',  ( -6.888301784570739272, -16.62983158437509701, -11.44613749981969519 ) ) ;
#8238=CARTESIAN_POINT ( 'NONE',  ( -10.46442989454075168, -10.46442989202483709, -5.193416918480926903 ) ) ;
#8261=CARTESIAN_POINT ( 'NONE',  ( -6.929096494179684207, -2.870125741905212635, 20.18713750018031305 ) ) ;
#8264=CARTESIAN_POINT ( 'NONE',  ( -10.32494394809439164, -4.276731812588563386, -5.356672250286801606 ) ) ;
#8270=CARTESIAN_POINT ( 'NONE',  ( 6.888301784570728614, 16.62983158437510056, 12.11636250018031369 ) ) ;
#8285=EDGE_CURVE ( 'NONE', #1316, #7136, #20025, .T. ) ;
#8287=CARTESIAN_POINT ( 'NONE',  ( -4.248408730893245000, -6.358192987158590270, 3.613643750180311809 ) ) ;
#8299=DIRECTION ( 'NONE',  ( -0.000000000000000000, -0.000000000000000000, -1.000000000000000000 ) ) ;
#8302=DIRECTION ( 'NONE',  ( -0.000000000000000000, -0.000000000000000000, -1.000000000000000000 ) ) ;
#8310=CARTESIAN_POINT ( 'NONE',  ( 2.222972768810839383, -11.17563879758428769, 9.129328500647432065 ) ) ;
#8317=EDGE_LOOP ( 'NONE', ( #10971, #626, #11788, #16289, #20566, #17794, #9570, #11481, #9047, #3602, #3935, #13858, #14448 ) ) ;
#8320=DIRECTION ( 'NONE',  ( -1.000000000000000000, 1.202124453834178339E-10, 0.000000000000000000 ) ) ;
#8332=CARTESIAN_POINT ( 'NONE',  ( 6.929096493489630859, -2.870125743571144472, -11.62223749981968624 ) ) ;
#8336=CARTESIAN_POINT ( 'NONE',  ( 16.62983158603122646, 6.888301780572504640, -14.98051249981969413 ) ) ;
#8343=VECTOR ( 'NONE', #8632, 1000.000000000000000 ) ;
#8344=CARTESIAN_POINT ( 'NONE',  ( 13.67243654642774686, -5.663308650141536837, 1.286270581519075362 ) ) ;
#8353=ORIENTED_EDGE ( 'NONE', *, *, #8639, .F. ) ;
#8358=ORIENTED_EDGE ( 'NONE', *, *, #13166, .F. ) ;
#8360=AXIS2_PLACEMENT_3D ( 'NONE', #7713, #6106, #20726 ) ;
#8368=SURFACE_STYLE_USAGE ( .BOTH. , #3187 ) ;
#8369=CARTESIAN_POINT ( 'NONE',  ( -9.015947181032835626E-10, -7.500000000000007994, 18.41995000018031803 ) ) ;
#8371=CARTESIAN_POINT ( 'NONE',  ( 4.276731812588566939, -10.32494394809438809, 1.712077749713197372 ) ) ;
#8372=CARTESIAN_POINT ( 'NONE',  ( 0.000000000000000000, 0.000000000000000000, 40.00000000000000000 ) ) ;
#8376=CARTESIAN_POINT ( 'NONE',  ( -3.580422610670018546, 18.00000000043041126, 11.23276875018031440 ) ) ;
#8391=CARTESIAN_POINT ( 'NONE',  ( -5.303300858261583706, 5.303300859536630441, 15.68942500018031438 ) ) ;
#8399=ORIENTED_EDGE ( 'NONE', *, *, #19895, .T. ) ;
#8400=CARTESIAN_POINT ( 'NONE',  ( 3.580422614997668340, 17.99999999956958519, 19.34223125018031553 ) ) ;
#8411=CARTESIAN_POINT ( 'NONE',  ( 2.222972771497741640, 11.17563879704982988, 14.43089100064742958 ) ) ;
#8415=VERTEX_POINT ( 'NONE', #2536 ) ;
#8432=CARTESIAN_POINT ( 'NONE',  ( 12.54593441764187567, 8.382925368423276069, 24.28169816884155097 ) ) ;
#8440=CARTESIAN_POINT ( 'NONE',  ( 14.79893867722909917, -2.943691928843437111, -17.85826066848093063 ) ) ;
#8452=CARTESIAN_POINT ( 'NONE',  ( -12.72792205982779556, 12.72792206288790773, -0.9804249998196894467 ) ) ;
#8457=CARTESIAN_POINT ( 'NONE',  ( -17.50000000000000355, 0.000000000000000000, 40.00000000000000000 ) ) ;
#8458=CARTESIAN_POINT ( 'NONE',  ( -6.888301784570739272, -16.62983158437509701, 16.82886250018031049 ) ) ;
#8461=CARTESIAN_POINT ( 'NONE',  ( -7.500000000000007994, 9.015942588607339023E-10, 20.77620000018031732 ) ) ;
#8462=CARTESIAN_POINT ( 'NONE',  ( 11.17563879758427525, 2.222972768810836719, 9.075358999713197150 ) ) ;
#8468=CARTESIAN_POINT ( 'NONE',  ( 15.25966316918061416, -10.19618095414378622, -24.83745624981969158 ) ) ;
#8473=CIRCLE ( 'NONE', #2737, 2.650000000000000355 ) ;
#8474=CARTESIAN_POINT ( 'NONE',  ( 0.000000000000000000, 0.000000000000000000, 40.00000000000000000 ) ) ;
#8483=CARTESIAN_POINT ( 'NONE',  ( -7.500000000179339210, -1.491842754445842800, 4.791768750180311898 ) ) ;
#8507=CARTESIAN_POINT ( 'NONE',  ( 17.99999999999999645, -2.163824016901520184E-09, -6.871049999819689447 ) ) ;
#8510=CARTESIAN_POINT ( 'NONE',  ( 11.17563879731705789, -1.343450868547281933E-09, 7.067609750647429578 ) ) ;
#8519=CARTESIAN_POINT ( 'NONE',  ( 16.62983158603122291, 6.888301780572502864, 3.869487500180311734 ) ) ;
#8536=CARTESIAN_POINT ( 'NONE',  ( 2.943691925285398803, -14.79893867793684059, 17.80201066884154315 ) ) ;
#8541=( NAMED_UNIT ( * ) SI_UNIT ( $, .STERADIAN. ) SOLID_ANGLE_UNIT ( ) );
#8542=CARTESIAN_POINT ( 'NONE',  ( -1.779019326032424095E-09, -14.79893867758296544, -15.79654191848093525 ) ) ;
#8544=AXIS2_PLACEMENT_3D ( 'NONE', #19243, #3126, #12889 ) ;
#8556=CARTESIAN_POINT ( 'NONE',  ( 15.25966316918061239, -10.19618095414378445, 3.437543750180311442 ) ) ;
#8565=CARTESIAN_POINT ( 'NONE',  ( 2.163825119083639947E-09, 18.00000000000000355, 20.95230000018031191 ) ) ;
#8566=CIRCLE ( 'NONE', #16348, 2.650000000000000355 ) ;
#8571=CARTESIAN_POINT ( 'NONE',  ( 6.358192988180019434, 4.248408729364581582, 5.755106250180314298 ) ) ;
#8572=CARTESIAN_POINT ( 'NONE',  ( -11.17563879704981922, 2.222972771497742972, -13.89807850028680392 ) ) ;
#8579=DIRECTION ( 'NONE',  ( -0.000000000000000000, -0.000000000000000000, 1.000000000000000000 ) ) ;
#8580=CARTESIAN_POINT ( 'NONE',  ( -18.00000000000000000, 2.163826221265758884E-09, -0.2539499998196886876 ) ) ;
#8599=CARTESIAN_POINT ( 'NONE',  ( 2.870125743571137811, 6.929096493489625530, -10.81838749981969094 ) ) ;
#8607=CARTESIAN_POINT ( 'NONE',  ( -2.163827323447878234E-09, -18.00000000000000000, -4.514799999819688381 ) ) ;
#8615=CIRCLE ( 'NONE', #5244, 2.649999999999999467 ) ;
#8616=CARTESIAN_POINT ( 'NONE',  ( -7.500000000000000888, 1.491842755816075172, -13.46916874991221391 ) ) ;
#8617=CARTESIAN_POINT ( 'NONE',  ( 15.25966317163202568, 10.19618095047498230, -7.754643749819691401 ) ) ;
#8618=CARTESIAN_POINT ( 'NONE',  ( 4.924999999999924327, -8.530350227276771946, -43.00000000000000000 ) ) ;
#8621=CARTESIAN_POINT ( 'NONE',  ( 10.32494394706616347, -4.276731815070950127, 7.656672250647431177 ) ) ;
#8625=DIRECTION ( 'NONE',  ( 1.000000000000000000, 0.000000000000000000, 0.000000000000000000 ) ) ;
#8630=CARTESIAN_POINT ( 'NONE',  ( 18.00000000000000000, -2.163824016901520184E-09, 4.458550000180312445 ) ) ;
#8632=DIRECTION ( 'NONE',  ( -0.000000000000000000, -0.000000000000000000, -1.000000000000000000 ) ) ;
#8639=EDGE_CURVE ( 'NONE', #2818, #19185, #11258, .T. ) ;
#8643=CARTESIAN_POINT ( 'NONE',  ( -14.79893867758297610, 1.779018419858781159E-09, 11.02779191884154564 ) ) ;
#8645=EDGE_CURVE ( 'NONE', #20518, #19935, #4538, .T. ) ;
#8648=CARTESIAN_POINT ( 'NONE',  ( -12.54593441562640166, 8.382925371439625906, -21.98169816848092850 ) ) ;
#8651=EDGE_CURVE ( 'NONE', #17634, #1625, #10923, .T. ) ;
#8655=DIRECTION ( 'NONE',  ( 1.000000000000000000, 0.000000000000000000, 0.000000000000000000 ) ) ;
#8656=CARTESIAN_POINT ( 'NONE',  ( -7.500000000000002665, 1.491842755816070509, 14.80583125008778822 ) ) ;
#8658=CARTESIAN_POINT ( 'NONE',  ( 6.358192987158596488, -4.248408730893249441, 7.522293750180316430 ) ) ;
#8661=CARTESIAN_POINT ( 'NONE',  ( -12.72792206288790950, -12.72792205982779556, 6.088325000180311086 ) ) ;
#8674=CARTESIAN_POINT ( 'NONE',  ( -5.303300859536636658, -5.303300858261589035, 0.7480750001803149196 ) ) ;
#8675=CARTESIAN_POINT ( 'NONE',  ( 11.17563879704981566, -2.222972771497744304, -9.185578500286805337 ) ) ;
#8685=CARTESIAN_POINT ( 'NONE',  ( 15.25966317163202746, 10.19618095047498407, 3.574956250180310935 ) ) ;
#8704=CARTESIAN_POINT ( 'NONE',  ( 4.248408730893245888, 6.358192987158590270, -10.52385624981969059 ) ) ;
#8712=CARTESIAN_POINT ( 'NONE',  ( 7.500000000000007994, 1.491842754878805577, 6.344168750087792574 ) ) ;
#8715=CARTESIAN_POINT ( 'NONE',  ( 12.72792205982779734, -12.72792206288791128, -5.692924999819687137 ) ) ;
#8724=AXIS2_PLACEMENT_3D ( 'NONE', #8749, #15215, #696 ) ;
#8725=( BOUNDED_CURVE ( )  B_SPLINE_CURVE ( 2, ( #19359, #4844, #9814, #11315, #3252, #1677, #14597, #72, #6528, #19464, #1008, #12349, #12669, #10855, #7777, #2596, #14252 ),
 .UNSPECIFIED., .F., .F. ) 
 B_SPLINE_CURVE_WITH_KNOTS ( ( 3, 2, 2, 2, 2, 2, 2, 2, 3 ),
 ( 0.6000000000038511194, 0.6125000000038511860, 0.6250000000038511416, 0.6375000000038510972, 0.6500000000038511638, 0.6625000000038511194, 0.6750000000038511860, 0.6875000000038511416, 0.7000000000038510972 ),
 .UNSPECIFIED. ) 
 CURVE ( )  GEOMETRIC_REPRESENTATION_ITEM ( )  RATIONAL_B_SPLINE_CURVE ( ( 0.9999999999940800688, 0.9807852804091503618, 1.000000000000000000, 0.9807852804032304306, 1.000000000000000000, 0.9807852804032304306, 1.000000000000000000, 0.9807852804032304306, 1.000000000000000000, 0.9807852804032304306, 1.000000000000000000, 0.9807852804032304306, 1.000000000000000000, 0.9807852804032304306, 1.000000000000000000, 0.9807852803973104994, 1.000000000005919931 ) ) 
 REPRESENTATION_ITEM ( '' )  );
#8727=CARTESIAN_POINT ( 'NONE',  ( -2.870125741905210415, 6.929096494179677990, -11.99651249981969414 ) ) ;
#8728=CARTESIAN_POINT ( 'NONE',  ( 12.72792205982779379, -12.72792206288790950, -15.11792499981969051 ) ) ;
#8731=CARTESIAN_POINT ( 'NONE',  ( -2.222972771497745192, -11.17563879704982632, 9.718391000647429223 ) ) ;
#8738=CARTESIAN_POINT ( 'NONE',  ( 17.99999999956958163, -3.580422614997676334, 14.17808125018031440 ) ) ;
#8739=CARTESIAN_POINT ( 'NONE',  ( 4.925000000000044231, 8.530350227276702668, -40.00000000000000000 ) ) ;
#8744=CARTESIAN_POINT ( 'NONE',  ( -6.358192987158597376, 4.248408730893249441, 12.23479375018031590 ) ) ;
#8749=CARTESIAN_POINT ( 'NONE',  ( 0.000000000000000000, 0.000000000000000000, 40.00000000000000000 ) ) ;
#8752=CARTESIAN_POINT ( 'NONE',  ( -13.67243654642775574, 5.663308650141533285, 21.04185441884154883 ) ) ;
#8755=CARTESIAN_POINT ( 'NONE',  ( 8.900000000000053646, 10.82531754730546147, 43.00000000000000000 ) ) ;
#8756=CARTESIAN_POINT ( 'NONE',  ( 12.54593441562639988, -8.382925371439625906, -26.69419816848093419 ) ) ;
#8761=ORIENTED_EDGE ( 'NONE', *, *, #8645, .T. ) ;
#8765=CARTESIAN_POINT ( 'NONE',  ( -16.62983158603121936, -6.888301780572499311, 6.677387500180310020 ) ) ;
#8772=CARTESIAN_POINT ( 'NONE',  ( 6.929096494179683319, 2.870125741905213079, -12.80036249981968766 ) ) ;
#8775=CARTESIAN_POINT ( 'NONE',  ( 1.491842754445843688, -7.500000000179346316, -0.7245812498196841922 ) ) ;
#8777=CARTESIAN_POINT ( 'NONE',  ( 10.32494394706615637, -4.276731815070946574, -8.891047250286803205 ) ) ;
#8781=CARTESIAN_POINT ( 'NONE',  ( 16.62983158603122291, 6.888301780572502864, -5.555512499819688088 ) ) ;
#8794=CYLINDRICAL_SURFACE ( 'NONE', #20087, 2.649999999999998579 ) ;
#8795=CARTESIAN_POINT ( 'NONE',  ( -4.248408730893245000, -6.358192987158590270, -15.23635624981969272 ) ) ;
#8797=CARTESIAN_POINT ( 'NONE',  ( 6.249999999999902300, -10.82531754730554496, 43.00000000000000000 ) ) ;
#8805=CARTESIAN_POINT ( 'NONE',  ( -17.99999999956958519, 3.580422614997674113, 7.560981250180312863 ) ) ;
#8818=CARTESIAN_POINT ( 'NONE',  ( -15.25966316918061416, 10.19618095414378445, -1.274956249819690024 ) ) ;
#8822=CARTESIAN_POINT ( 'NONE',  ( -6.358192988180015881, -4.248408729364577141, 13.62770625018031012 ) ) ;
#8824=CARTESIAN_POINT ( 'NONE',  ( 6.330490856366294494, -9.474249098604513364, -0.8847339993525716872 ) ) ;
#8828=FACE_OUTER_BOUND ( 'NONE', #10451, .T. ) ;
#8832=CARTESIAN_POINT ( 'NONE',  ( -2.163827323447878234E-09, -18.00000000000000000, 6.814800000180313511 ) ) ;
#8835=( BOUNDED_CURVE ( )  B_SPLINE_CURVE ( 2, ( #13221, #20853, #3360, #11213, #10040, #11429, #18097, #290, #17898, #9823, #19671, #3458, #14062, #16290, #17988, #9925, #14713 ),
 .UNSPECIFIED., .F., .F. ) 
 B_SPLINE_CURVE_WITH_KNOTS ( ( 3, 2, 2, 2, 2, 2, 2, 2, 3 ),
 ( 0.2000000000038511805, 0.2125000000038511638, 0.2250000000038511749, 0.2375000000038511860, 0.2500000000038511971, 0.2625000000038512082, 0.2750000000038512193, 0.2875000000038511749, 0.3000000000038511860 ),
 .UNSPECIFIED. ) 
 CURVE ( )  GEOMETRIC_REPRESENTATION_ITEM ( )  RATIONAL_B_SPLINE_CURVE ( ( 0.9999999999940800688, 0.9807852804091503618, 1.000000000000000000, 0.9807852804032304306, 1.000000000000000000, 0.9807852804032304306, 1.000000000000000000, 0.9807852804032304306, 1.000000000000000000, 0.9807852804032304306, 1.000000000000000000, 0.9807852804032304306, 1.000000000000000000, 0.9807852804032304306, 1.000000000000000000, 0.9807852803973104994, 1.000000000005919931 ) ) 
 REPRESENTATION_ITEM ( '' )  );
#8852=CARTESIAN_POINT ( 'NONE',  ( -14.79893867793684059, -2.943691925285399691, 10.73326066884154528 ) ) ;
#8860=CARTESIAN_POINT ( 'NONE',  ( 14.79893867722909917, -2.943691928843437111, -27.28326066848093490 ) ) ;
#8865=ORIENTED_EDGE ( 'NONE', *, *, #1832, .F. ) ;
#8870=CARTESIAN_POINT ( 'NONE',  ( -10.19618095047497874, 15.25966317163202746, 8.739106250180309843 ) ) ;
#8880=CARTESIAN_POINT ( 'NONE',  ( -17.99999999956958874, 3.580422614997675002, 18.89058125018030765 ) ) ;
#8882=CARTESIAN_POINT ( 'NONE',  ( -2.870125741905213079, 6.929096494179683319, -5.731612499819686235 ) ) ;
#8883=VECTOR ( 'NONE', #2954, 1000.000000000000000 ) ;
#8884=CARTESIAN_POINT ( 'NONE',  ( 5.303300858261588147, -5.303300859536636658, 17.24182500018031661 ) ) ;
#8887=CARTESIAN_POINT ( 'NONE',  ( 7.902369976724389566, -7.902369978624323110, -8.301984750286806047 ) ) ;
#8894=DIRECTION ( 'NONE',  ( 0.000000000000000000, 0.000000000000000000, 1.000000000000000000 ) ) ;
#8895=CARTESIAN_POINT ( 'NONE',  ( -17.99999999956958519, 3.580422614997674113, -9.384418749819685601 ) ) ;
#8910=AXIS2_PLACEMENT_3D ( 'NONE', #1770, #19259, #8124 ) ;
#8912=CARTESIAN_POINT ( 'NONE',  ( -2.870125743571140919, -6.929096493489624642, -6.105887499819689701 ) ) ;
#8919=ORIENTED_EDGE ( 'NONE', *, *, #10693, .F. ) ;
#8922=CARTESIAN_POINT ( 'NONE',  ( -15.25966317163203279, -10.19618095047498052, -3.042143749819686160 ) ) ;
#8936=CARTESIAN_POINT ( 'NONE',  ( -16.62983158603121936, -6.888301780572499311, -12.17261249981969229 ) ) ;
#8942=CARTESIAN_POINT ( 'NONE',  ( 2.222972768810839383, -11.17563879758428769, -19.14567149935257007 ) ) ;
#8943=EDGE_LOOP ( 'NONE', ( #4716, #14205, #7759, #18297, #11121, #11388 ) ) ;
#8946=EDGE_LOOP ( 'NONE', ( #8056, #12185 ) ) ;
#8950=CARTESIAN_POINT ( 'NONE',  ( 10.19618095414378800, 15.25966316918061416, -15.86410624981969164 ) ) ;
#8952=DIRECTION ( 'NONE',  ( 0.000000000000000000, 0.000000000000000000, -1.000000000000000000 ) ) ;
#8966=CARTESIAN_POINT ( 'NONE',  ( 8.382925371439633011, 12.54593441562640876, 4.842635668841546170 ) ) ;
#8973=EDGE_CURVE ( 'NONE', #14958, #14416, #4149, .T. ) ;
#8974=CARTESIAN_POINT ( 'NONE',  ( -2.163827323447877821E-09, -17.99999999999999645, 4.910200000180310553 ) ) ;
#8975=CARTESIAN_POINT ( 'NONE',  ( 18.00000000000000000, -2.163824016901520184E-09, 23.30855000018031475 ) ) ;
#8977=ORIENTED_EDGE ( 'NONE', *, *, #9161, .T. ) ;
#8981=VERTEX_POINT ( 'NONE', #7899 ) ;
#8985=CARTESIAN_POINT ( 'NONE',  ( 6.929096493489625530, -2.870125743571142252, 0.9628625001803087224 ) ) ;
#8986=CARTESIAN_POINT ( 'NONE',  ( 17.99999999999999645, -2.163824016901520184E-09, -16.29604999981969371 ) ) ;
#8994=CARTESIAN_POINT ( 'NONE',  ( 3.580422610670021211, -18.00000000043041481, -2.904731249819689776 ) ) ;
#8995=PRODUCT_DEFINITION_CONTEXT ( 'detailed design', #17546, 'design' ) ;
#8999=CARTESIAN_POINT ( 'NONE',  ( -6.358192988180021210, -4.248408729364580694, -8.382393749819687656 ) ) ;
#9004=CARTESIAN_POINT ( 'NONE',  ( -6.330490858644137298, -9.474249097082495297, -15.66526600028680782 ) ) ;
#9009=CARTESIAN_POINT ( 'NONE',  ( -16.62983158603122291, -6.888301780572501087, -0.8430124998196862895 ) ) ;
#9013=ORIENTED_EDGE ( 'NONE', *, *, #17358, .F. ) ;
#9027=CIRCLE ( 'NONE', #2607, 2.649999999999999467 ) ;
#9028=CARTESIAN_POINT ( 'NONE',  ( -7.500000000000000888, 9.015942588607330751E-10, -4.338699999819690234 ) ) ;
#9038=CARTESIAN_POINT ( 'NONE',  ( -18.00000000000000000, 2.163826221265758884E-09, 7.266450000180315172 ) ) ;
#9047=ORIENTED_EDGE ( 'NONE', *, *, #10403, .T. ) ;
#9064=DIRECTION ( 'NONE',  ( -0.000000000000000000, -0.000000000000000000, 1.000000000000000000 ) ) ;
#9067=CARTESIAN_POINT ( 'NONE',  ( -3.580422610670018546, 18.00000000043041126, -17.04223124981968596 ) ) ;
#9074=CARTESIAN_POINT ( 'NONE',  ( 7.500000000000008882, 1.491842754878802690, 15.76916875008778973 ) ) ;
#9079=CARTESIAN_POINT ( 'NONE',  ( 8.382925368423272516, -12.54593441764187745, 7.787948168841544394 ) ) ;
#9086=CARTESIAN_POINT ( 'NONE',  ( -3.580422610670017658, 18.00000000043040771, 9.328168750180312330 ) ) ;
#9092=LINE ( 'NONE', #17036, #7018 ) ;
#9096=CARTESIAN_POINT ( 'NONE',  ( 3.580422610670019878, -18.00000000043040771, -14.23433124981968945 ) ) ;
#9102=CARTESIAN_POINT ( 'NONE',  ( 0.000000000000000000, 0.000000000000000000, 40.00000000000000000 ) ) ;
#9104=CARTESIAN_POINT ( 'NONE',  ( -16.62983158603122646, -6.888301780572501976, -0.8430124998196897312 ) ) ;
#9105=ADVANCED_FACE ( 'NONE', ( #9176 ), #15634, .T. ) ;
#9110=CARTESIAN_POINT ( 'NONE',  ( 5.663308646854338768, -13.67243654778934747, 11.88939558151907683 ) ) ;
#9114=CARTESIAN_POINT ( 'NONE',  ( -9.850000000000006750, 0.000000000000000000, 43.00000000000000000 ) ) ;
#9130=CARTESIAN_POINT ( 'NONE',  ( -7.499999999820661678, 1.491842756249031288, -22.89416874981969130 ) ) ;
#9138=CARTESIAN_POINT ( 'NONE',  ( 10.19618095414378800, 15.25966316918061416, -8.343706249819687670 ) ) ;
#9143=ORIENTED_EDGE ( 'NONE', *, *, #2506, .T. ) ;
#9148=CARTESIAN_POINT ( 'NONE',  ( 6.929096493489630859, -2.870125743571144472, -21.04723749981969050 ) ) ;
#9150=CARTESIAN_POINT ( 'NONE',  ( -3.580422610670017658, 18.00000000043040771, -18.94683124981969158 ) ) ;
#9156=CARTESIAN_POINT ( 'NONE',  ( -12.50000000000000533, 0.000000000000000000, 43.00000000000000000 ) ) ;
#9161=EDGE_CURVE ( 'NONE', #10032, #14416, #16567, .T. ) ;
#9164=CARTESIAN_POINT ( 'NONE',  ( 15.25966316918061416, -10.19618095414378622, -13.50785624981968702 ) ) ;
#9168=DIRECTION ( 'NONE',  ( -0.1159034202170323435, 1.393303357259113989E-11, -0.9932604880805406822 ) ) ;
#9174=CIRCLE ( 'NONE', #11871, 17.50000000000000355 ) ;
#9176=FACE_OUTER_BOUND ( 'NONE', #16019, .T. ) ;
#9177=CARTESIAN_POINT ( 'NONE',  ( -13.67243654642775574, 5.663308650141533285, -7.233145581158455961 ) ) ;
#9183=CARTESIAN_POINT ( 'NONE',  ( 10.19618095414378622, 15.25966316918061239, 1.081293750180310820 ) ) ;
#9195=CARTESIAN_POINT ( 'NONE',  ( -17.99999999956958163, 3.580422614997673669, -11.28901874981968945 ) ) ;
#9205=CARTESIAN_POINT ( 'NONE',  ( 12.72792206288791128, 12.72792205982780267, 3.280425000180310580 ) ) ;
#9210=CARTESIAN_POINT ( 'NONE',  ( -7.500000000000007994, -1.491842754878805355, 20.48166875008779542 ) ) ;
#9211=CARTESIAN_POINT ( 'NONE',  ( -13.67243654778935102, -5.663308646854334327, 4.820645581519075407 ) ) ;
#9215=CARTESIAN_POINT ( 'NONE',  ( -2.163827323447878234E-09, -18.00000000000000000, -21.46019999981968951 ) ) ;
#9230=CARTESIAN_POINT ( 'NONE',  ( 9.470358143689582064, -1.138454911109690799E-09, 8.603271702811174038 ) ) ;
#9234=CARTESIAN_POINT ( 'NONE',  ( 7.500000000179339210, 1.491842754445841690, -18.77073124981968988 ) ) ;
#9244=CARTESIAN_POINT ( 'NONE',  ( -16.62983158437510056, 6.888301784570729502, -10.99448749981968554 ) ) ;
#9255=VERTEX_POINT ( 'NONE', #8109 ) ;
#9261=AXIS2_PLACEMENT_3D ( 'NONE', #9230, #16007, #12415 ) ;
#9271=VERTEX_POINT ( 'NONE', #14580 ) ;
#9272=CARTESIAN_POINT ( 'NONE',  ( 18.00000000043041126, 3.580422610670019434, -5.260981249819686845 ) ) ;
#9287=CARTESIAN_POINT ( 'NONE',  ( 5.663308650141532397, 13.67243654642775574, -4.876895581158458448 ) ) ;
#9292=CARTESIAN_POINT ( 'NONE',  ( -7.500000000000004441, -1.491842754878798916, -23.48323124991221178 ) ) ;
#9293=CARTESIAN_POINT ( 'NONE',  ( -12.72792206288790950, -12.72792205982779556, 6.088325000180311086 ) ) ;
#9295=CARTESIAN_POINT ( 'NONE',  ( 5.303300859536631329, 5.303300858261585482, -19.65432499981969627 ) ) ;
#9303=CARTESIAN_POINT ( 'NONE',  ( 17.99999999956957808, -3.580422614997675446, -16.00151874981969158 ) ) ;
#9308=PLANE ( 'NONE',  #17683 ) ;
#9309=CARTESIAN_POINT ( 'NONE',  ( -12.50000000000000533, 0.000000000000000000, -43.00000000000000000 ) ) ;
#9311=CARTESIAN_POINT ( 'NONE',  ( -18.00000000043041481, -3.580422610670022987, -0.5484812498196925956 ) ) ;
#9312=CARTESIAN_POINT ( 'NONE',  ( -5.303300859536636658, -5.303300858261589035, -18.10192499981969050 ) ) ;
#9317=CARTESIAN_POINT ( 'NONE',  ( -10.46442989454075168, -10.46442989202483709, 13.65658308151907541 ) ) ;
#9322=CARTESIAN_POINT ( 'NONE',  ( -16.62983158603122291, -6.888301780572501087, -19.69301249981969093 ) ) ;
#9337=CARTESIAN_POINT ( 'NONE',  ( 9.474249097082498849, -6.330490858644140850, -1.473796499352572953 ) ) ;
#9339=CARTESIAN_POINT ( 'NONE',  ( -6.358192987158591158, 4.248408730893245000, -22.30510624981969059 ) ) ;
#9348=CARTESIAN_POINT ( 'NONE',  ( -6.888301784570738384, -16.62983158437509346, -13.35073749981969016 ) ) ;
#9351=VERTEX_POINT ( 'NONE', #7347 ) ;
#9363=CARTESIAN_POINT ( 'NONE',  ( -15.25966316918061416, 10.19618095414378445, -20.12495624981969300 ) ) ;
#9368=CARTESIAN_POINT ( 'NONE',  ( -5.303300859536632217, -5.303300858261584594, 13.33317500018030977 ) ) ;
#9370=EDGE_CURVE ( 'NONE', #16482, #13364, #8566, .T. ) ;
#9381=CARTESIAN_POINT ( 'NONE',  ( 18.00000000043041126, 3.580422610670019434, -14.68598124981969022 ) ) ;
#9397=CARTESIAN_POINT ( 'NONE',  ( 5.663308646854342321, -13.67243654778935635, -1.342520581158454851 ) ) ;
#9398=VERTEX_POINT ( 'NONE', #12224 ) ;
#9409=DIRECTION ( 'NONE',  ( -0.000000000000000000, -0.000000000000000000, 1.000000000000000000 ) ) ;
#9415=CARTESIAN_POINT ( 'NONE',  ( 17.99999999999999645, -2.163824016901520184E-09, -6.871049999819689447 ) ) ;
#9416=SHAPE_REPRESENTATION ( 'worm', ( #12461 ), #7026 ) ;
#9421=CARTESIAN_POINT ( 'NONE',  ( 6.250000000000054179, 10.82531754730546147, 43.00000000000000000 ) ) ;
#9423=CARTESIAN_POINT ( 'NONE',  ( -12.72792205982780089, 12.72792206288791128, 0.9241750001803099579 ) ) ;
#9424=CARTESIAN_POINT ( 'NONE',  ( 6.358192987158595599, -4.248408730893249441, -20.75270624981969192 ) ) ;
#9427=CARTESIAN_POINT ( 'NONE',  ( 11.17563879704981566, -2.222972771497744304, -28.03557850028681031 ) ) ;
#9433=CARTESIAN_POINT ( 'NONE',  ( 8.899999999999900879, -10.82531754730554496, 40.00000000000000000 ) ) ;
#9436=VERTEX_POINT ( 'NONE', #2271 ) ;
#9440=ORIENTED_EDGE ( 'NONE', *, *, #3165, .T. ) ;
#9444=CARTESIAN_POINT ( 'NONE',  ( 11.17563879731705789, -1.343450868547281933E-09, -11.78239024935257540 ) ) ;
#9445=CARTESIAN_POINT ( 'NONE',  ( 2.870125743571137811, 6.929096493489625530, -20.24338749981969343 ) ) ;
#9452=CARTESIAN_POINT ( 'NONE',  ( -15.25966317163203279, -10.19618095047498052, -21.89214374981969158 ) ) ;
#9457=CARTESIAN_POINT ( 'NONE',  ( -4.248408730893246776, -6.358192987158592047, -5.811356249819692898 ) ) ;
#9464=CARTESIAN_POINT ( 'NONE',  ( -16.62983158437509701, 6.888301784570728614, -20.41948749981969158 ) ) ;
#9475=ORIENTED_EDGE ( 'NONE', *, *, #11818, .F. ) ;
#9485=EDGE_CURVE ( 'NONE', #13866, #20036, #1563, .T. ) ;
#9491=CARTESIAN_POINT ( 'NONE',  ( -4.276731815070949239, -10.32494394706616347, 19.43792225064743562 ) ) ;
#9500=EDGE_CURVE ( 'NONE', #1825, #100, #4875, .T. ) ;
#9512=LINE ( 'NONE', #1477, #10056 ) ;
#9516=CARTESIAN_POINT ( 'NONE',  ( -15.25966317163203456, -10.19618095047498230, -10.56254374981969413 ) ) ;
#9520=CARTESIAN_POINT ( 'NONE',  ( -4.276731815070945686, -10.32494394706615637, -25.38479725028680889 ) ) ;
#9541=CARTESIAN_POINT ( 'NONE',  ( 9.474249098604511587, 6.330490856366296271, -12.66598399935257468 ) ) ;
#9544=CARTESIAN_POINT ( 'NONE',  ( 7.499999999820660790, -1.491842756249031954, -18.18166874981969272 ) ) ;
#9549=ORIENTED_EDGE ( 'NONE', *, *, #11938, .T. ) ;
#9552=CARTESIAN_POINT ( 'NONE',  ( 15.25966317163202746, 10.19618095047498407, -17.17964374981969300 ) ) ;
#9559=CARTESIAN_POINT ( 'NONE',  ( -4.248408729364577141, 6.358192988180014993, -2.866043749819691122 ) ) ;
#9568=CARTESIAN_POINT ( 'NONE',  ( 5.303300858261583706, -5.303300859536632217, 10.97692500018030870 ) ) ;
#9570=ORIENTED_EDGE ( 'NONE', *, *, #4167, .T. ) ;
#9572=CARTESIAN_POINT ( 'NONE',  ( 7.500000000000005329, -1.491842755816077393, -2.491768749912207870 ) ) ;
#9596=CARTESIAN_POINT ( 'NONE',  ( 8.382925371439633011, 12.54593441562640876, -14.00736433115846324 ) ) ;
#9611=CIRCLE ( 'NONE', #11961, 2.649999999999999467 ) ;
#9629=CARTESIAN_POINT ( 'NONE',  ( -12.72792206288791483, -12.72792205982780089, -20.28207499981969519 ) ) ;
#9636=CARTESIAN_POINT ( 'NONE',  ( 12.54593441562639988, -8.382925371439625906, -7.844198168480929212 ) ) ;
#9643=DIRECTION ( 'NONE',  ( 0.000000000000000000, 0.000000000000000000, -1.000000000000000000 ) ) ;
#9644=DIRECTION ( 'NONE',  ( -0.000000000000000000, -0.000000000000000000, 1.000000000000000000 ) ) ;
#9651=ORIENTED_EDGE ( 'NONE', *, *, #12128, .F. ) ;
#9657=CARTESIAN_POINT ( 'NONE',  ( -4.248408729364580694, 6.358192988180020322, 12.82385625018031483 ) ) ;
#9659=CARTESIAN_POINT ( 'NONE',  ( 9.474249097082495297, -6.330490858644137298, 0.8284839997131990819 ) ) ;
#9661=( BOUNDED_CURVE ( )  B_SPLINE_CURVE ( 2, ( #12394, #9210, #2542, #5595, #7402, #10807, #18436, #20445, #10593, #15564, #13879, #2423, #8884, #3899, #7185, #12077, #13778 ),
 .UNSPECIFIED., .F., .F. ) 
 B_SPLINE_CURVE_WITH_KNOTS ( ( 3, 2, 2, 2, 2, 2, 2, 2, 3 ),
 ( 0.1000000000038511888, 0.1125000000038511860, 0.1250000000038511694, 0.1375000000038511805, 0.1500000000038511638, 0.1625000000038511749, 0.1750000000038511583, 0.1875000000038511694, 0.2000000000038511805 ),
 .UNSPECIFIED. ) 
 CURVE ( )  GEOMETRIC_REPRESENTATION_ITEM ( )  RATIONAL_B_SPLINE_CURVE ( ( 0.9999999999940800688, 0.9807852804091503618, 1.000000000000000000, 0.9807852804032304306, 1.000000000000000000, 0.9807852804032304306, 1.000000000000000000, 0.9807852804032304306, 1.000000000000000000, 0.9807852804032304306, 1.000000000000000000, 0.9807852804032304306, 1.000000000000000000, 0.9807852804032304306, 1.000000000000000000, 0.9807852803973104994, 1.000000000005919931 ) ) 
 REPRESENTATION_ITEM ( '' )  );
#9664=EDGE_LOOP ( 'NONE', ( #18747, #6141, #7215, #8919 ) ) ;
#9666=ORIENTED_EDGE ( 'NONE', *, *, #11190, .T. ) ;
#9667=CARTESIAN_POINT ( 'NONE',  ( -12.72792206288791128, -12.72792205982779912, 7.992925000180314044 ) ) ;
#9669=VERTEX_POINT ( 'NONE', #8182 ) ;
#9678=DIRECTION ( 'NONE',  ( 0.000000000000000000, 0.000000000000000000, -1.000000000000000000 ) ) ;
#9684=CARTESIAN_POINT ( 'NONE',  ( 6.929096493489630859, -2.870125743571144472, -2.197237499819686857 ) ) ;
#9703=CARTESIAN_POINT ( 'NONE',  ( -11.17563879731705789, 1.343452237168309506E-09, 21.20510975064742709 ) ) ;
#9713=DIRECTION ( 'NONE',  ( 1.202124453834178339E-10, 1.000000000000000000, 8.650973189387494397E-26 ) ) ;
#9720=CARTESIAN_POINT ( 'NONE',  ( -2.163827323447877821E-09, -17.99999999999999645, -23.36479999981969158 ) ) ;
#9724=EDGE_CURVE ( 'NONE', #13652, #9255, #17849, .T. ) ;
#9728=CARTESIAN_POINT ( 'NONE',  ( 15.25966316918061771, -10.19618095414378800, -13.50785624981969235 ) ) ;
#9729=AXIS2_PLACEMENT_3D ( 'NONE', #6164, #18907, #1527 ) ;
#9735=CARTESIAN_POINT ( 'NONE',  ( -5.663308646854335215, 13.67243654778934925, -2.248104418480928235 ) ) ;
#9749=CARTESIAN_POINT ( 'NONE',  ( -15.25966317163202923, -10.19618095047497874, 15.80785625018031304 ) ) ;
#9758=CARTESIAN_POINT ( 'NONE',  ( 4.248408730893249441, 6.358192987158595599, 14.59104375018031519 ) ) ;
#9759=CARTESIAN_POINT ( 'NONE',  ( 4.276731815070940357, 10.32494394706615815, -1.822297250286802450 ) ) ;
#9765=CARTESIAN_POINT ( 'NONE',  ( -12.72792205982779912, 12.72792206288790950, 10.34917500018031333 ) ) ;
#9775=ORIENTED_EDGE ( 'NONE', *, *, #18575, .T. ) ;
#9781=CARTESIAN_POINT ( 'NONE',  ( 1.491842754445842134, -7.500000000179339210, 11.86051875018031332 ) ) ;
#9791=FACE_OUTER_BOUND ( 'NONE', #9664, .T. ) ;
#9797=CARTESIAN_POINT ( 'NONE',  ( 9.474249098604511587, 6.330490856366296271, 25.03401600064742993 ) ) ;
#9801=ADVANCED_FACE ( 'NONE', ( #13578 ), #8794, .F. ) ;
#9804=CARTESIAN_POINT ( 'NONE',  ( 7.500000000000002665, -9.015933403756338579E-10, -27.90119999981969556 ) ) ;
#9806=CARTESIAN_POINT ( 'NONE',  ( -12.50000000000000533, 0.000000000000000000, -43.00000000000000000 ) ) ;
#9807=CYLINDRICAL_SURFACE ( 'NONE', #17504, 2.649999999999999467 ) ;
#9811=VERTEX_POINT ( 'NONE', #11989 ) ;
#9814=CARTESIAN_POINT ( 'NONE',  ( 6.929096494179683319, 2.870125741905213079, -3.375362499819685613 ) ) ;
#9820=CARTESIAN_POINT ( 'NONE',  ( 18.00000000000000355, -2.163824016901520597E-09, -4.966449999819690042 ) ) ;
#9823=CARTESIAN_POINT ( 'NONE',  ( -1.491842754445841690, 7.500000000179340987, 7.148018750180309411 ) ) ;
#9825=CARTESIAN_POINT ( 'NONE',  ( 14.79893867758296544, -1.779016607511491977E-09, 0.6972080815190739855 ) ) ;
#9831=CARTESIAN_POINT ( 'NONE',  ( 5.303300859536635770, 5.303300858261589923, 24.31057500018031803 ) ) ;
#9849=CARTESIAN_POINT ( 'NONE',  ( -2.870125743571144028, -6.929096493489630859, 19.00901250018031519 ) ) ;
#9850=CARTESIAN_POINT ( 'NONE',  ( -11.17563879704981922, 2.222972771497742972, -4.473078500286804093 ) ) ;
#9854=CIRCLE ( 'NONE', #10188, 17.50000000000000355 ) ;
#9857=ADVANCED_FACE ( 'NONE', ( #10299 ), #17079, .F. ) ;
#9858=CARTESIAN_POINT ( 'NONE',  ( -10.19618095047498052, 15.25966317163203101, 10.64370625018031191 ) ) ;
#9878=CARTESIAN_POINT ( 'NONE',  ( -4.248408729364575365, 6.358192988180014105, 6.558956250180312253 ) ) ;
#9887=CARTESIAN_POINT ( 'NONE',  ( -3.580422614997675002, -17.99999999956958163, 14.62973125018031517 ) ) ;
#9892=CARTESIAN_POINT ( 'NONE',  ( 7.500000000000000000, 9.184850993605147944E-16, 40.00000000000000000 ) ) ;
#9900=CARTESIAN_POINT ( 'NONE',  ( 11.17563879758428769, 2.222972768810838939, 25.62307850064743420 ) ) ;
#9902=EDGE_LOOP ( 'NONE', ( #664, #12951, #15968, #6449 ) ) ;
#9903=DIRECTION ( 'NONE',  ( 1.000000000000000000, 0.000000000000000000, 0.000000000000000000 ) ) ;
#9909=CARTESIAN_POINT ( 'NONE',  ( 3.580422610670020322, -18.00000000043041126, 15.94526875018031298 ) ) ;
#9920=DIRECTION ( 'NONE',  ( 0.5017436386064959564, -6.031582975246068435E-11, 0.8650163704334813408 ) ) ;
#9923=CARTESIAN_POINT ( 'NONE',  ( -3.580422614997675890, -17.99999999956958519, -11.74066874981969555 ) ) ;
#9925=CARTESIAN_POINT ( 'NONE',  ( -7.500000000000002665, 1.491842755816068955, 5.380831250087785733 ) ) ;
#9929=CARTESIAN_POINT ( 'NONE',  ( 12.54593441562639988, -8.382925371439625906, 1.580801831519075495 ) ) ;
#9930=ORIENTED_EDGE ( 'NONE', *, *, #6690, .F. ) ;
#9949=CIRCLE ( 'NONE', #19768, 17.50000000000000355 ) ;
#9954=CARTESIAN_POINT ( 'NONE',  ( -5.303300858261589035, 5.303300859536635770, 21.95432500018031874 ) ) ;
#9956=CARTESIAN_POINT ( 'NONE',  ( 7.902369976724389566, -7.902369978624323110, 10.54801524971320070 ) ) ;
#9962=CARTESIAN_POINT ( 'NONE',  ( 10.19618095047497874, -15.25966317163203279, 15.35620625018031404 ) ) ;
#9982=CARTESIAN_POINT ( 'NONE',  ( 6.929096494179676213, 2.870125741905210415, 18.63473750018031083 ) ) ;
#9994=CYLINDRICAL_SURFACE ( 'NONE', #15670, 2.649999999999999467 ) ;
#10000=VERTEX_POINT ( 'NONE', #20775 ) ;
#10004=ADVANCED_FACE ( 'NONE', ( #20665 ), #7422, .T. ) ;
#10008=CARTESIAN_POINT ( 'NONE',  ( 7.902369976724399336, -7.902369978624331104, 17.67073475064742993 ) ) ;
#10031=CARTESIAN_POINT ( 'NONE',  ( -4.248408730893249441, -6.358192987158596488, -18.39645624981969263 ) ) ;
#10032=VERTEX_POINT ( 'NONE', #17292 ) ;
#10033=CARTESIAN_POINT ( 'NONE',  ( 0.000000000000000000, 0.000000000000000000, -43.00000000000000000 ) ) ;
#10037=CARTESIAN_POINT ( 'NONE',  ( -1.779019326032424922E-09, -14.79893867758297610, 8.671541918841546348 ) ) ;
#10040=CARTESIAN_POINT ( 'NONE',  ( 5.303300859536631329, 5.303300858261585482, 8.620675000180307634 ) ) ;
#10044=CARTESIAN_POINT ( 'NONE',  ( 5.663308646854338768, -13.67243654778934747, -6.960604418480926370 ) ) ;
#10046=( GEOMETRIC_REPRESENTATION_CONTEXT ( 3 ) GLOBAL_UNCERTAINTY_ASSIGNED_CONTEXT ( ( #12171 ) ) GLOBAL_UNIT_ASSIGNED_CONTEXT ( ( #234, #19927, #19618 ) ) REPRESENTATION_CONTEXT ( 'NONE', 'WORKASPACE' ) );
#10052=CARTESIAN_POINT ( 'NONE',  ( -2.870125743571144028, -6.929096493489630859, 9.584012500180316252 ) ) ;
#10055=CARTESIAN_POINT ( 'NONE',  ( 2.163825119083639120E-09, 17.99999999999999645, 9.622700000180310909 ) ) ;
#10056=VECTOR ( 'NONE', #7491, 1000.000000000000000 ) ;
#10066=CARTESIAN_POINT ( 'NONE',  ( -6.358192987158596488, 4.248408730893249441, 21.65979375018031661 ) ) ;
#10069=CARTESIAN_POINT ( 'NONE',  ( 6.330490858644138186, 9.474249097082495297, 7.897233999713197505 ) ) ;
#10072=CARTESIAN_POINT ( 'NONE',  ( 7.500000000000009770, -8.788009009181406898E-15, -12.21129999999768501 ) ) ;
#10077=CARTESIAN_POINT ( 'NONE',  ( -18.00000000000000000, 2.163826221265758884E-09, 18.59605000018031262 ) ) ;
#10091=CARTESIAN_POINT ( 'NONE',  ( 7.499999999820660790, -1.491842756249031954, 10.09333125018031119 ) ) ;
#10096=MANIFOLD_SOLID_BREP ( 'Mirror1', #5562 ) ;
#10101=DIRECTION ( 'NONE',  ( -0.000000000000000000, -0.000000000000000000, 1.000000000000000000 ) ) ;
#10116=CARTESIAN_POINT ( 'NONE',  ( 11.17563879704982632, -2.222972771497745637, 7.362141000647429934 ) ) ;
#10124=CARTESIAN_POINT ( 'NONE',  ( -15.25966316918061771, 10.19618095414378622, 0.6296437501803129333 ) ) ;
#10138=CARTESIAN_POINT ( 'NONE',  ( -14.79893867758297610, 1.779018419858781159E-09, 20.45279191884155168 ) ) ;
#10145=CARTESIAN_POINT ( 'NONE',  ( 6.888301784570727726, 16.62983158437509701, 19.63676250018031411 ) ) ;
#10150=CARTESIAN_POINT ( 'NONE',  ( -2.870125741905210415, 6.929096494179677990, 16.27848750018030799 ) ) ;
#10155=CARTESIAN_POINT ( 'NONE',  ( -12.72792205982779556, 12.72792206288790773, 8.444575000180309488 ) ) ;
#10163=CARTESIAN_POINT ( 'NONE',  ( 10.19618095414378978, 15.25966316918061771, 21.83589375018031475 ) ) ;
#10164=CARTESIAN_POINT ( 'NONE',  ( 7.499999999820668783, -1.491842756249033508, -2.491768749819687656 ) ) ;
#10165=CARTESIAN_POINT ( 'NONE',  ( 10.32494394809438987, 4.276731812588564274, -19.49417225028681244 ) ) ;
#10170=FACE_OUTER_BOUND ( 'NONE', #11872, .T. ) ;
#10172=CARTESIAN_POINT ( 'NONE',  ( 17.99999999956958163, -3.580422614997676334, 4.753081250180312800 ) ) ;
#10188=AXIS2_PLACEMENT_3D ( 'NONE', #18731, #10878, #18943 ) ;
#10189=CARTESIAN_POINT ( 'NONE',  ( -6.358192987158591158, 4.248408730893245000, -12.88010624981968810 ) ) ;
#10198=CARTESIAN_POINT ( 'NONE',  ( 3.580422614997668340, 17.99999999956958519, 9.917231250180313040 ) ) ;
#10207=COLOUR_RGB ( '', 0.31764706, 0.68627451, 0.89019608) ;
#10210=CARTESIAN_POINT ( 'NONE',  ( 6.929096494179677990, 2.870125741905210859, -9.640262499819693076 ) ) ;
#10211=CARTESIAN_POINT ( 'NONE',  ( -17.99999999999999645, 2.163826221265758470E-09, -11.58354999981969158 ) ) ;
#10215=CARTESIAN_POINT ( 'NONE',  ( 10.32494394809439875, 4.276731812588567827, 15.90354725064743135 ) ) ;
#10219=CARTESIAN_POINT ( 'NONE',  ( 0.000000000000000000, 0.000000000000000000, -40.00000000000000000 ) ) ;
#10225=CARTESIAN_POINT ( 'NONE',  ( -10.19618095414378622, -15.25966316918061416, -1.726606249819687910 ) ) ;
#10239=CARTESIAN_POINT ( 'NONE',  ( 8.382925368423272516, -12.54593441764187745, 17.21294816884154955 ) ) ;
#10247=CARTESIAN_POINT ( 'NONE',  ( 14.79893867758296544, -1.779016607511491977E-09, -18.15279191848092921 ) ) ;
#10250=ADVANCED_FACE ( 'NONE', ( #2215 ), #12172, .T. ) ;
#10257=CARTESIAN_POINT ( 'NONE',  ( -4.248408730893249441, -6.358192987158596488, 9.878543750180313054 ) ) ;
#10260=CARTESIAN_POINT ( 'NONE',  ( -17.99999999956958163, 3.580422614997673669, 7.560981250180310198 ) ) ;
#10268=CARTESIAN_POINT ( 'NONE',  ( 6.250000000000054179, 10.82531754730546147, -43.00000000000000000 ) ) ;
#10269=CARTESIAN_POINT ( 'NONE',  ( 16.62983158603122646, 6.888301780572504640, 22.71948750018031049 ) ) ;
#10273=CARTESIAN_POINT ( 'NONE',  ( -6.929096494179684207, -2.870125741905212635, -8.087862499819687301 ) ) ;
#10274=CARTESIAN_POINT ( 'NONE',  ( 2.222972771497739419, 11.17563879704981922, -20.96682850028681244 ) ) ;
#10283=CARTESIAN_POINT ( 'NONE',  ( -6.888301784570738384, -16.62983158437509346, -11.44613749981969164 ) ) ;
#10299=FACE_OUTER_BOUND ( 'NONE', #19689, .T. ) ;
#10302=CARTESIAN_POINT ( 'NONE',  ( 7.500000000000000888, -9.015933403756337545E-10, 0.3738000001803111205 ) ) ;
#10311=CARTESIAN_POINT ( 'NONE',  ( -16.62983158603122291, -6.888301780572501087, 6.677387500180313573 ) ) ;
#10315=VERTEX_POINT ( 'NONE', #12893 ) ;
#10321=CARTESIAN_POINT ( 'NONE',  ( 6.888301780572505528, -16.62983158603121581, -14.52886249981968980 ) ) ;
#10324=CARTESIAN_POINT ( 'NONE',  ( 6.330490856366294494, -9.474249098604513364, 8.540266000647427802 ) ) ;
#10330=EDGE_LOOP ( 'NONE', ( #16862, #5636 ) ) ;
#10332=CARTESIAN_POINT ( 'NONE',  ( 12.72792205982779734, -12.72792206288791128, -3.788324999819688177 ) ) ;
#10345=AXIS2_PLACEMENT_3D ( 'NONE', #17926, #4888, #4682 ) ;
#10348=CARTESIAN_POINT ( 'NONE',  ( 8.382925371439633011, 12.54593441562640876, 23.69263566884154670 ) ) ;
#10351=ORIENTED_EDGE ( 'NONE', *, *, #2089, .T. ) ;
#10353=CARTESIAN_POINT ( 'NONE',  ( -5.663308650141535949, -13.67243654642774686, -15.20747941848092921 ) ) ;
#10357=AXIS2_PLACEMENT_3D ( 'NONE', #1866, #9713, #8320 ) ;
#10361=VERTEX_POINT ( 'NONE', #11293 ) ;
#10366=CARTESIAN_POINT ( 'NONE',  ( -10.19618095414378445, -15.25966316918061239, 15.21879375018031233 ) ) ;
#10379=CARTESIAN_POINT ( 'NONE',  ( -5.303300858261589035, 5.303300859536635770, 3.104325000180315541 ) ) ;
#10381=CARTESIAN_POINT ( 'NONE',  ( 11.17563879758427525, 2.222972768810836719, -9.774641000286804271 ) ) ;
#10389=CARTESIAN_POINT ( 'NONE',  ( -10.19618095414378622, -15.25966316918061416, -1.726606249819687688 ) ) ;
#10395=VERTEX_POINT ( 'NONE', #20618 ) ;
#10403=EDGE_CURVE ( 'NONE', #16910, #1886, #4517, .T. ) ;
#10408=CARTESIAN_POINT ( 'NONE',  ( 6.929096494179676213, 2.870125741905210415, -0.2152624998196898953 ) ) ;
#10417=CARTESIAN_POINT ( 'NONE',  ( 6.358192988180019434, 4.248408729364581582, 5.755106250180313410 ) ) ;
#10419=CARTESIAN_POINT ( 'NONE',  ( -3.580422614997675002, -17.99999999956958163, 5.204731250180315349 ) ) ;
#10431=CARTESIAN_POINT ( 'NONE',  ( 16.62983158437509346, -6.888301784570737496, -6.281987499819692289 ) ) ;
#10433=CARTESIAN_POINT ( 'NONE',  ( -7.500000000000002665, -4.022542205827308438E-17, 14.51130000000230602 ) ) ;
#10434=CARTESIAN_POINT ( 'NONE',  ( 11.17563879704982632, -2.222972771497745637, 16.78714100064743420 ) ) ;
#10441=CARTESIAN_POINT ( 'NONE',  ( -6.888301780572501976, 16.62983158603122291, 10.93823750018031404 ) ) ;
#10449=CARTESIAN_POINT ( 'NONE',  ( 0.000000000000000000, 0.000000000000000000, 40.00000000000000000 ) ) ;
#10451=EDGE_LOOP ( 'NONE', ( #20835, #19960 ) ) ;
#10457=CARTESIAN_POINT ( 'NONE',  ( -5.663308646854337880, 13.67243654778935991, 22.21997941884154315 ) ) ;
#10462=CARTESIAN_POINT ( 'NONE',  ( -18.00000000043040771, -3.580422610670021211, 16.39691875018031197 ) ) ;
#10467=CARTESIAN_POINT ( 'NONE',  ( 5.303300859536631329, 5.303300858261585482, 18.04567500018031012 ) ) ;
#10473=CARTESIAN_POINT ( 'NONE',  ( 6.888301784570727726, 16.62983158437509701, 10.21176250018031162 ) ) ;
#10480=CARTESIAN_POINT ( 'NONE',  ( -16.62983158437510411, 6.888301784570731279, 19.18511250018030978 ) ) ;
#10483=CARTESIAN_POINT ( 'NONE',  ( 4.248408730893249441, 6.358192987158595599, -4.258956249819687123 ) ) ;
#10485=EDGE_CURVE ( 'NONE', #11708, #15181, #8615, .T. ) ;
#10486=CARTESIAN_POINT ( 'NONE',  ( -9.474249098604506258, -6.330490856366290053, -15.07620350028680711 ) ) ;
#10490=CARTESIAN_POINT ( 'NONE',  ( -15.25966316918061771, 10.19618095414378622, -8.795356249819686667 ) ) ;
#10505=CARTESIAN_POINT ( 'NONE',  ( -1.491842756249031510, -7.499999999820660790, 3.024581250180311986 ) ) ;
#10507=CYLINDRICAL_SURFACE ( 'NONE', #13893, 2.649999999999998579 ) ;
#10516=CARTESIAN_POINT ( 'NONE',  ( -2.163827323447878234E-09, -18.00000000000000000, 4.910200000180314106 ) ) ;
#10530=CARTESIAN_POINT ( 'NONE',  ( 16.62983158603121936, 6.888301780572501976, -16.88511249981969442 ) ) ;
#10535=CARTESIAN_POINT ( 'NONE',  ( 1.343451552857795926E-09, 11.17563879731705789, -4.713640249352573086 ) ) ;
#10539=DIRECTION ( 'NONE',  ( -0.000000000000000000, -0.000000000000000000, 1.000000000000000000 ) ) ;
#10543=CARTESIAN_POINT ( 'NONE',  ( 3.580422614997668340, 17.99999999956958519, 2.396831250180312622 ) ) ;
#10551=CARTESIAN_POINT ( 'NONE',  ( 9.015937996181842420E-10, 7.500000000000007994, 13.70745000018031590 ) ) ;
#10557=CARTESIAN_POINT ( 'NONE',  ( -10.46442989202484242, 10.46442989454075700, -6.644083081158454362 ) ) ;
#10565=CARTESIAN_POINT ( 'NONE',  ( -16.62983158437509701, 6.888301784570728614, 7.855512500180310553 ) ) ;
#10572=ORIENTED_EDGE ( 'NONE', *, *, #13772, .T. ) ;
#10573=AXIS2_PLACEMENT_3D ( 'NONE', #6970, #17628, #3101 ) ;
#10577=CARTESIAN_POINT ( 'NONE',  ( -9.015947181032828388E-10, -7.500000000000002665, 2.730050000180308523 ) ) ;
#10578=CARTESIAN_POINT ( 'NONE',  ( -12.72792205982779556, 12.72792206288790773, -19.83042499981969087 ) ) ;
#10588=CARTESIAN_POINT ( 'NONE',  ( 12.72792205982779912, -12.72792206288791483, 15.06167500018031014 ) ) ;
#10591=CARTESIAN_POINT ( 'NONE',  ( 6.929096494179683319, 2.870125741905213079, 6.049637500180313765 ) ) ;
#10593=CARTESIAN_POINT ( 'NONE',  ( -9.015947181032835626E-10, -7.500000000000007994, 18.41995000018031803 ) ) ;
#10595=CARTESIAN_POINT ( 'NONE',  ( -11.17563879731704723, 1.343452237168308679E-09, -23.61760975028680321 ) ) ;
#10601=DIRECTION ( 'NONE',  ( -0.000000000000000000, -0.000000000000000000, -1.000000000000000000 ) ) ;
#10602=CARTESIAN_POINT ( 'NONE',  ( -15.25966316918061771, 10.19618095414378622, 0.6296437501803129333 ) ) ;
#10604=CIRCLE ( 'NONE', #11952, 2.649999999999999467 ) ;
#10616=VECTOR ( 'NONE', #8299, 1000.000000000000000 ) ;
#10619=DIRECTION ( 'NONE',  ( 1.000000000000000000, 0.000000000000000000, 0.000000000000000000 ) ) ;
#10622=CARTESIAN_POINT ( 'NONE',  ( -7.499999999820661678, 1.491842756249031288, -4.044168749819689879 ) ) ;
#10631=CARTESIAN_POINT ( 'NONE',  ( -3.580422610670018546, 18.00000000043041126, -0.09683124981968786738 ) ) ;
#10636=VERTEX_POINT ( 'NONE', #20803 ) ;
#10640=CARTESIAN_POINT ( 'NONE',  ( 0.000000000000000000, 0.000000000000000000, 43.00000000000000000 ) ) ;
#10647=CARTESIAN_POINT ( 'NONE',  ( -15.25966316918061416, 10.19618095414378445, -10.69995624981968874 ) ) ;
#10651=EDGE_CURVE ( 'NONE', #9351, #16482, #6178, .T. ) ;
#10652=CARTESIAN_POINT ( 'NONE',  ( -6.330490858644140850, -9.474249097082498849, -8.542546499352576816 ) ) ;
#10659=CARTESIAN_POINT ( 'NONE',  ( -15.25966316918061771, 10.19618095414378622, -18.22035624981969093 ) ) ;
#10661=LINE ( 'NONE', #2178, #8343 ) ;
#10675=CARTESIAN_POINT ( 'NONE',  ( -2.943691925285397470, 14.79893867793684059, -5.760489331158455961 ) ) ;
#10680=CARTESIAN_POINT ( 'NONE',  ( 10.19618095047497697, -15.25966317163202923, 13.45160625018031197 ) ) ;
#10692=CARTESIAN_POINT ( 'NONE',  ( -17.99999999999999645, 2.163826221265758470E-09, -21.00854999981969229 ) ) ;
#10693=EDGE_CURVE ( 'NONE', #8981, #1332, #17434, .T. ) ;
#10698=DIRECTION ( 'NONE',  ( 1.384478184788908018E-16, -1.611744734445712550E-26, -1.000000000000000000 ) ) ;
#10700=CARTESIAN_POINT ( 'NONE',  ( 17.99999999956958519, -3.580422614997676778, 14.17808125018031085 ) ) ;
#10707=CARTESIAN_POINT ( 'NONE',  ( 11.17563879731704723, -1.343450868547281106E-09, -28.33010975028681244 ) ) ;
#10712=CARTESIAN_POINT ( 'NONE',  ( 6.888301784570728614, 16.62983158437510056, -16.15863749981969377 ) ) ;
#10722=DIRECTION ( 'NONE',  ( 0.000000000000000000, 0.000000000000000000, 1.000000000000000000 ) ) ;
#10731=CARTESIAN_POINT ( 'NONE',  ( -4.248408729364575365, 6.358192988180014105, -21.71604374981968988 ) ) ;
#10740=CARTESIAN_POINT ( 'NONE',  ( 15.25966317163202746, 10.19618095047498407, -7.754643749819687848 ) ) ;
#10764=ADVANCED_FACE ( 'NONE', ( #14968 ), #14674, .F. ) ;
#10766=CARTESIAN_POINT ( 'NONE',  ( -15.25966316918061771, 10.19618095414378622, -8.795356249819686667 ) ) ;
#10777=CARTESIAN_POINT ( 'NONE',  ( 12.54593441562640876, -8.382925371439629458, -2.226114331158456139 ) ) ;
#10783=CARTESIAN_POINT ( 'NONE',  ( 16.62983158603121936, 6.888301780572501976, 1.964887500180308777 ) ) ;
#10785=DIRECTION ( 'NONE',  ( -1.000000000000000000, 0.000000000000000000, 0.000000000000000000 ) ) ;
#10795=CARTESIAN_POINT ( 'NONE',  ( -3.580422614997674557, -17.99999999956957808, -4.220268749819691578 ) ) ;
#10803=CARTESIAN_POINT ( 'NONE',  ( 6.888301784570730391, 16.62983158437510411, 2.691362500180309425 ) ) ;
#10805=CARTESIAN_POINT ( 'NONE',  ( 9.015937996181842420E-10, 7.500000000000007994, -14.56754999981968446 ) ) ;
#10807=CARTESIAN_POINT ( 'NONE',  ( -4.248408730893249441, -6.358192987158596488, 19.30354375018031732 ) ) ;
#10808=CARTESIAN_POINT ( 'NONE',  ( -5.663308650141535949, -13.67243654642774686, 13.06752058151907647 ) ) ;
#10813=CARTESIAN_POINT ( 'NONE',  ( 12.72792205982779734, -12.72792206288791128, -22.63832499981969093 ) ) ;
#10825=CARTESIAN_POINT ( 'NONE',  ( 9.474249098604504482, 6.330490856366291830, 17.91129649971319537 ) ) ;
#10833=CARTESIAN_POINT ( 'NONE',  ( 15.25966316918061416, -10.19618095414378622, -5.987456249819688381 ) ) ;
#10838=CARTESIAN_POINT ( 'NONE',  ( -5.303300859536632217, -5.303300858261584594, -5.516824999819692543 ) ) ;
#10839=CARTESIAN_POINT ( 'NONE',  ( 7.500000000000002665, -9.015933403756338579E-10, -27.90119999981969556 ) ) ;
#10845=CARTESIAN_POINT ( 'NONE',  ( -17.99999999999999645, 2.163826221265758470E-09, -21.00854999981969229 ) ) ;
#10849=VERTEX_POINT ( 'NONE', #5862 ) ;
#10855=CARTESIAN_POINT ( 'NONE',  ( -6.358192987158597376, 4.248408730893249441, -6.615206249819684636 ) ) ;
#10857=CARTESIAN_POINT ( 'NONE',  ( -16.62983158437510056, 6.888301784570729502, -18.51488749981968951 ) ) ;
#10871=CARTESIAN_POINT ( 'NONE',  ( -8.382925368423274293, 12.54593441764187745, 3.075448168841546703 ) ) ;
#10877=CARTESIAN_POINT ( 'NONE',  ( 12.72792206288790773, 12.72792205982779912, 10.80082500018031055 ) ) ;
#10878=DIRECTION ( 'NONE',  ( -0.000000000000000000, -0.000000000000000000, 1.000000000000000000 ) ) ;
#10888=CARTESIAN_POINT ( 'NONE',  ( 6.888301784570727726, 16.62983158437509701, -18.06323749981969584 ) ) ;
#10889=( BOUNDED_CURVE ( )  B_SPLINE_CURVE ( 2, ( #17349, #9292, #7910, #14389, #15753, #14181, #20831, #12897, #6315, #11297, #2714, #1141, #16375, #11713, #1668, #3438, #9804 ),
 .UNSPECIFIED., .F., .F. ) 
 B_SPLINE_CURVE_WITH_KNOTS ( ( 3, 2, 2, 2, 2, 2, 2, 2, 3 ),
 ( 0.9000000000038511638, 0.9125000000033697267, 0.9250000000028884006, 0.9375000000024069635, 0.9500000000019255264, 0.9625000000014442003, 0.9750000000009627632, 0.9875000000004814371, 1.000000000000000000 ),
 .UNSPECIFIED. ) 
 CURVE ( )  GEOMETRIC_REPRESENTATION_ITEM ( )  RATIONAL_B_SPLINE_CURVE ( ( 0.9999999999940800688, 0.9807852804091503618, 1.000000000000000000, 0.9807852804032304306, 1.000000000000000000, 0.9807852804032304306, 1.000000000000000000, 0.9807852804032304306, 1.000000000000000000, 0.9807852804032304306, 1.000000000000000000, 0.9807852804032304306, 1.000000000000000000, 0.9807852804032304306, 1.000000000000000000, 0.9807852804032304306, 1.000000000000000000 ) ) 
 REPRESENTATION_ITEM ( '' )  );
#10895=DIRECTION ( 'NONE',  ( -1.000000000000000000, 0.000000000000000000, 0.000000000000000000 ) ) ;
#10897=CIRCLE ( 'NONE', #6142, 2.649999999999999467 ) ;
#10899=CARTESIAN_POINT ( 'NONE',  ( -12.72792205982780089, 12.72792206288791128, 10.34917500018030978 ) ) ;
#10900=CARTESIAN_POINT ( 'NONE',  ( 2.870125741905214412, -6.929096494179682431, -10.44411249981968481 ) ) ;
#10904=CARTESIAN_POINT ( 'NONE',  ( -13.67243654778935102, -5.663308646854334327, 14.24564558151907789 ) ) ;
#10908=CARTESIAN_POINT ( 'NONE',  ( 16.62983158437509346, -6.888301784570739272, -23.22738749981969164 ) ) ;
#10923=CIRCLE ( 'NONE', #13631, 2.649999999999999467 ) ;
#10928=CARTESIAN_POINT ( 'NONE',  ( 7.499999999820660790, -1.491842756249031954, -27.60666874981969343 ) ) ;
#10936=CARTESIAN_POINT ( 'NONE',  ( 15.25966316918061416, -10.19618095414378622, -15.41245624981968732 ) ) ;
#10964=CARTESIAN_POINT ( 'NONE',  ( -12.72792205982779912, 12.72792206288790950, -8.500824999819686312 ) ) ;
#10971=ORIENTED_EDGE ( 'NONE', *, *, #1806, .F. ) ;
#10978=CARTESIAN_POINT ( 'NONE',  ( 1.779017513685136568E-09, 14.79893867758297610, -5.465958081158456494 ) ) ;
#10980=CARTESIAN_POINT ( 'NONE',  ( -7.500000000000004441, -1.491842754878798916, -14.05823124991221285 ) ) ;
#10985=CARTESIAN_POINT ( 'NONE',  ( -6.888301784570736608, -16.62983158437509346, 5.499262500180311264 ) ) ;
#10986=CARTESIAN_POINT ( 'NONE',  ( -2.870125741905210415, 6.929096494179677990, -21.42151249981969130 ) ) ;
#10993=CARTESIAN_POINT ( 'NONE',  ( -6.929096494179678878, -2.870125741905209971, 4.497237500180307990 ) ) ;
#10994=CARTESIAN_POINT ( 'NONE',  ( -16.62983158603121936, -6.888301780572499311, -21.59761249981969300 ) ) ;
#10996=CARTESIAN_POINT ( 'NONE',  ( -2.870125743571144028, -6.929096493489630859, -9.265987499819688722 ) ) ;
#11002=CARTESIAN_POINT ( 'NONE',  ( -16.62983158603122646, -6.888301780572501976, 8.581987500180309425 ) ) ;
#11003=CARTESIAN_POINT ( 'NONE',  ( -7.500000000179346316, -1.491842754445844355, -17.21833124981968766 ) ) ;
#11007=CARTESIAN_POINT ( 'NONE',  ( -12.54593441562640166, 8.382925371439625906, 15.71830183151907612 ) ) ;
#11014=CARTESIAN_POINT ( 'NONE',  ( -18.00000000043041126, -3.580422610670022543, -19.39848124981969235 ) ) ;
#11017=EDGE_LOOP ( 'NONE', ( #12400, #17577, #12163, #12667 ) ) ;
#11030=AXIS2_PLACEMENT_3D ( 'NONE', #19202, #6461, #1516 ) ;
#11032=CARTESIAN_POINT ( 'NONE',  ( 10.32494394706616347, -4.276731815070950127, -11.19332774935257468 ) ) ;
#11034=CARTESIAN_POINT ( 'NONE',  ( -6.929096493489625530, 2.870125743571138255, -22.59963749981969272 ) ) ;
#11035=CARTESIAN_POINT ( 'NONE',  ( 6.249999999999902300, -10.82531754730554496, 43.00000000000000000 ) ) ;
#11045=CARTESIAN_POINT ( 'NONE',  ( 17.99999999956958163, -3.580422614997676334, -16.00151874981968803 ) ) ;
#11054=CARTESIAN_POINT ( 'NONE',  ( 1.491842756249029289, 7.499999999820664343, -1.687918749819692588 ) ) ;
#11060=CARTESIAN_POINT ( 'NONE',  ( 6.250000000000054179, 10.82531754730546147, -43.00000000000000000 ) ) ;
#11063=CARTESIAN_POINT ( 'NONE',  ( 6.929096493489625530, -2.870125743571142252, 10.38786250018030799 ) ) ;
#11071=CARTESIAN_POINT ( 'NONE',  ( -6.929096494179684207, -2.870125741905212635, 1.337137500180316074 ) ) ;
#11072=ORIENTED_EDGE ( 'NONE', *, *, #19926, .T. ) ;
#11076=CARTESIAN_POINT ( 'NONE',  ( -16.62983158437510056, 6.888301784570729502, -9.089887499819687022 ) ) ;
#11091=CARTESIAN_POINT ( 'NONE',  ( -11.17563879704982988, 2.222972771497744748, 21.49964100064742922 ) ) ;
#11093=CARTESIAN_POINT ( 'NONE',  ( 6.929096493489625530, -2.870125743571142252, -17.88713749981969414 ) ) ;
#11115=CARTESIAN_POINT ( 'NONE',  ( 10.19618095047498052, -15.25966317163203456, -12.91879374981968986 ) ) ;
#11116=CARTESIAN_POINT ( 'NONE',  ( -5.303300858261589035, 5.303300859536635770, -15.74567499981968588 ) ) ;
#11119=CARTESIAN_POINT ( 'NONE',  ( -8.382925368423267187, 12.54593441764186856, 16.30736433151907860 ) ) ;
#11121=ORIENTED_EDGE ( 'NONE', *, *, #2175, .T. ) ;
#11123=CARTESIAN_POINT ( 'NONE',  ( -3.580422610670018546, 18.00000000043041126, -17.04223124981968951 ) ) ;
#11131=ORIENTED_EDGE ( 'NONE', *, *, #504, .T. ) ;
#11138=CARTESIAN_POINT ( 'NONE',  ( -7.902369976724401113, 7.902369978624329327, -5.891765249352570954 ) ) ;
#11139=CARTESIAN_POINT ( 'NONE',  ( -10.32494394706615815, 4.276731815070940357, 14.67145274971319857 ) ) ;
#11147=CARTESIAN_POINT ( 'NONE',  ( -18.00000000000000000, 2.163826221265758884E-09, -21.00854999981968874 ) ) ;
#11160=EDGE_CURVE ( 'NONE', #20507, #10032, #20151, .T. ) ;
#11161=ADVANCED_FACE ( 'NONE', ( #14634 ), #11458, .T. ) ;
#11164=CARTESIAN_POINT ( 'NONE',  ( -9.850000000000006750, 0.000000000000000000, 43.00000000000000000 ) ) ;
#11166=CARTESIAN_POINT ( 'NONE',  ( 4.248408729364579806, -6.358192988180021210, -1.313643749819685347 ) ) ;
#11172=CARTESIAN_POINT ( 'NONE',  ( 17.99999999956958163, -3.580422614997676334, -23.52191874981969022 ) ) ;
#11187=CARTESIAN_POINT ( 'NONE',  ( 12.54593441764187567, 8.382925368423276069, -13.41830183115846076 ) ) ;
#11190=EDGE_CURVE ( 'NONE', #13652, #10636, #2217, .T. ) ;
#11206=CARTESIAN_POINT ( 'NONE',  ( 12.72792205982779379, -12.72792206288790950, -24.54292499981969300 ) ) ;
#11208=CARTESIAN_POINT ( 'NONE',  ( 4.248408729364579806, -6.358192988180021210, -10.73864374981968517 ) ) ;
#11212=CARTESIAN_POINT ( 'NONE',  ( 6.888301784570730391, 16.62983158437510411, -16.15863749981969733 ) ) ;
#11213=CARTESIAN_POINT ( 'NONE',  ( 6.358192988180014993, 4.248408729364578917, 8.915206250180309766 ) ) ;
#11216=CARTESIAN_POINT ( 'NONE',  ( 13.67243654778934925, 5.663308646854335215, 0.1081455815190729419 ) ) ;
#11231=ORIENTED_EDGE ( 'NONE', *, *, #9500, .F. ) ;
#11237=CARTESIAN_POINT ( 'NONE',  ( 4.276731812588570492, -10.32494394809439697, -19.44020274935257220 ) ) ;
#11238=AXIS2_PLACEMENT_3D ( 'NONE', #9102, #17261, #10895 ) ;
#11239=CARTESIAN_POINT ( 'NONE',  ( -1.343452921478823292E-09, -11.17563879731704723, 2.301140249713198749 ) ) ;
#11247=CARTESIAN_POINT ( 'NONE',  ( -16.62983158603122291, -6.888301780572501087, 8.581987500180312978 ) ) ;
#11258=CIRCLE ( 'NONE', #4823, 2.649999999999999467 ) ;
#11264=CARTESIAN_POINT ( 'NONE',  ( -7.500000000000000000, 0.000000000000000000, 40.00000000000000000 ) ) ;
#11268=CARTESIAN_POINT ( 'NONE',  ( 1.491842754445843688, -7.500000000179346316, -0.7245812498196841922 ) ) ;
#11276=CARTESIAN_POINT ( 'NONE',  ( -12.50000000000000533, 0.000000000000000000, 43.00000000000000000 ) ) ;
#11291=CARTESIAN_POINT ( 'NONE',  ( -1.779019326032424922E-09, -14.79893867758297610, -19.60345808115846111 ) ) ;
#11293=CARTESIAN_POINT ( 'NONE',  ( 7.500000000000000888, 4.207617034106124418E-15, 0.3738000000023073421 ) ) ;
#11297=CARTESIAN_POINT ( 'NONE',  ( 1.491842754445842578, -7.500000000179340987, -25.83948124981969485 ) ) ;
#11301=CARTESIAN_POINT ( 'NONE',  ( 12.72792206288790950, 12.72792205982780089, 22.13042500018031689 ) ) ;
#11305=VECTOR ( 'NONE', #17619, 1000.000000000000000 ) ;
#11315=CARTESIAN_POINT ( 'NONE',  ( 6.358192988180019434, 4.248408729364581582, -3.669893749819685969 ) ) ;
#11323=CARTESIAN_POINT ( 'NONE',  ( -2.163827323447878648E-09, -18.00000000000000355, -21.46019999981969306 ) ) ;
#11329=CARTESIAN_POINT ( 'NONE',  ( -13.67243654778935102, -5.663308646854334327, -14.02935441848092957 ) ) ;
#11334=CARTESIAN_POINT ( 'NONE',  ( 6.358192988180019434, 4.248408729364581582, 24.60510625018031661 ) ) ;
#11351=CARTESIAN_POINT ( 'NONE',  ( 9.474249097082498849, -6.330490858644140850, -20.32379649935257504 ) ) ;
#11352=CARTESIAN_POINT ( 'NONE',  ( -11.17563879758427525, -2.222972768810838051, 4.362858999713199459 ) ) ;
#11358=CARTESIAN_POINT ( 'NONE',  ( 3.580422614997668340, 17.99999999956958519, 11.82183125018031511 ) ) ;
#11375=CARTESIAN_POINT ( 'NONE',  ( 9.015937996181834148E-10, 7.500000000000000888, 16.86755000018031225 ) ) ;
#11388=ORIENTED_EDGE ( 'NONE', *, *, #15535, .F. ) ;
#11393=CIRCLE ( 'NONE', #11723, 17.50000000000000355 ) ;
#11394=CARTESIAN_POINT ( 'NONE',  ( 7.574999999999881162, -13.12028486733431976, -43.00000000000000000 ) ) ;
#11395=CARTESIAN_POINT ( 'NONE',  ( -2.222972771497745192, -11.17563879704982632, 19.14339100064742993 ) ) ;
#11406=CARTESIAN_POINT ( 'NONE',  ( -9.850000000000006750, 0.000000000000000000, -40.00000000000000000 ) ) ;
#11417=AXIS2_PLACEMENT_3D ( 'NONE', #6440, #9644, #16106 ) ;
#11423=CARTESIAN_POINT ( 'NONE',  ( 3.580422610670021211, -18.00000000043041481, -21.75473124981969164 ) ) ;
#11426=ORIENTED_EDGE ( 'NONE', *, *, #19926, .F. ) ;
#11429=CARTESIAN_POINT ( 'NONE',  ( 4.248408730893246776, 6.358192987158592047, 8.326143750180307279 ) ) ;
#11431=CARTESIAN_POINT ( 'NONE',  ( 1.779017513685135741E-09, 14.79893867758296544, -11.08404191848092779 ) ) ;
#11454=SURFACE_STYLE_FILL_AREA ( #14120 ) ;
#11455=CARTESIAN_POINT ( 'NONE',  ( 4.248408729364579806, -6.358192988180021210, 17.53635625018031519 ) ) ;
#11456=CARTESIAN_POINT ( 'NONE',  ( 4.276731815070940357, 10.32494394706615815, 7.602702749713199815 ) ) ;
#11458=CYLINDRICAL_SURFACE ( 'NONE', #10345, 7.500000000000000000 ) ;
#11461=CARTESIAN_POINT ( 'NONE',  ( 10.19618095047497874, -15.25966317163203279, 5.931206250180311557 ) ) ;
#11474=CARTESIAN_POINT ( 'NONE',  ( -5.303300859536631329, -5.303300858261583706, 3.908175000180312164 ) ) ;
#11481=ORIENTED_EDGE ( 'NONE', *, *, #7210, .T. ) ;
#11482=CARTESIAN_POINT ( 'NONE',  ( 3.580422610670020322, -18.00000000043041126, 14.04066875018031446 ) ) ;
#11491=CARTESIAN_POINT ( 'NONE',  ( 5.663308646854342321, -13.67243654778935635, -20.19252058115845827 ) ) ;
#11512=CARTESIAN_POINT ( 'NONE',  ( -17.99999999956958874, 3.580422614997675002, -18.80941874981969164 ) ) ;
#11514=VECTOR ( 'NONE', #10539, 1000.000000000000000 ) ;
#11516=( LENGTH_UNIT ( ) NAMED_UNIT ( * ) SI_UNIT ( .MILLI., .METRE. ) );
#11517=CARTESIAN_POINT ( 'NONE',  ( -14.79893867793683349, -2.943691925285398359, -4.309823168480927613 ) ) ;
#11519=AXIS2_PLACEMENT_3D ( 'NONE', #19943, #7335, #13501 ) ;
#11542=CARTESIAN_POINT ( 'NONE',  ( -6.358192988180021210, -4.248408729364580694, 10.46760625018031376 ) ) ;
#11543=CARTESIAN_POINT ( 'NONE',  ( -2.222972768810836275, 11.17563879758427525, -2.705891000286804182 ) ) ;
#11551=CARTESIAN_POINT ( 'NONE',  ( -10.19618095414378622, -15.25966316918061416, 17.12339375018031262 ) ) ;
#11565=ADVANCED_FACE ( 'NONE', ( #5248 ), #490, .T. ) ;
#11572=CARTESIAN_POINT ( 'NONE',  ( -9.015947181032828388E-10, -7.500000000000000888, 12.15505000018031367 ) ) ;
#11596=CARTESIAN_POINT ( 'NONE',  ( 2.222972771497741640, 11.17563879704982988, 5.005891000647428868 ) ) ;
#11606=CARTESIAN_POINT ( 'NONE',  ( -18.00000000043041126, -3.580422610670022099, 18.30151875018031760 ) ) ;
#11609=VECTOR ( 'NONE', #9064, 1000.000000000000000 ) ;
#11621=CARTESIAN_POINT ( 'NONE',  ( -8.382925368423274293, 12.54593441764187745, 21.92544816884154457 ) ) ;
#11627=CARTESIAN_POINT ( 'NONE',  ( 14.79893867722909917, -2.943691928843437111, 0.9917393315190744518 ) ) ;
#11630=CARTESIAN_POINT ( 'NONE',  ( 3.600000000000054712, 10.82531754730546147, 43.00000000000000000 ) ) ;
#11650=CARTESIAN_POINT ( 'NONE',  ( -6.358192988180021210, -4.248408729364580694, 19.89260625018031803 ) ) ;
#11653=CARTESIAN_POINT ( 'NONE',  ( -6.330490856366290053, 9.474249098604506258, 6.130046499713198926 ) ) ;
#11660=CARTESIAN_POINT ( 'NONE',  ( -6.888301780572501976, 16.62983158603122291, 10.93823750018031404 ) ) ;
#11677=CARTESIAN_POINT ( 'NONE',  ( -7.499999999820661678, 1.491842756249031288, 5.380831250180311720 ) ) ;
#11688=CARTESIAN_POINT ( 'NONE',  ( 10.19618095047497874, -15.25966317163203279, 13.45160625018031553 ) ) ;
#11697=( BOUNDED_SURFACE ( )  B_SPLINE_SURFACE ( 1, 2, ( 
 ( #11791, #5109, #18254, #17859, #16159, #1942, #14668, #8400, #346, #1652, #13183, #142, #8100, #6492, #6799, #12978, #6595, #19431, #13283, #4915, #13081, #19537, #19742, #9887, #5020, #11482, #5223, #11688, #16355, #765, #7016, #15183, #15498, #16769, #5521, #20037, #18357, #15391, #17090, #10198, #13700, #567, #20361, #12000, #7432, #12208, #18467, #8805, #9038, #13814, #10311, #15277, #7329, #20258, #3933, #10419, #10516, #16880, #20145, #13912, #989, #5634, #5845, #13496, #12323, #19938, #16660, #12111, #4147, #16973, #18676, #15080, #7218, #10631, #2573, #2355, #2457, #18579, #660, #5416, #7109, #5735, #4039, #8922, #13589, #875, #3720, #2150, #8607, #11887, #3826, #2255, #8715, #10833, #7971, #1312, #7539, #20894, #2993, #10740, #12531, #9138, #6057, #2776, #1408, #2883, #4581, #2677, #18994, #14026, #9244, #16022, #19108, #7859, #20474, #4367, #6268, #4468, #9348, #3087, #14340, #17302, #15813, #20787, #12755, #10936, #20581, #11045, #17416, #7757, #14446, #9552, #20674, #1521, #1094, #6374, #5951, #17203, #6158, #19209, #17522, #4686, #15595, #14229, #11147, #17616, #12646, #9452, #15912, #15708, #12429, #1203, #18789, #4259, #18901, #7649, #14130, #8468, #8166, #6679, #13158 ),
 ( #16326, #1626, #14950, #18024, #4780, #6573, #3198, #115, #17832, #16426, #17929, #19608, #17725, #13052, #8078, #3305, #10077, #5085, #1915, #14547, #19404, #11551, #19709, #3490, #16534, #428, #3392, #9962, #12952, #322, #13, #6465, #19297, #5190, #1816, #6776, #4892, #3600, #8270, #11358, #221, #8376, #11660, #9858, #9765, #2018, #12853, #14743, #13256, #16230, #11247, #14847, #9667, #1715, #18130, #16132, #19507, #14637, #4996, #11461, #5494, #18333, #3906, #10172, #3799, #18648, #19916, #8685, #2224, #538, #18554, #20235, #13367, #16855, #3698, #2548, #15158, #10602, #20011, #2328, #8580, #5707, #9009, #12181, #637, #10389, #11974, #2429, #7084, #15055, #850, #2122, #19814, #13566, #16947, #18443, #16743, #739, #8781, #15254, #5394, #13675, #6985, #13473, #7191, #17064, #16634, #4010, #5297, #10490, #11769, #8895, #18234, #15476, #20124, #5603, #11863, #13786, #10283, #7303, #12084, #15367, #4117, #6881, #4662, #6036, #13885, #12508, #14104, #20451, #2749, #3062, #5931, #7407, #10712, #7735, #1384, #11123, #18972, #15569, #2856, #6241, #20330, #15888, #4442, #11014, #9322, #12402, #18874, #5816, #2658, #1063, #9215, #20557, #7510, #4346, #10813, #7830, #10908, #17277, #17491 ) ),
 .UNSPECIFIED., .F., .F., .T. ) 
 B_SPLINE_SURFACE_WITH_KNOTS ( ( 2, 2 ),
 ( 3, 2, 2, 2, 2, 2, 2, 2, 2, 2, 2, 2, 2, 2, 2, 2, 2, 2, 2, 2, 2, 2, 2, 2, 2, 2, 2, 2, 2, 2, 2, 2, 2, 2, 2, 2, 2, 2, 2, 2, 2, 2, 2, 2, 2, 2, 2, 2, 2, 2, 2, 2, 2, 2, 2, 2, 2, 2, 2, 2, 2, 2, 2, 2, 2, 2, 2, 2, 2, 2, 2, 2, 2, 2, 2, 2, 2, 2, 2, 2, 3 ),
 ( 0.000000000000000000, 1.000000000000000000 ),
 ( 0.000000000000000000, 0.01250000000000000069, 0.02500000000000000139, 0.03749999999999999861, 0.05000000000000000278, 0.06250000000000000000, 0.07499999999999999722, 0.08749999999999999445, 0.1000000000000000056, 0.1125000000000000028, 0.1250000000000000000, 0.1375000000000000111, 0.1499999999999999944, 0.1625000000000000056, 0.1749999999999999889, 0.1875000000000000000, 0.2000000000000000111, 0.2124999999999999944, 0.2250000000000000056, 0.2374999999999999889, 0.2500000000000000000, 0.2625000000000000111, 0.2750000000000000222, 0.2874999999999999778, 0.2999999999999999889, 0.3125000000000000000, 0.3250000000000000111, 0.3375000000000000222, 0.3499999999999999778, 0.3624999999999999889, 0.3750000000000000000, 0.3875000000000000111, 0.4000000000000000222, 0.4124999999999999778, 0.4249999999999999889, 0.4375000000000000000, 0.4500000000000000111, 0.4625000000000000222, 0.4749999999999999778, 0.4874999999999999889, 0.5000000000000000000, 0.5124999999999999556, 0.5250000000000000222, 0.5374999999999999778, 0.5500000000000000444, 0.5625000000000000000, 0.5749999999999999556, 0.5875000000000000222, 0.5999999999999999778, 0.6125000000000000444, 0.6250000000000000000, 0.6374999999999999556, 0.6500000000000000222, 0.6624999999999999778, 0.6750000000000000444, 0.6875000000000000000, 0.6999999999999999556, 0.7125000000000000222, 0.7249999999999999778, 0.7375000000000000444, 0.7500000000000000000, 0.7624999999999999556, 0.7750000000000000222, 0.7874999999999999778, 0.8000000000000000444, 0.8125000000000000000, 0.8249999999999999556, 0.8375000000000000222, 0.8499999999999999778, 0.8625000000000000444, 0.8750000000000000000, 0.8874999999999999556, 0.9000000000000000222, 0.9124999999999999778, 0.9250000000000000444, 0.9375000000000000000, 0.9499999999999999556, 0.9625000000000000222, 0.9749999999999999778, 0.9875000000000000444, 1.000000000000000000 ),
 .UNSPECIFIED. ) 
 GEOMETRIC_REPRESENTATION_ITEM ( )  RATIONAL_B_SPLINE_SURFACE ( (
 ( 1.000000000000000000, 0.9807852804032304306, 1.000000000000000000, 0.9807852804032304306, 1.000000000000000000, 0.9807852804032304306, 1.000000000000000000, 0.9807852804032304306, 1.000000000000000000, 0.9807852804032304306, 1.000000000000000000, 0.9807852804032304306, 1.000000000000000000, 0.9807852804032304306, 1.000000000000000000, 0.9807852804032304306, 1.000000000000000000, 0.9807852804032304306, 1.000000000000000000, 0.9807852804032304306, 1.000000000000000000, 0.9807852804032304306, 1.000000000000000000, 0.9807852804032304306, 1.000000000000000000, 0.9807852804032304306, 1.000000000000000000, 0.9807852804032304306, 1.000000000000000000, 0.9807852804032304306, 1.000000000000000000, 0.9807852804032304306, 1.000000000000000000, 0.9807852804032304306, 1.000000000000000000, 0.9807852804032304306, 1.000000000000000000, 0.9807852804032304306, 1.000000000000000000, 0.9807852804032304306, 1.000000000000000000, 0.9807852804032304306, 1.000000000000000000, 0.9807852804032304306, 1.000000000000000000, 0.9807852804032304306, 1.000000000000000000, 0.9807852804032304306, 1.000000000000000000, 0.9807852804032304306, 1.000000000000000000, 0.9807852804032304306, 1.000000000000000000, 0.9807852804032304306, 1.000000000000000000, 0.9807852804032304306, 1.000000000000000000, 0.9807852804032304306, 1.000000000000000000, 0.9807852804032304306, 1.000000000000000000, 0.9807852804032304306, 1.000000000000000000, 0.9807852804032304306, 1.000000000000000000, 0.9807852804032304306, 1.000000000000000000, 0.9807852804032304306, 1.000000000000000000, 0.9807852804032304306, 1.000000000000000000, 0.9807852804032304306, 1.000000000000000000, 0.9807852804032304306, 1.000000000000000000, 0.9807852804032304306, 1.000000000000000000, 0.9807852804032304306, 1.000000000000000000, 0.9807852804032304306, 1.000000000000000000, 0.9807852804032304306, 1.000000000000000000, 0.9807852804032304306, 1.000000000000000000, 0.9807852804032304306, 1.000000000000000000, 0.9807852804032304306, 1.000000000000000000, 0.9807852804032304306, 1.000000000000000000, 0.9807852804032304306, 1.000000000000000000, 0.9807852804032304306, 1.000000000000000000, 0.9807852804032304306, 1.000000000000000000, 0.9807852804032304306, 1.000000000000000000, 0.9807852804032304306, 1.000000000000000000, 0.9807852804032304306, 1.000000000000000000, 0.9807852804032304306, 1.000000000000000000, 0.9807852804032304306, 1.000000000000000000, 0.9807852804032304306, 1.000000000000000000, 0.9807852804032304306, 1.000000000000000000, 0.9807852804032304306, 1.000000000000000000, 0.9807852804032304306, 1.000000000000000000, 0.9807852804032304306, 1.000000000000000000, 0.9807852804032304306, 1.000000000000000000, 0.9807852804032304306, 1.000000000000000000, 0.9807852804032304306, 1.000000000000000000, 0.9807852804032304306, 1.000000000000000000, 0.9807852804032304306, 1.000000000000000000, 0.9807852804032304306, 1.000000000000000000, 0.9807852804032304306, 1.000000000000000000, 0.9807852804032304306, 1.000000000000000000, 0.9807852804032304306, 1.000000000000000000, 0.9807852804032304306, 1.000000000000000000, 0.9807852804032304306, 1.000000000000000000, 0.9807852804032304306, 1.000000000000000000, 0.9807852804032304306, 1.000000000000000000, 0.9807852804032304306, 1.000000000000000000, 0.9807852804032304306, 1.000000000000000000, 0.9807852804032304306, 1.000000000000000000, 0.9807852804032304306, 1.000000000000000000, 0.9807852804032304306, 1.000000000000000000, 0.9807852804032304306, 1.000000000000000000, 0.9807852804032304306, 1.000000000000000000, 0.9807852804032304306, 1.000000000000000000, 0.9807852804032304306, 1.000000000000000000),
 ( 1.000000000000000000, 0.9807852804032304306, 1.000000000000000000, 0.9807852804032304306, 1.000000000000000000, 0.9807852804032304306, 1.000000000000000000, 0.9807852804032304306, 1.000000000000000000, 0.9807852804032304306, 1.000000000000000000, 0.9807852804032304306, 1.000000000000000000, 0.9807852804032304306, 1.000000000000000000, 0.9807852804032304306, 1.000000000000000000, 0.9807852804032304306, 1.000000000000000000, 0.9807852804032304306, 1.000000000000000000, 0.9807852804032304306, 1.000000000000000000, 0.9807852804032304306, 1.000000000000000000, 0.9807852804032304306, 1.000000000000000000, 0.9807852804032304306, 1.000000000000000000, 0.9807852804032304306, 1.000000000000000000, 0.9807852804032304306, 1.000000000000000000, 0.9807852804032304306, 1.000000000000000000, 0.9807852804032304306, 1.000000000000000000, 0.9807852804032304306, 1.000000000000000000, 0.9807852804032304306, 1.000000000000000000, 0.9807852804032304306, 1.000000000000000000, 0.9807852804032304306, 1.000000000000000000, 0.9807852804032304306, 1.000000000000000000, 0.9807852804032304306, 1.000000000000000000, 0.9807852804032304306, 1.000000000000000000, 0.9807852804032304306, 1.000000000000000000, 0.9807852804032304306, 1.000000000000000000, 0.9807852804032304306, 1.000000000000000000, 0.9807852804032304306, 1.000000000000000000, 0.9807852804032304306, 1.000000000000000000, 0.9807852804032304306, 1.000000000000000000, 0.9807852804032304306, 1.000000000000000000, 0.9807852804032304306, 1.000000000000000000, 0.9807852804032304306, 1.000000000000000000, 0.9807852804032304306, 1.000000000000000000, 0.9807852804032304306, 1.000000000000000000, 0.9807852804032304306, 1.000000000000000000, 0.9807852804032304306, 1.000000000000000000, 0.9807852804032304306, 1.000000000000000000, 0.9807852804032304306, 1.000000000000000000, 0.9807852804032304306, 1.000000000000000000, 0.9807852804032304306, 1.000000000000000000, 0.9807852804032304306, 1.000000000000000000, 0.9807852804032304306, 1.000000000000000000, 0.9807852804032304306, 1.000000000000000000, 0.9807852804032304306, 1.000000000000000000, 0.9807852804032304306, 1.000000000000000000, 0.9807852804032304306, 1.000000000000000000, 0.9807852804032304306, 1.000000000000000000, 0.9807852804032304306, 1.000000000000000000, 0.9807852804032304306, 1.000000000000000000, 0.9807852804032304306, 1.000000000000000000, 0.9807852804032304306, 1.000000000000000000, 0.9807852804032304306, 1.000000000000000000, 0.9807852804032304306, 1.000000000000000000, 0.9807852804032304306, 1.000000000000000000, 0.9807852804032304306, 1.000000000000000000, 0.9807852804032304306, 1.000000000000000000, 0.9807852804032304306, 1.000000000000000000, 0.9807852804032304306, 1.000000000000000000, 0.9807852804032304306, 1.000000000000000000, 0.9807852804032304306, 1.000000000000000000, 0.9807852804032304306, 1.000000000000000000, 0.9807852804032304306, 1.000000000000000000, 0.9807852804032304306, 1.000000000000000000, 0.9807852804032304306, 1.000000000000000000, 0.9807852804032304306, 1.000000000000000000, 0.9807852804032304306, 1.000000000000000000, 0.9807852804032304306, 1.000000000000000000, 0.9807852804032304306, 1.000000000000000000, 0.9807852804032304306, 1.000000000000000000, 0.9807852804032304306, 1.000000000000000000, 0.9807852804032304306, 1.000000000000000000, 0.9807852804032304306, 1.000000000000000000, 0.9807852804032304306, 1.000000000000000000, 0.9807852804032304306, 1.000000000000000000, 0.9807852804032304306, 1.000000000000000000, 0.9807852804032304306, 1.000000000000000000, 0.9807852804032304306, 1.000000000000000000, 0.9807852804032304306, 1.000000000000000000) ) ) 
 REPRESENTATION_ITEM ( '' )  SURFACE ( )  );
#11703=ADVANCED_FACE ( 'NONE', ( #3346 ), #9807, .F. ) ;
#11707=CARTESIAN_POINT ( 'NONE',  ( 9.474249097082498849, -6.330490858644140850, 7.951203500647429756 ) ) ;
#11708=VERTEX_POINT ( 'NONE', #11406 ) ;
#11713=CARTESIAN_POINT ( 'NONE',  ( 6.358192987158592047, -4.248408730893246776, -27.01760624981969627 ) ) ;
#11715=CARTESIAN_POINT ( 'NONE',  ( -12.72792205982779912, 12.72792206288790950, 10.34917500018031333 ) ) ;
#11721=ORIENTED_EDGE ( 'NONE', *, *, #8285, .F. ) ;
#11723=AXIS2_PLACEMENT_3D ( 'NONE', #5574, #18417, #8655 ) ;
#11730=CARTESIAN_POINT ( 'NONE',  ( -13.67243654642775574, 5.663308650141533285, 11.61685441884154812 ) ) ;
#11737=CARTESIAN_POINT ( 'NONE',  ( -2.943691925285395694, 14.79893867793683349, -20.80357316848093063 ) ) ;
#11743=CARTESIAN_POINT ( 'NONE',  ( -1.491842754445841690, 7.500000000179340987, 16.57301875018031012 ) ) ;
#11748=CARTESIAN_POINT ( 'NONE',  ( 15.25966317163202568, 10.19618095047498230, 11.09535625018031091 ) ) ;
#11758=CARTESIAN_POINT ( 'NONE',  ( 3.580422610670021211, -18.00000000043041481, 15.94526875018031298 ) ) ;
#11760=CARTESIAN_POINT ( 'NONE',  ( -5.303300859536636658, -5.303300858261589035, -8.676924999819688011 ) ) ;
#11762=CARTESIAN_POINT ( 'NONE',  ( -7.902369978624323110, -7.902369976724391343, -15.37073475028680569 ) ) ;
#11769=CARTESIAN_POINT ( 'NONE',  ( -16.62983158437510056, 6.888301784570729502, -9.089887499819687022 ) ) ;
#11783=CARTESIAN_POINT ( 'NONE',  ( 1.491842756249028845, 7.499999999820661678, 17.16208125018031438 ) ) ;
#11788=ORIENTED_EDGE ( 'NONE', *, *, #9485, .T. ) ;
#11789=DIRECTION ( 'NONE',  ( -0.000000000000000000, -0.000000000000000000, -1.000000000000000000 ) ) ;
#11791=CARTESIAN_POINT ( 'NONE',  ( 18.00000000000000000, -2.163824016901520184E-09, 21.40395000018031624 ) ) ;
#11794=DIRECTION ( 'NONE',  ( 1.000000000000000000, 0.000000000000000000, 0.000000000000000000 ) ) ;
#11802=CARTESIAN_POINT ( 'NONE',  ( -12.72792205982779556, 12.72792206288790773, -10.40542499981968838 ) ) ;
#11807=CARTESIAN_POINT ( 'NONE',  ( 11.17563879731705789, -1.343450868547281933E-09, 16.49260975064743562 ) ) ;
#11814=CARTESIAN_POINT ( 'NONE',  ( 15.25966317163202746, 10.19618095047498407, 3.574956250180311379 ) ) ;
#11818=EDGE_CURVE ( 'NONE', #16910, #8415, #10661, .T. ) ;
#11821=EDGE_LOOP ( 'NONE', ( #667, #15133, #15039, #17703 ) ) ;
#11829=CARTESIAN_POINT ( 'NONE',  ( -5.663308650141539502, -13.67243654642775574, 18.68560441884154599 ) ) ;
#11835=CARTESIAN_POINT ( 'NONE',  ( -17.99999999956958163, 3.580422614997673669, 16.98598125018030913 ) ) ;
#11845=CARTESIAN_POINT ( 'NONE',  ( 17.99999999956957808, -3.580422614997675446, 2.848481250180310287 ) ) ;
#11853=EDGE_CURVE ( 'NONE', #20507, #14958, #12135, .T. ) ;
#11855=CARTESIAN_POINT ( 'NONE',  ( -4.248408729364580694, 6.358192988180020322, -6.026143749819683038 ) ) ;
#11857=CARTESIAN_POINT ( 'NONE',  ( 7.902369976724389566, -7.902369978624323110, -17.72698475028679965 ) ) ;
#11861=CARTESIAN_POINT ( 'NONE',  ( 0.000000000000000000, 0.000000000000000000, -43.00000000000000000 ) ) ;
#11863=CARTESIAN_POINT ( 'NONE',  ( -12.72792206288791128, -12.72792205982779912, -10.85707499981969093 ) ) ;
#11871=AXIS2_PLACEMENT_3D ( 'NONE', #8474, #14748, #12957 ) ;
#11872=EDGE_LOOP ( 'NONE', ( #9549, #12370, #14586, #13168 ) ) ;
#11879=CARTESIAN_POINT ( 'NONE',  ( -5.303300858261583706, 5.303300859536630441, -3.160574999819688369 ) ) ;
#11887=CARTESIAN_POINT ( 'NONE',  ( 3.580422610670020322, -18.00000000043041126, -4.809331249819685183 ) ) ;
#11897=CARTESIAN_POINT ( 'NONE',  ( 6.358192988180014993, 4.248408729364578917, -9.934793749819693431 ) ) ;
#11898=CARTESIAN_POINT ( 'NONE',  ( 3.580422614997667896, 17.99999999956958163, -8.932768749819693710 ) ) ;
#11902=CARTESIAN_POINT ( 'NONE',  ( -10.32494394706616703, 4.276731815070943910, 12.36917225064743242 ) ) ;
#11912=CARTESIAN_POINT ( 'NONE',  ( 15.25966316918061416, -10.19618095414378622, 14.76714375018031333 ) ) ;
#11928=CARTESIAN_POINT ( 'NONE',  ( 14.79893867758297610, -1.779016607511492805E-09, 15.74029191884154599 ) ) ;
#11930=EDGE_LOOP ( 'NONE', ( #18420, #2779, #16134, #9475 ) ) ;
#11934=( BOUNDED_CURVE ( )  B_SPLINE_CURVE ( 2, ( #15755, #12696, #7596, #17570, #9295, #14073, #6007, #20525, #12478, #17461, #10986, #15959, #1256, #2935, #1460, #5781, #12257 ),
 .UNSPECIFIED., .F., .T. ) 
 B_SPLINE_CURVE_WITH_KNOTS ( ( 3, 2, 2, 2, 2, 2, 2, 2, 3 ),
 ( 0.8000000000038511860, 0.8125000000038511416, 0.8250000000038510972, 0.8375000000038511638, 0.8500000000038511194, 0.8625000000038511860, 0.8750000000038511416, 0.8875000000038510972, 0.9000000000038511638 ),
 .UNSPECIFIED. ) 
 CURVE ( )  GEOMETRIC_REPRESENTATION_ITEM ( )  RATIONAL_B_SPLINE_CURVE ( ( 0.9999999999940800688, 0.9807852804091503618, 1.000000000000000000, 0.9807852804032304306, 1.000000000000000000, 0.9807852804032304306, 1.000000000000000000, 0.9807852804032304306, 1.000000000000000000, 0.9807852804032304306, 1.000000000000000000, 0.9807852804032304306, 1.000000000000000000, 0.9807852804032304306, 1.000000000000000000, 0.9807852803973104994, 1.000000000005919931 ) ) 
 REPRESENTATION_ITEM ( '' )  );
#11937=CARTESIAN_POINT ( 'NONE',  ( 17.99999999999999645, -2.163824016901520184E-09, 21.40395000018031268 ) ) ;
#11938=EDGE_CURVE ( 'NONE', #16003, #17243, #17070, .T. ) ;
#11942=ORIENTED_EDGE ( 'NONE', *, *, #14282, .T. ) ;
#11950=CARTESIAN_POINT ( 'NONE',  ( -6.888301780572500199, 16.62983158603121936, 9.033637500180310198 ) ) ;
#11952=AXIS2_PLACEMENT_3D ( 'NONE', #5824, #14110, #1187 ) ;
#11956=CARTESIAN_POINT ( 'NONE',  ( 7.500000000000001776, -9.015933403756337545E-10, 22.35625000018031017 ) ) ;
#11961=AXIS2_PLACEMENT_3D ( 'NONE', #14746, #6576, #13055 ) ;
#11965=CARTESIAN_POINT ( 'NONE',  ( -7.500000000000007994, 9.015942588607339023E-10, 1.926200000180313454 ) ) ;
#11967=CARTESIAN_POINT ( 'NONE',  ( 11.17563879758427525, 2.222972768810836719, -19.19964100028681031 ) ) ;
#11974=CARTESIAN_POINT ( 'NONE',  ( -6.888301784570738384, -16.62983158437509346, -2.021137499819688266 ) ) ;
#11983=ORIENTED_EDGE ( 'NONE', *, *, #14052, .F. ) ;
#11986=CIRCLE ( 'NONE', #17059, 2.649999999999999467 ) ;
#11989=CARTESIAN_POINT ( 'NONE',  ( 17.50000000000000355, 2.143131898507868643E-15, 40.00000000000000000 ) ) ;
#11992=CARTESIAN_POINT ( 'NONE',  ( 4.248408729364575365, -6.358192988180014993, -7.578543749819688813 ) ) ;
#11998=CARTESIAN_POINT ( 'NONE',  ( -7.500000000000007105, 1.491842755816076505, 2.220731250087793818 ) ) ;
#12000=CARTESIAN_POINT ( 'NONE',  ( -10.19618095047498052, 15.25966317163203101, 8.739106250180315172 ) ) ;
#12007=DIRECTION ( 'NONE',  ( 1.000000000000000000, 0.000000000000000000, -0.000000000000000000 ) ) ;
#12013=CARTESIAN_POINT ( 'NONE',  ( 6.888301784570727726, 16.62983158437509701, -18.06323749981969584 ) ) ;
#12016=CARTESIAN_POINT ( 'NONE',  ( -13.67243654642775041, 5.663308650141531508, -12.85122941848092815 ) ) ;
#12017=CARTESIAN_POINT ( 'NONE',  ( 9.474249097082498849, -6.330490858644140850, 17.37620350064743135 ) ) ;
#12025=CARTESIAN_POINT ( 'NONE',  ( -6.888301780572501976, 16.62983158603122291, 1.513237500180310890 ) ) ;
#12042=CARTESIAN_POINT ( 'NONE',  ( 14.79893867793684059, 2.943691925285398359, 15.44576066884154564 ) ) ;
#12049=CARTESIAN_POINT ( 'NONE',  ( -12.72792205982779556, 12.72792206288790773, 17.86957500018031197 ) ) ;
#12061=CARTESIAN_POINT ( 'NONE',  ( 17.99999999956957808, -3.580422614997675446, 12.27348125018031233 ) ) ;
#12076=CARTESIAN_POINT ( 'NONE',  ( 5.303300858261588147, -5.303300859536636658, 7.816825000180313232 ) ) ;
#12077=CARTESIAN_POINT ( 'NONE',  ( 7.500000000000007105, -1.491842755816074284, 16.35823125008779044 ) ) ;
#12078=CARTESIAN_POINT ( 'NONE',  ( -6.330490856366290053, 9.474249098604506258, -12.71995350028680249 ) ) ;
#12079=AXIS2_PLACEMENT_3D ( 'NONE', #20762, #17183, #19187 ) ;
#12084=CARTESIAN_POINT ( 'NONE',  ( -2.163827323447878234E-09, -18.00000000000000000, -12.03519999981969235 ) ) ;
#12103=CARTESIAN_POINT ( 'NONE',  ( 7.499999999820660790, -1.491842756249031954, 0.6683312501803116978 ) ) ;
#12111=CARTESIAN_POINT ( 'NONE',  ( 15.25966317163202746, 10.19618095047498407, 1.670356250180311752 ) ) ;
#12114=DIRECTION ( 'NONE',  ( -0.000000000000000000, -0.000000000000000000, -1.000000000000000000 ) ) ;
#12122=CARTESIAN_POINT ( 'NONE',  ( -10.19618095414378445, -15.25966316918061239, -3.631206249819690424 ) ) ;
#12123=CARTESIAN_POINT ( 'NONE',  ( 17.50000000000000355, -2.143131898507868643E-15, -43.00000000000000000 ) ) ;
#12125=CARTESIAN_POINT ( 'NONE',  ( -2.222972771497745192, -11.17563879704982632, -18.55660899935256936 ) ) ;
#12126=EDGE_LOOP ( 'NONE', ( #1188, #17426 ) ) ;
#12128=EDGE_CURVE ( 'NONE', #7832, #19785, #9949, .T. ) ;
#12133=CARTESIAN_POINT ( 'NONE',  ( -16.62983158603122291, -6.888301780572501087, -0.8430124998196862895 ) ) ;
#12135=LINE ( 'NONE', #17006, #5628 ) ;
#12139=CARTESIAN_POINT ( 'NONE',  ( 4.248408730893249441, 6.358192987158596488, 14.59104375018031519 ) ) ;
#12141=DIRECTION ( 'NONE',  ( 0.000000000000000000, 0.000000000000000000, 1.000000000000000000 ) ) ;
#12144=PRODUCT_CONTEXT ( 'NONE', #13591, 'mechanical' ) ;
#12145=CARTESIAN_POINT ( 'NONE',  ( -10.46442989202484242, 10.46442989454075700, 2.780916918841545460 ) ) ;
#12151=CARTESIAN_POINT ( 'NONE',  ( 13.67243654778934925, 5.663308646854335215, -18.74185441848092637 ) ) ;
#12154=ORIENTED_EDGE ( 'NONE', *, *, #10485, .F. ) ;
#12161=CARTESIAN_POINT ( 'NONE',  ( 18.00000000043040771, 3.580422610670018546, 2.259418750180309576 ) ) ;
#12163=ORIENTED_EDGE ( 'NONE', *, *, #10693, .T. ) ;
#12169=CARTESIAN_POINT ( 'NONE',  ( 9.015937996181842420E-10, 7.500000000000007994, -14.56754999981968446 ) ) ;
#12171=UNCERTAINTY_MEASURE_WITH_UNIT (LENGTH_MEASURE( 1.000000000000000082E-05 ), #234, 'distance_accuracy_value', 'NONE');
#12172=CYLINDRICAL_SURFACE ( 'NONE', #3227, 7.500000000000000000 ) ;
#12173=CARTESIAN_POINT ( 'NONE',  ( 6.929096493489630859, -2.870125743571144472, 7.227762500180316074 ) ) ;
#12175=CARTESIAN_POINT ( 'NONE',  ( -7.902369978624323110, -7.902369976724391343, -24.79573475028681173 ) ) ;
#12181=CARTESIAN_POINT ( 'NONE',  ( -15.25966317163203279, -10.19618095047498052, -1.137543749819686978 ) ) ;
#12185=ORIENTED_EDGE ( 'NONE', *, *, #8639, .T. ) ;
#12196=CARTESIAN_POINT ( 'NONE',  ( -1.491842754445841246, 7.500000000179339210, -11.70198124981968846 ) ) ;
#12208=CARTESIAN_POINT ( 'NONE',  ( -15.25966316918061771, 10.19618095414378622, 8.150043750180314461 ) ) ;
#12222=CARTESIAN_POINT ( 'NONE',  ( 6.888301780572505528, -16.62983158603121581, -5.103862499819689980 ) ) ;
#12224=CARTESIAN_POINT ( 'NONE',  ( -7.500000000000000888, -3.289131931895657122E-15, 5.086300000002307087 ) ) ;
#12226=CARTESIAN_POINT ( 'NONE',  ( 7.902369976724399336, -7.902369978624331104, -10.60426524935257042 ) ) ;
#12233=CARTESIAN_POINT ( 'NONE',  ( 16.62983158437509346, -6.888301784570739272, -13.80238749981968915 ) ) ;
#12248=CARTESIAN_POINT ( 'NONE',  ( 14.79893867722910450, -2.943691928843438443, -2.815176831158457293 ) ) ;
#12256=CARTESIAN_POINT ( 'NONE',  ( 17.99999999999999645, -2.163824016901520184E-09, 2.553950000180309932 ) ) ;
#12257=CARTESIAN_POINT ( 'NONE',  ( -7.500000000000004441, 9.706494107352906755E-15, -23.18869999999769860 ) ) ;
#12268=CARTESIAN_POINT ( 'NONE',  ( -6.888301780572500199, 16.62983158603121936, -19.24136249981969016 ) ) ;
#12280=CARTESIAN_POINT ( 'NONE',  ( -12.72792206288791483, -12.72792205982780089, -1.432074999819690664 ) ) ;
#12286=CARTESIAN_POINT ( 'NONE',  ( -2.943691925285395694, 14.79893867793683349, 16.89642683151907576 ) ) ;
#12303=DIRECTION ( 'NONE',  ( -0.000000000000000000, -0.000000000000000000, 1.000000000000000000 ) ) ;
#12312=CARTESIAN_POINT ( 'NONE',  ( -2.870125741905209971, 6.929096494179676213, -11.99651249981969059 ) ) ;
#12323=CARTESIAN_POINT ( 'NONE',  ( 18.00000000000000000, -2.163824016901520184E-09, 2.553950000180313484 ) ) ;
#12336=CARTESIAN_POINT ( 'NONE',  ( -10.19618095047497874, 15.25966317163202746, -19.53589374981968874 ) ) ;
#12341=CARTESIAN_POINT ( 'NONE',  ( 1.491842754445842578, -7.500000000179340987, 11.86051875018030977 ) ) ;
#12349=CARTESIAN_POINT ( 'NONE',  ( -4.248408729364580694, 6.358192988180020322, -6.026143749819683038 ) ) ;
#12351=CARTESIAN_POINT ( 'NONE',  ( 2.163825119083639534E-09, 18.00000000000000000, -16.74769999981968738 ) ) ;
#12367=CARTESIAN_POINT ( 'NONE',  ( -14.79893867758297610, 1.779018419858781159E-09, 1.602791918841543595 ) ) ;
#12370=ORIENTED_EDGE ( 'NONE', *, *, #14999, .T. ) ;
#12372=CARTESIAN_POINT ( 'NONE',  ( 17.99999999956957808, -3.580422614997675446, 2.848481250180310287 ) ) ;
#12373=CARTESIAN_POINT ( 'NONE',  ( 0.000000000000000000, 0.000000000000000000, 40.00000000000000000 ) ) ;
#12380=VECTOR ( 'NONE', #19013, 1000.000000000000000 ) ;
#12382=CARTESIAN_POINT ( 'NONE',  ( 6.888301784570727726, 16.62983158437509701, -8.638237499819693355 ) ) ;
#12389=CARTESIAN_POINT ( 'NONE',  ( 15.25966316918061771, -10.19618095414378800, 14.76714375018030978 ) ) ;
#12392=CARTESIAN_POINT ( 'NONE',  ( -6.358192987158596488, 4.248408730893249441, -16.04020624981968979 ) ) ;
#12394=CARTESIAN_POINT ( 'NONE',  ( -7.500000000000007994, -4.022542210876018231E-17, 20.77620000000231570 ) ) ;
#12396=CARTESIAN_POINT ( 'NONE',  ( -14.79893867722910095, 2.943691928843434891, 5.704239331519073808 ) ) ;
#12400=ORIENTED_EDGE ( 'NONE', *, *, #14421, .F. ) ;
#12401=CARTESIAN_POINT ( 'NONE',  ( -7.500000000000009770, 9.706494115329868228E-15, -7.498799999997683763 ) ) ;
#12402=CARTESIAN_POINT ( 'NONE',  ( -15.25966317163203279, -10.19618095047498052, -19.98754374981969306 ) ) ;
#12415=DIRECTION ( 'NONE',  ( 0.5017436386064966225, -6.031582975246074897E-11, 0.8650163704334810078 ) ) ;
#12419=CARTESIAN_POINT ( 'NONE',  ( 4.248408729364575365, -6.358192988180014993, -26.42854374981969201 ) ) ;
#12429=CARTESIAN_POINT ( 'NONE',  ( -6.888301784570738384, -16.62983158437509346, -22.77573749981968732 ) ) ;
#12435=CARTESIAN_POINT ( 'NONE',  ( -7.500000000000004441, 9.706494107352906755E-15, -4.338699999997692736 ) ) ;
#12441=DIRECTION ( 'NONE',  ( 1.000000000000000000, 0.000000000000000000, 0.000000000000000000 ) ) ;
#12446=CARTESIAN_POINT ( 'NONE',  ( 7.500000000000000888, -2.290195989456150567E-15, 9.798800000002307442 ) ) ;
#12456=CARTESIAN_POINT ( 'NONE',  ( -2.163827323447878234E-09, -18.00000000000000000, -21.46019999981968951 ) ) ;
#12461=AXIS2_PLACEMENT_3D ( 'NONE', #19474, #3361, #185 ) ;
#12471=CARTESIAN_POINT ( 'NONE',  ( -10.46442989454075878, -10.46442989202484242, -9.000333081158460757 ) ) ;
#12477=CARTESIAN_POINT ( 'NONE',  ( 16.62983158437509346, -6.888301784570737496, 3.143012500180311086 ) ) ;
#12478=CARTESIAN_POINT ( 'NONE',  ( 9.015937996181835182E-10, 7.500000000000002665, -20.83244999981969059 ) ) ;
#12488=CARTESIAN_POINT ( 'NONE',  ( -6.358192988180015881, -4.248408729364577141, 4.202706250180307634 ) ) ;
#12490=CARTESIAN_POINT ( 'NONE',  ( -18.00000000043040771, -3.580422610670021211, -11.87808124981969193 ) ) ;
#12498=CARTESIAN_POINT ( 'NONE',  ( 15.25966317163203101, 10.19618095047498585, 3.574956250180307826 ) ) ;
#12499=CARTESIAN_POINT ( 'NONE',  ( 6.929096493489630859, -2.870125743571144472, -11.62223749981968624 ) ) ;
#12504=CARTESIAN_POINT ( 'NONE',  ( 2.943691928843430450, 14.79893867722910095, 17.48548933151908358 ) ) ;
#12507=DIRECTION ( 'NONE',  ( 1.000000000000000000, 0.000000000000000000, 0.000000000000000000 ) ) ;
#12508=CARTESIAN_POINT ( 'NONE',  ( 17.99999999956958163, -3.580422614997676334, -14.09691874981968773 ) ) ;
#12510=( BOUNDED_CURVE ( )  B_SPLINE_CURVE ( 2, ( #4862, #13028, #12830, #11334, #9831, #1788, #19273, #17698, #19483, #8050, #1596, #4968, #14522, #6439, #5058, #12925, #17906 ),
 .UNSPECIFIED., .F., .F. ) 
 B_SPLINE_CURVE_WITH_KNOTS ( ( 3, 2, 2, 2, 2, 2, 2, 2, 3 ),
 ( 0.000000000000000000, 0.01250000000048139860, 0.02500000000096279720, 0.03750000000144419060, 0.05000000000192559441, 0.06250000000240699127, 0.07500000000288838120, 0.08750000000336977113, 0.1000000000038511888 ),
 .UNSPECIFIED. ) 
 CURVE ( )  GEOMETRIC_REPRESENTATION_ITEM ( )  RATIONAL_B_SPLINE_CURVE ( ( 1.000000000000000000, 0.9807852804032304306, 1.000000000000000000, 0.9807852804032304306, 1.000000000000000000, 0.9807852804032304306, 1.000000000000000000, 0.9807852804032304306, 1.000000000000000000, 0.9807852804032304306, 1.000000000000000000, 0.9807852804032304306, 1.000000000000000000, 0.9807852804032304306, 1.000000000000000000, 0.9807852803973104994, 1.000000000005919931 ) ) 
 REPRESENTATION_ITEM ( '' )  );
#12524=CARTESIAN_POINT ( 'NONE',  ( -7.500000000000000888, 9.015942588607330751E-10, -23.18869999981969343 ) ) ;
#12531=CARTESIAN_POINT ( 'NONE',  ( 12.72792206288790950, 12.72792205982780089, -8.049174999819687315 ) ) ;
#12550=LINE ( 'NONE', #17110, #11514 ) ;
#12556=CARTESIAN_POINT ( 'NONE',  ( -18.00000000043041126, -3.580422610670022099, -9.973481249819688088 ) ) ;
#12569=CARTESIAN_POINT ( 'NONE',  ( 2.943691925285398803, -14.79893867793684059, -10.47298933115845188 ) ) ;
#12576=VECTOR ( 'NONE', #40, 1000.000000000000000 ) ;
#12577=CARTESIAN_POINT ( 'NONE',  ( -10.19618095414378445, -15.25966316918061239, 5.793793750180309843 ) ) ;
#12588=CARTESIAN_POINT ( 'NONE',  ( -2.163827323447877821E-09, -17.99999999999999645, -13.93979999981969442 ) ) ;
#12590=CARTESIAN_POINT ( 'NONE',  ( -6.929096494179684207, -2.870125741905212635, -8.087862499819687301 ) ) ;
#12599=CARTESIAN_POINT ( 'NONE',  ( 17.99999999956958519, -3.580422614997676778, 4.753081250180309247 ) ) ;
#12606=CARTESIAN_POINT ( 'NONE',  ( 14.79893867758296544, -1.779016607511491977E-09, 19.54720808151908074 ) ) ;
#12633=VECTOR ( 'NONE', #19137, 1000.000000000000000 ) ;
#12636=CARTESIAN_POINT ( 'NONE',  ( 4.276731815070943910, 10.32494394706616703, -13.54957774935257753 ) ) ;
#12638=CARTESIAN_POINT ( 'NONE',  ( 5.303300858261582817, -5.303300859536631329, -26.72307499981969059 ) ) ;
#12646=CARTESIAN_POINT ( 'NONE',  ( -16.62983158603122291, -6.888301780572501087, -21.59761249981969300 ) ) ;
#12653=CARTESIAN_POINT ( 'NONE',  ( -9.015947181032828388E-10, -7.500000000000002665, -6.694949999819694852 ) ) ;
#12654=CARTESIAN_POINT ( 'NONE',  ( 4.925000000000044231, 8.530350227276702668, -43.00000000000000000 ) ) ;
#12655=CARTESIAN_POINT ( 'NONE',  ( -7.500000000000000000, 0.000000000000000000, 40.00000000000000000 ) ) ;
#12666=CARTESIAN_POINT ( 'NONE',  ( -7.500000000000009770, 9.706494107251932559E-15, 1.926200000002316060 ) ) ;
#12667=ORIENTED_EDGE ( 'NONE', *, *, #14140, .T. ) ;
#12669=CARTESIAN_POINT ( 'NONE',  ( -5.303300858261589035, 5.303300859536635770, -6.320674999819683393 ) ) ;
#12673=CARTESIAN_POINT ( 'NONE',  ( -17.99999999956958519, 3.580422614997674113, -9.384418749819685601 ) ) ;
#12688=CARTESIAN_POINT ( 'NONE',  ( -9.474249097082500626, 6.330490858644140850, 22.08870350064742993 ) ) ;
#12690=CARTESIAN_POINT ( 'NONE',  ( -9.015947181032828388E-10, -7.500000000000002665, -16.11994999981969556 ) ) ;
#12696=CARTESIAN_POINT ( 'NONE',  ( 7.500000000000004441, 1.491842754878798027, -18.77073124991221320 ) ) ;
#12706=CARTESIAN_POINT ( 'NONE',  ( 10.19618095047497697, -15.25966317163202923, -14.82339374981969016 ) ) ;
#12714=CARTESIAN_POINT ( 'NONE',  ( -3.580422614997675890, -17.99999999956958519, -2.315668749819692618 ) ) ;
#12716=CARTESIAN_POINT ( 'NONE',  ( -6.929096494179684207, -2.870125741905212635, -17.51286249981968979 ) ) ;
#12720=CARTESIAN_POINT ( 'NONE',  ( 12.54593441764186679, 8.382925368423272516, 9.238614331519077183 ) ) ;
#12736=CARTESIAN_POINT ( 'NONE',  ( 18.00000000000000000, -2.163824016901520184E-09, 22.35625000018031372 ) ) ;
#12743=CARTESIAN_POINT ( 'NONE',  ( 9.474249097082498849, -6.330490858644140850, -10.89879649935257433 ) ) ;
#12744=CARTESIAN_POINT ( 'NONE',  ( 5.303300858261582817, -5.303300859536631329, -17.29807499981968988 ) ) ;
#12752=CYLINDRICAL_SURFACE ( 'NONE', #17001, 7.500000000000000000 ) ;
#12755=CARTESIAN_POINT ( 'NONE',  ( 12.72792205982779734, -12.72792206288791128, -15.11792499981968696 ) ) ;
#12764=CARTESIAN_POINT ( 'NONE',  ( -1.491842754445841690, 7.500000000179340987, -2.276981249819693520 ) ) ;
#12769=CARTESIAN_POINT ( 'NONE',  ( 12.72792205982779379, -12.72792206288790950, -24.54292499981969300 ) ) ;
#12797=DIRECTION ( 'NONE',  ( -1.000000000000000000, 0.000000000000000000, 0.000000000000000000 ) ) ;
#12798=CARTESIAN_POINT ( 'NONE',  ( 2.222972768810839383, -11.17563879758428769, 18.55432850064742922 ) ) ;
#12805=VECTOR ( 'NONE', #19214, 1000.000000000000000 ) ;
#12808=VERTEX_POINT ( 'NONE', #9433 ) ;
#12822=CARTESIAN_POINT ( 'NONE',  ( 10.19618095414378978, 15.25966316918061771, -6.439106249819692707 ) ) ;
#12826=CARTESIAN_POINT ( 'NONE',  ( -14.79893867758296544, 1.779018419858780125E-09, -4.015291918480927258 ) ) ;
#12830=CARTESIAN_POINT ( 'NONE',  ( 6.929096494179683319, 2.870125741905213079, 24.89963750018031519 ) ) ;
#12836=CARTESIAN_POINT ( 'NONE',  ( 15.25966317163202568, 10.19618095047498230, 20.52035625018030984 ) ) ;
#12843=CARTESIAN_POINT ( 'NONE',  ( 4.276731815070943910, 10.32494394706616703, -4.124577749352575040 ) ) ;
#12845=CARTESIAN_POINT ( 'NONE',  ( 6.330490858644138186, 9.474249097082495297, 17.32223399971320532 ) ) ;
#12853=CARTESIAN_POINT ( 'NONE',  ( -16.62983158437510056, 6.888301784570729502, 9.760112500180312622 ) ) ;
#12868=EDGE_CURVE ( 'NONE', #15181, #2818, #2857, .T. ) ;
#12889=DIRECTION ( 'NONE',  ( -0.4999999999999918954, 0.8660254037844433705, 0.000000000000000000 ) ) ;
#12891=CARTESIAN_POINT ( 'NONE',  ( 10.46442989202484064, -10.46442989454075878, -11.35658308115845472 ) ) ;
#12893=CARTESIAN_POINT ( 'NONE',  ( -7.500000000000000000, 0.000000000000000000, -40.00000000000000000 ) ) ;
#12897=CARTESIAN_POINT ( 'NONE',  ( -1.491842756249031954, -7.499999999820663454, -25.25041874981969414 ) ) ;
#12913=CARTESIAN_POINT ( 'NONE',  ( -15.25966316918061949, 10.19618095414378800, -18.22035624981969093 ) ) ;
#12918=CARTESIAN_POINT ( 'NONE',  ( -14.79893867793683349, -2.943691925285398359, -13.73482316848092744 ) ) ;
#12925=CARTESIAN_POINT ( 'NONE',  ( -7.500000000000007994, 1.491842755816071842, 21.07073125008779613 ) ) ;
#12933=CARTESIAN_POINT ( 'NONE',  ( -6.888301780572500199, 16.62983158603121936, 18.45863750018030913 ) ) ;
#12942=CARTESIAN_POINT ( 'NONE',  ( 6.358192988180019434, 4.248408729364581582, 24.60510625018031661 ) ) ;
#12944=CARTESIAN_POINT ( 'NONE',  ( 9.474249098604504482, 6.330490856366291830, -0.9387035002868041600 ) ) ;
#12948=DIRECTION ( 'NONE',  ( 1.000000000000000000, 0.000000000000000000, 0.000000000000000000 ) ) ;
#12951=ORIENTED_EDGE ( 'NONE', *, *, #7519, .F. ) ;
#12952=CARTESIAN_POINT ( 'NONE',  ( 12.72792205982779734, -12.72792206288791128, 15.06167500018031369 ) ) ;
#12957=DIRECTION ( 'NONE',  ( 1.000000000000000000, 0.000000000000000000, 0.000000000000000000 ) ) ;
#12965=AXIS2_PLACEMENT_3D ( 'NONE', #16584, #5450, #1871 ) ;
#12970=CARTESIAN_POINT ( 'NONE',  ( -6.929096493489625530, 2.870125743571138255, 5.675362500180312075 ) ) ;
#12978=CARTESIAN_POINT ( 'NONE',  ( -17.99999999956958519, 3.580422614997674113, 16.98598125018031268 ) ) ;
#12992=CARTESIAN_POINT ( 'NONE',  ( -11.17563879758428769, -2.222972768810840272, 20.91057850064743207 ) ) ;
#12998=CIRCLE ( 'NONE', #5185, 2.649999999999999467 ) ;
#13000=CARTESIAN_POINT ( 'NONE',  ( -6.888301784570738384, -16.62983158437509346, 16.82886250018031404 ) ) ;
#13006=ADVANCED_FACE ( 'NONE', ( #3172 ), #16205, .F. ) ;
#13013=CARTESIAN_POINT ( 'NONE',  ( 10.19618095047497697, -15.25966317163202923, -24.24839374981969087 ) ) ;
#13019=CARTESIAN_POINT ( 'NONE',  ( -3.580422610670018990, 18.00000000043041481, -7.617231249819690575 ) ) ;
#13024=CARTESIAN_POINT ( 'NONE',  ( 10.46442989454075168, 10.46442989202483886, -9.905916918480928146 ) ) ;
#13028=CARTESIAN_POINT ( 'NONE',  ( 7.500000000179346316, 1.491842754445843244, 25.19416875018031732 ) ) ;
#13035=CARTESIAN_POINT ( 'NONE',  ( 6.888301784570727726, 16.62983158437509701, 19.63676250018031411 ) ) ;
#13039=DIRECTION ( 'NONE',  ( 0.000000000000000000, 0.000000000000000000, 1.000000000000000000 ) ) ;
#13045=CARTESIAN_POINT ( 'NONE',  ( 6.330490856366294494, -9.474249098604513364, -19.73473399935257788 ) ) ;
#13047=CARTESIAN_POINT ( 'NONE',  ( -9.474249097082497073, 6.330490858644137298, -3.884016000286802495 ) ) ;
#13052=CARTESIAN_POINT ( 'NONE',  ( -15.25966316918061771, 10.19618095414378622, 19.47964375018031546 ) ) ;
#13055=DIRECTION ( 'NONE',  ( 1.000000000000000000, 0.000000000000000000, 0.000000000000000000 ) ) ;
#13070=CARTESIAN_POINT ( 'NONE',  ( -4.248408730893245000, -6.358192987158590270, 13.03864375018031296 ) ) ;
#13073=DIRECTION ( 'NONE',  ( -1.000000000000000000, 0.000000000000000000, 0.000000000000000000 ) ) ;
#13081=CARTESIAN_POINT ( 'NONE',  ( -12.72792206288791128, -12.72792205982779912, 15.51332500018031624 ) ) ;
#13094=CARTESIAN_POINT ( 'NONE',  ( -7.902369978624331104, -7.902369976724401113, 20.02698475064743278 ) ) ;
#13102=AXIS2_PLACEMENT_3D ( 'NONE', #10033, #4950, #4847 ) ;
#13110=EDGE_CURVE ( 'NONE', #3529, #13866, #19666, .T. ) ;
#13113=CYLINDRICAL_SURFACE ( 'NONE', #12965, 2.650000000000000355 ) ;
#13115=CARTESIAN_POINT ( 'NONE',  ( -6.888301784570736608, -16.62983158437509346, -22.77573749981969087 ) ) ;
#13117=ORIENTED_EDGE ( 'NONE', *, *, #17932, .F. ) ;
#13122=CARTESIAN_POINT ( 'NONE',  ( 16.62983158437509701, -6.888301784570740161, -4.377387499819692884 ) ) ;
#13130=CARTESIAN_POINT ( 'NONE',  ( 5.663308646854338768, -13.67243654778934747, 2.464395581519073897 ) ) ;
#13152=CARTESIAN_POINT ( 'NONE',  ( -5.303300858261589035, 5.303300859536635770, 12.52932500018031448 ) ) ;
#13153=CARTESIAN_POINT ( 'NONE',  ( 11.17563879731704723, -1.343450868547281106E-09, -0.05510975028680254600 ) ) ;
#13156=EDGE_LOOP ( 'NONE', ( #94, #8977, #1674, #20043 ) ) ;
#13158=CARTESIAN_POINT ( 'NONE',  ( 18.00000000000000000, -2.163824016901520184E-09, -25.72104999981969087 ) ) ;
#13166=EDGE_CURVE ( 'NONE', #10361, #7721, #9092, .T. ) ;
#13168=ORIENTED_EDGE ( 'NONE', *, *, #355, .F. ) ;
#13170=SURFACE_STYLE_FILL_AREA ( #14859 ) ;
#13174=CARTESIAN_POINT ( 'NONE',  ( -7.500000000000000888, 9.015942588607330751E-10, 14.51130000018031119 ) ) ;
#13180=ORIENTED_EDGE ( 'NONE', *, *, #5970, .F. ) ;
#13183=CARTESIAN_POINT ( 'NONE',  ( -6.888301780572501976, 16.62983158603122291, 18.45863750018031268 ) ) ;
#13189=FACE_BOUND ( 'NONE', #1767, .T. ) ;
#13191=( BOUNDED_CURVE ( )  B_SPLINE_CURVE ( 2, ( #3894, #16937, #8772, #3999, #6866, #7074, #13554, #20000, #12169, #16733, #5484, #13461, #5283, #19907, #18544, #2212, #18320 ),
 .UNSPECIFIED., .F., .F. ) 
 B_SPLINE_CURVE_WITH_KNOTS ( ( 3, 2, 2, 2, 2, 2, 2, 2, 3 ),
 ( 0.8000000000038511860, 0.8125000000038511416, 0.8250000000038510972, 0.8375000000038511638, 0.8500000000038511194, 0.8625000000038511860, 0.8750000000038511416, 0.8875000000038510972, 0.9000000000038511638 ),
 .UNSPECIFIED. ) 
 CURVE ( )  GEOMETRIC_REPRESENTATION_ITEM ( )  RATIONAL_B_SPLINE_CURVE ( ( 0.9999999999940800688, 0.9807852804091503618, 1.000000000000000000, 0.9807852804032304306, 1.000000000000000000, 0.9807852804032304306, 1.000000000000000000, 0.9807852804032304306, 1.000000000000000000, 0.9807852804032304306, 1.000000000000000000, 0.9807852804032304306, 1.000000000000000000, 0.9807852804032304306, 1.000000000000000000, 0.9807852803973104994, 1.000000000005919931 ) ) 
 REPRESENTATION_ITEM ( '' )  );
#13196=CARTESIAN_POINT ( 'NONE',  ( -9.474249097082500626, 6.330490858644140850, 3.238703500647428957 ) ) ;
#13203=CARTESIAN_POINT ( 'NONE',  ( 18.00000000043041126, 3.580422610670019434, 23.01401875018031262 ) ) ;
#13210=CARTESIAN_POINT ( 'NONE',  ( -5.303300859536636658, -5.303300858261589035, -18.10192499981969050 ) ) ;
#13219=CARTESIAN_POINT ( 'NONE',  ( -12.72792205982780089, 12.72792206288791128, -17.92582499981969235 ) ) ;
#13221=CARTESIAN_POINT ( 'NONE',  ( 7.500000000000000888, -2.290195989456150567E-15, 9.798800000002307442 ) ) ;
#13224=CARTESIAN_POINT ( 'NONE',  ( 12.54593441764186679, 8.382925368423272516, -0.1863856684809275799 ) ) ;
#13228=FACE_OUTER_BOUND ( 'NONE', #13156, .T. ) ;
#13229=CARTESIAN_POINT ( 'NONE',  ( -6.929096493489627306, 2.870125743571138699, 15.10036250018031012 ) ) ;
#13232=CARTESIAN_POINT ( 'NONE',  ( -5.303300859536636658, -5.303300858261589035, 10.17307500018031519 ) ) ;
#13233=EDGE_LOOP ( 'NONE', ( #16554, #3797, #19407, #6592, #13823, #20019 ) ) ;
#13248=CARTESIAN_POINT ( 'NONE',  ( -9.015947181032835626E-10, -7.500000000000007994, 8.994950000180315541 ) ) ;
#13249=CARTESIAN_POINT ( 'NONE',  ( -1.343452921478823292E-09, -11.17563879731704723, 11.72614024971320212 ) ) ;
#13256=CARTESIAN_POINT ( 'NONE',  ( -18.00000000000000000, 2.163826221265758884E-09, 9.171050000180313688 ) ) ;
#13275=CARTESIAN_POINT ( 'NONE',  ( 2.870125743571137811, 6.929096493489625530, 8.031612500180312253 ) ) ;
#13283=CARTESIAN_POINT ( 'NONE',  ( -16.62983158603122291, -6.888301780572501087, 16.10238750018031695 ) ) ;
#13291=PLANE ( 'NONE',  #14155 ) ;
#13295=CARTESIAN_POINT ( 'NONE',  ( -7.500000000000004441, 9.706494115430842424E-15, -13.76369999999769256 ) ) ;
#13298=CARTESIAN_POINT ( 'NONE',  ( -9.474249098604513364, -6.330490856366295382, 1.471516000647429268 ) ) ;
#13310=CARTESIAN_POINT ( 'NONE',  ( 6.888301784570728614, 16.62983158437510056, 12.11636250018031369 ) ) ;
#13315=EDGE_LOOP ( 'NONE', ( #3777, #1637 ) ) ;
#13322=DIRECTION ( 'NONE',  ( -0.000000000000000000, -0.000000000000000000, -1.000000000000000000 ) ) ;
#13325=CARTESIAN_POINT ( 'NONE',  ( 1.779017513685136568E-09, 14.79893867758297610, 22.80904191884154741 ) ) ;
#13334=CARTESIAN_POINT ( 'NONE',  ( -6.888301780572500199, 16.62983158603121936, 18.45863750018030913 ) ) ;
#13347=CARTESIAN_POINT ( 'NONE',  ( -12.72792206288790950, -12.72792205982779556, -3.336674999819690068 ) ) ;
#13357=CARTESIAN_POINT ( 'NONE',  ( -1.491842756249033064, -7.499999999820668783, 18.71448125018031661 ) ) ;
#13359=CARTESIAN_POINT ( 'NONE',  ( 4.276731815070940357, 10.32494394706615815, -11.24729725028680782 ) ) ;
#13364=VERTEX_POINT ( 'NONE', #3144 ) ;
#13367=CARTESIAN_POINT ( 'NONE',  ( 2.163825119083639534E-09, 18.00000000000000000, 2.102300000180311823 ) ) ;
#13386=CARTESIAN_POINT ( 'NONE',  ( -2.870125743571140919, -6.929096493489624642, 3.319112500180312786 ) ) ;
#13405=CARTESIAN_POINT ( 'NONE',  ( 4.248408730893246776, 6.358192987158592047, -10.52385624981969414 ) ) ;
#13406=CARTESIAN_POINT ( 'NONE',  ( -12.72792206288790950, -12.72792205982779556, -12.76167499981969300 ) ) ;
#13410=CARTESIAN_POINT ( 'NONE',  ( -11.17563879704982988, 2.222972771497744748, 2.649641000647427802 ) ) ;
#13419=CARTESIAN_POINT ( 'NONE',  ( -17.99999999956958519, 3.580422614997674113, 0.04058125018031183417 ) ) ;
#13430=EDGE_LOOP ( 'NONE', ( #3349, #16267, #7155, #2660 ) ) ;
#13434=CARTESIAN_POINT ( 'NONE',  ( 10.46442989454075700, 10.46442989202484419, 14.56216691884154812 ) ) ;
#13441=CARTESIAN_POINT ( 'NONE',  ( 12.72792206288790773, 12.72792205982779912, 20.22582500018031482 ) ) ;
#13452=CARTESIAN_POINT ( 'NONE',  ( -10.19618095047497874, 15.25966317163202746, -0.6858937498196888694 ) ) ;
#13453=ADVANCED_FACE ( 'NONE', ( #20940, #13189, #14877, #6805 ), #13291, .T. ) ;
#13454=ORIENTED_EDGE ( 'NONE', *, *, #7266, .F. ) ;
#13461=CARTESIAN_POINT ( 'NONE',  ( -4.248408729364580694, 6.358192988180020322, -15.45114374981968552 ) ) ;
#13464=CARTESIAN_POINT ( 'NONE',  ( -6.358192988180021210, -4.248408729364580694, 1.042606250180315497 ) ) ;
#13466=CARTESIAN_POINT ( 'NONE',  ( -2.222972768810836275, 11.17563879758427525, -12.13089100028680534 ) ) ;
#13473=CARTESIAN_POINT ( 'NONE',  ( 3.580422614997668340, 17.99999999956958519, -7.028168749819689864 ) ) ;
#13487=CARTESIAN_POINT ( 'NONE',  ( 6.358192988180013216, 4.248408729364577141, -9.934793749819688102 ) ) ;
#13496=CARTESIAN_POINT ( 'NONE',  ( 17.99999999956958163, -3.580422614997676334, 2.848481250180313840 ) ) ;
#13501=DIRECTION ( 'NONE',  ( -0.4999999999999918954, 0.8660254037844433705, 0.000000000000000000 ) ) ;
#13502=DIRECTION ( 'NONE',  ( 0.000000000000000000, 0.000000000000000000, 1.000000000000000000 ) ) ;
#13506=CARTESIAN_POINT ( 'NONE',  ( -6.888301784570736608, -16.62983158437509346, -13.35073749981969371 ) ) ;
#13512=CARTESIAN_POINT ( 'NONE',  ( 1.343451552857795926E-09, 11.17563879731705789, 4.711359750647427624 ) ) ;
#13518=CARTESIAN_POINT ( 'NONE',  ( 3.580422610670020322, -18.00000000043041126, -2.904731249819686667 ) ) ;
#13521=ORIENTED_EDGE ( 'NONE', *, *, #7940, .F. ) ;
#13532=CARTESIAN_POINT ( 'NONE',  ( 15.25966316918061771, -10.19618095414378800, -22.93285624981969306 ) ) ;
#13537=CARTESIAN_POINT ( 'NONE',  ( 8.382925368423265411, -12.54593441764187034, -26.10513566848092992 ) ) ;
#13547=CARTESIAN_POINT ( 'NONE',  ( 16.62983158603121936, 6.888301780572501976, 1.964887500180308777 ) ) ;
#13554=CARTESIAN_POINT ( 'NONE',  ( 2.870125743571140475, 6.929096493489632635, -13.97848749981969085 ) ) ;
#13556=CARTESIAN_POINT ( 'NONE',  ( -1.491842756249033064, -7.499999999820668783, -0.1355187498196866458 ) ) ;
#13559=CARTESIAN_POINT ( 'NONE',  ( -6.330490856366290053, 9.474249098604506258, -22.14495350028680676 ) ) ;
#13566=CARTESIAN_POINT ( 'NONE',  ( 15.25966316918061416, -10.19618095414378622, -4.082856249819688088 ) ) ;
#13573=ORIENTED_EDGE ( 'NONE', *, *, #10403, .F. ) ;
#13578=FACE_OUTER_BOUND ( 'NONE', #218, .T. ) ;
#13580=CARTESIAN_POINT ( 'NONE',  ( 7.500000000179339210, 1.491842754445841690, 0.07926875018031064035 ) ) ;
#13587=CARTESIAN_POINT ( 'NONE',  ( 5.303300859536635770, 5.303300858261589923, 5.460575000180316607 ) ) ;
#13589=CARTESIAN_POINT ( 'NONE',  ( -12.72792206288791128, -12.72792205982779912, -3.336674999819686516 ) ) ;
#13591=APPLICATION_CONTEXT ( 'automotive_design' ) ;
#13598=VERTEX_POINT ( 'NONE', #7023 ) ;
#13603=CARTESIAN_POINT ( 'NONE',  ( 15.25966317163202568, 10.19618095047498230, -17.17964374981969655 ) ) ;
#13608=CARTESIAN_POINT ( 'NONE',  ( -1.343452921478824119E-09, -11.17563879731705789, -0.001140249352573480474 ) ) ;
#13611=FACE_OUTER_BOUND ( 'NONE', #3883, .T. ) ;
#13617=CARTESIAN_POINT ( 'NONE',  ( 6.888301780572507305, -16.62983158603121936, 6.225737500180312800 ) ) ;
#13625=EDGE_CURVE ( 'NONE', #10361, #9436, #6672, .T. ) ;
#13631=AXIS2_PLACEMENT_3D ( 'NONE', #9421, #7929, #15876 ) ;
#13635=CARTESIAN_POINT ( 'NONE',  ( -10.46442989202484242, 10.46442989454075700, 21.63091691884155310 ) ) ;
#13642=CARTESIAN_POINT ( 'NONE',  ( -14.79893867793683349, -2.943691925285398359, -23.15982316848093348 ) ) ;
#13645=CIRCLE ( 'NONE', #17729, 7.500000000000000000 ) ;
#13648=CARTESIAN_POINT ( 'NONE',  ( 7.500000000000000888, -2.290195989456150567E-15, 9.798800000002307442 ) ) ;
#13652=VERTEX_POINT ( 'NONE', #12655 ) ;
#13654=CARTESIAN_POINT ( 'NONE',  ( 15.25966316918061239, -10.19618095414378445, 12.86254375018031126 ) ) ;
#13667=CARTESIAN_POINT ( 'NONE',  ( 1.491842756249030622, 7.499999999820669672, 4.576981250180313765 ) ) ;
#13669=CARTESIAN_POINT ( 'NONE',  ( -11.17563879704981922, 2.222972771497742972, -23.32307850028680463 ) ) ;
#13675=CARTESIAN_POINT ( 'NONE',  ( 10.19618095414378800, 15.25966316918061416, -6.439106249819689154 ) ) ;
#13693=CARTESIAN_POINT ( 'NONE',  ( -7.500000000179339210, -1.491842754445842800, -4.633231249819690589 ) ) ;
#13700=CARTESIAN_POINT ( 'NONE',  ( 2.163825119083639534E-09, 18.00000000000000000, 9.622700000180314461 ) ) ;
#13703=DIRECTION ( 'NONE',  ( 0.000000000000000000, 0.000000000000000000, 1.000000000000000000 ) ) ;
#13713=CARTESIAN_POINT ( 'NONE',  ( 16.62983158603121936, 6.888301780572501976, -7.460112499819690157 ) ) ;
#13717=CARTESIAN_POINT ( 'NONE',  ( -6.330490858644140850, -9.474249097082498849, -17.96754649935258286 ) ) ;
#13719=EDGE_LOOP ( 'NONE', ( #8865, #13573, #19239, #3214 ) ) ;
#13726=CARTESIAN_POINT ( 'NONE',  ( -16.62983158437510056, 6.888301784570729502, 9.760112500180312622 ) ) ;
#13732=CARTESIAN_POINT ( 'NONE',  ( 1.491842756249030399, 7.499999999820669672, 14.00198125018031625 ) ) ;
#13740=CARTESIAN_POINT ( 'NONE',  ( 2.943691928843431782, 14.79893867722910628, -5.171426831158459692 ) ) ;
#13747=CARTESIAN_POINT ( 'NONE',  ( -8.382925371439625906, -12.54593441562639988, -24.33794816848093134 ) ) ;
#13754=CARTESIAN_POINT ( 'NONE',  ( 7.500000000000000000, -9.015933403756339613E-10, -21.63629999981969121 ) ) ;
#13760=CARTESIAN_POINT ( 'NONE',  ( 3.580422614997667896, 17.99999999956958163, 9.917231250180311264 ) ) ;
#13772=EDGE_CURVE ( 'NONE', #12808, #13364, #1416, .T. ) ;
#13777=CARTESIAN_POINT ( 'NONE',  ( -2.870125741905213079, 6.929096494179683319, 3.693387500180313143 ) ) ;
#13778=CARTESIAN_POINT ( 'NONE',  ( 7.500000000000007105, -2.290195989506637665E-15, 16.06370000000231357 ) ) ;
#13779=CARTESIAN_POINT ( 'NONE',  ( -10.32494394809439164, -4.276731812588563386, -24.20667225028680747 ) ) ;
#13786=CARTESIAN_POINT ( 'NONE',  ( -10.19618095414378622, -15.25966316918061416, -11.15160624981968951 ) ) ;
#13797=CARTESIAN_POINT ( 'NONE',  ( 6.249999999999902300, -10.82531754730554496, -43.00000000000000000 ) ) ;
#13805=CARTESIAN_POINT ( 'NONE',  ( -9.015947181032828388E-10, -7.500000000000000888, 2.730050000180312075 ) ) ;
#13806=CARTESIAN_POINT ( 'NONE',  ( 17.50000000000000355, -2.143131898507868643E-15, -43.00000000000000000 ) ) ;
#13809=CARTESIAN_POINT ( 'NONE',  ( 6.250000000000054179, 10.82531754730546147, -40.00000000000000000 ) ) ;
#13814=CARTESIAN_POINT ( 'NONE',  ( -18.00000000043041126, -3.580422610670022543, 6.971918750180314817 ) ) ;
#13823=ORIENTED_EDGE ( 'NONE', *, *, #17892, .F. ) ;
#13824=CARTESIAN_POINT ( 'NONE',  ( -6.358192988180021210, -4.248408729364580694, -17.80739374981969192 ) ) ;
#13826=CARTESIAN_POINT ( 'NONE',  ( 18.00000000043040771, 3.580422610670018546, -16.59058124981969229 ) ) ;
#13829=CARTESIAN_POINT ( 'NONE',  ( -11.17563879758428769, -2.222972768810840272, -7.364421499352572731 ) ) ;
#13836=CARTESIAN_POINT ( 'NONE',  ( 6.888301780572507305, -16.62983158603121936, -12.62426249981968596 ) ) ;
#13842=CARTESIAN_POINT ( 'NONE',  ( 7.500000000000007105, -2.290195989506637665E-15, 16.06370000000231357 ) ) ;
#13847=CARTESIAN_POINT ( 'NONE',  ( -10.46442989454075878, -10.46442989202484242, 0.4246669188415451712 ) ) ;
#13852=CARTESIAN_POINT ( 'NONE',  ( -17.99999999956958163, 3.580422614997673669, 7.560981250180310198 ) ) ;
#13858=ORIENTED_EDGE ( 'NONE', *, *, #18557, .F. ) ;
#13863=CARTESIAN_POINT ( 'NONE',  ( 10.19618095414378622, 15.25966316918061239, -8.343706249819691223 ) ) ;
#13866=VERTEX_POINT ( 'NONE', #6472 ) ;
#13872=CARTESIAN_POINT ( 'NONE',  ( -10.19618095414378800, -15.25966316918061771, 7.698393750180310136 ) ) ;
#13876=CARTESIAN_POINT ( 'NONE',  ( 2.870125741905214412, -6.929096494179682431, -1.019112499819684770 ) ) ;
#13879=CARTESIAN_POINT ( 'NONE',  ( 2.870125741905214412, -6.929096494179682431, 17.83088750018031732 ) ) ;
#13880=CARTESIAN_POINT ( 'NONE',  ( 1.779017513685135741E-09, 14.79893867758296544, 7.765958081519076295 ) ) ;
#13884=CARTESIAN_POINT ( 'NONE',  ( 7.575000000000064126, 13.12028486733421850, -43.00000000000000000 ) ) ;
#13885=CARTESIAN_POINT ( 'NONE',  ( 16.62983158437509346, -6.888301784570739272, -13.80238749981968915 ) ) ;
#13886=CARTESIAN_POINT ( 'NONE',  ( -15.15000000000000568, -3.245314017740485469E-16, -43.00000000000000000 ) ) ;
#13893=AXIS2_PLACEMENT_3D ( 'NONE', #8797, #18783, #17295 ) ;
#13900=CARTESIAN_POINT ( 'NONE',  ( 0.000000000000000000, 0.000000000000000000, 43.00000000000000000 ) ) ;
#13901=CARTESIAN_POINT ( 'NONE',  ( -6.358192987158591158, 4.248408730893245000, -3.455106249819688724 ) ) ;
#13909=ORIENTED_EDGE ( 'NONE', *, *, #18566, .F. ) ;
#13912=CARTESIAN_POINT ( 'NONE',  ( 10.19618095047497874, -15.25966317163203279, 4.026606250180313040 ) ) ;
#13937=CARTESIAN_POINT ( 'NONE',  ( -18.00000000000000000, 2.163826221265758884E-09, -19.10394999981969022 ) ) ;
#13953=CARTESIAN_POINT ( 'NONE',  ( 14.79893867758297610, -1.779016607511492805E-09, -3.109708081158454096 ) ) ;
#13961=CARTESIAN_POINT ( 'NONE',  ( -6.888301780572500199, 16.62983158603121936, 9.033637500180310198 ) ) ;
#13972=CARTESIAN_POINT ( 'NONE',  ( 3.580422610670019878, -18.00000000043040771, -4.809331249819689624 ) ) ;
#13983=CARTESIAN_POINT ( 'NONE',  ( 18.00000000043041481, 3.580422610670020322, 13.58901875018030836 ) ) ;
#13984=CARTESIAN_POINT ( 'NONE',  ( 5.303300858261588147, -5.303300859536636658, -11.03317499981968552 ) ) ;
#13990=CARTESIAN_POINT ( 'NONE',  ( 14.79893867793683349, 2.943691925285396582, 9.827676831519074341 ) ) ;
#14004=ORIENTED_EDGE ( 'NONE', *, *, #17793, .F. ) ;
#14015=CARTESIAN_POINT ( 'NONE',  ( 5.303300859536630441, 5.303300858261584594, -19.65432499981969272 ) ) ;
#14026=CARTESIAN_POINT ( 'NONE',  ( -15.25966316918061771, 10.19618095414378622, -10.69995624981968518 ) ) ;
#14033=CYLINDRICAL_SURFACE ( 'NONE', #9729, 7.500000000000000000 ) ;
#14034=CARTESIAN_POINT ( 'NONE',  ( 4.248408730893246776, 6.358192987158592047, -1.098856249819691433 ) ) ;
#14051=CARTESIAN_POINT ( 'NONE',  ( 7.574999999999881162, -13.12028486733431976, -43.00000000000000000 ) ) ;
#14052=EDGE_CURVE ( 'NONE', #12808, #9351, #17507, .T. ) ;
#14054=CARTESIAN_POINT ( 'NONE',  ( -3.580422614997675002, -17.99999999956958163, -21.16566874981968738 ) ) ;
#14062=CARTESIAN_POINT ( 'NONE',  ( -5.303300858261584594, 5.303300859536631329, 6.264425000180307457 ) ) ;
#14066=CARTESIAN_POINT ( 'NONE',  ( -14.79893867758297610, 1.779018419858781159E-09, -7.822208081158454895 ) ) ;
#14072=CARTESIAN_POINT ( 'NONE',  ( -10.19618095414378445, -15.25966316918061239, 15.21879375018031055 ) ) ;
#14073=CARTESIAN_POINT ( 'NONE',  ( 4.248408730893246776, 6.358192987158592047, -19.94885624981969841 ) ) ;
#14082=AXIS2_PLACEMENT_3D ( 'NONE', #3193, #8, #12948 ) ;
#14084=CARTESIAN_POINT ( 'NONE',  ( 16.62983158437509346, -6.888301784570737496, -6.281987499819692289 ) ) ;
#14091=CARTESIAN_POINT ( 'NONE',  ( 2.163825119083639947E-09, 18.00000000000000355, 11.52730000018030942 ) ) ;
#14093=CARTESIAN_POINT ( 'NONE',  ( 2.870125741905214412, -6.929096494179682431, -19.86911249981968552 ) ) ;
#14098=CARTESIAN_POINT ( 'NONE',  ( -13.67243654642775041, 5.663308650141531508, 5.998770581519074163 ) ) ;
#14104=CARTESIAN_POINT ( 'NONE',  ( 18.00000000000000000, -2.163824016901520184E-09, -14.39144999981968986 ) ) ;
#14110=DIRECTION ( 'NONE',  ( -0.000000000000000000, -0.000000000000000000, 1.000000000000000000 ) ) ;
#14120=FILL_AREA_STYLE ('',( #7640 ) ) ;
#14121=CARTESIAN_POINT ( 'NONE',  ( -10.32494394809439164, -4.276731812588563386, 13.49332774971320248 ) ) ;
#14123=( BOUNDED_CURVE ( )  B_SPLINE_CURVE ( 2, ( #8215, #13203, #14588, #1565, #11301, #16486, #19559, #3441, #4935, #4729, #20935, #14692, #3240, #17666, #6318, #1669, #5035, #11606, #8116, #61, #17972, #6516, #13000, #19453, #19652, #9909, #1864, #275, #6723, #11912, #684, #8738, #3961, #369, #7244, #488, #15205, #3650, #13310, #6934, #3744, #794, #10441, #2176, #11715, #5246, #13726, #16903, #16686, #17003, #18600, #6823, #18494, #2379, #2490, #7133, #8832, #5347, #13617, #20174, #5548, #19763, #5440, #20066, #8630, #18185, #8519, #11814, #15307, #2063, #5660, #10543, #14893, #18385, #12025, #18277, #15000, #10124, #15104, #13419, #4061, #16794, #12133, #16577, #19872, #10225, #592, #2280, #7040, #13518, #19961, #3854, #10332, #19021, #15417, #1336, #15519, #9272, #18707, #7356, #1012, #7681, #15843, #4498, #17227, #5758, #20279, #7780, #10964, #10766, #11076, #12673, #904, #12556, #17440, #17553, #15734, #2911, #20392, #1233, #14255, #2698, #13836, #20502, #14160, #9164, #12233, #2601, #5878, #9381, #17116, #20700, #4605, #8950, #5981, #20603, #12351, #9067, #4178, #15621, #7456, #10659, #10857, #6187, #13937, #18816, #4287, #1123, #17328, #19133, #7569, #14054, #12456, #18924, #4389, #2804, #6080, #14666, #5107, #11172, #16158 ),
 .UNSPECIFIED., .F., .T. ) 
 B_SPLINE_CURVE_WITH_KNOTS ( ( 3, 2, 2, 2, 2, 2, 2, 2, 2, 2, 2, 2, 2, 2, 2, 2, 2, 2, 2, 2, 2, 2, 2, 2, 2, 2, 2, 2, 2, 2, 2, 2, 2, 2, 2, 2, 2, 2, 2, 2, 2, 2, 2, 2, 2, 2, 2, 2, 2, 2, 2, 2, 2, 2, 2, 2, 2, 2, 2, 2, 2, 2, 2, 2, 2, 2, 2, 2, 2, 2, 2, 2, 2, 2, 2, 2, 2, 2, 2, 2, 3 ),
 ( 0.000000000000000000, 0.01250000000000000069, 0.02500000000000000139, 0.03749999999999999861, 0.05000000000000000278, 0.06250000000000000000, 0.07499999999999999722, 0.08749999999999999445, 0.1000000000000000056, 0.1125000000000000028, 0.1250000000000000000, 0.1375000000000000111, 0.1499999999999999944, 0.1625000000000000056, 0.1749999999999999889, 0.1875000000000000000, 0.2000000000000000111, 0.2124999999999999944, 0.2250000000000000056, 0.2374999999999999889, 0.2500000000000000000, 0.2625000000000000111, 0.2750000000000000222, 0.2874999999999999778, 0.2999999999999999889, 0.3125000000000000000, 0.3250000000000000111, 0.3375000000000000222, 0.3499999999999999778, 0.3624999999999999889, 0.3750000000000000000, 0.3875000000000000111, 0.4000000000000000222, 0.4124999999999999778, 0.4249999999999999889, 0.4375000000000000000, 0.4500000000000000111, 0.4625000000000000222, 0.4749999999999999778, 0.4874999999999999889, 0.5000000000000000000, 0.5124999999999999556, 0.5250000000000000222, 0.5374999999999999778, 0.5500000000000000444, 0.5625000000000000000, 0.5749999999999999556, 0.5875000000000000222, 0.5999999999999999778, 0.6125000000000000444, 0.6250000000000000000, 0.6374999999999999556, 0.6500000000000000222, 0.6624999999999999778, 0.6750000000000000444, 0.6875000000000000000, 0.6999999999999999556, 0.7125000000000000222, 0.7249999999999999778, 0.7375000000000000444, 0.7500000000000000000, 0.7624999999999999556, 0.7750000000000000222, 0.7874999999999999778, 0.8000000000000000444, 0.8125000000000000000, 0.8249999999999999556, 0.8375000000000000222, 0.8499999999999999778, 0.8625000000000000444, 0.8750000000000000000, 0.8874999999999999556, 0.9000000000000000222, 0.9124999999999999778, 0.9250000000000000444, 0.9375000000000000000, 0.9499999999999999556, 0.9625000000000000222, 0.9749999999999999778, 0.9875000000000000444, 1.000000000000000000 ),
 .UNSPECIFIED. ) 
 CURVE ( )  GEOMETRIC_REPRESENTATION_ITEM ( )  RATIONAL_B_SPLINE_CURVE ( ( 1.000000000000000000, 0.9807852804032304306, 1.000000000000000000, 0.9807852804032304306, 1.000000000000000000, 0.9807852804032304306, 1.000000000000000000, 0.9807852804032304306, 1.000000000000000000, 0.9807852804032304306, 1.000000000000000000, 0.9807852804032304306, 1.000000000000000000, 0.9807852804032304306, 1.000000000000000000, 0.9807852804032304306, 1.000000000000000000, 0.9807852804032304306, 1.000000000000000000, 0.9807852804032304306, 1.000000000000000000, 0.9807852804032304306, 1.000000000000000000, 0.9807852804032304306, 1.000000000000000000, 0.9807852804032304306, 1.000000000000000000, 0.9807852804032304306, 1.000000000000000000, 0.9807852804032304306, 1.000000000000000000, 0.9807852804032304306, 1.000000000000000000, 0.9807852804032304306, 1.000000000000000000, 0.9807852804032304306, 1.000000000000000000, 0.9807852804032304306, 1.000000000000000000, 0.9807852804032304306, 1.000000000000000000, 0.9807852804032304306, 1.000000000000000000, 0.9807852804032304306, 1.000000000000000000, 0.9807852804032304306, 1.000000000000000000, 0.9807852804032304306, 1.000000000000000000, 0.9807852804032304306, 1.000000000000000000, 0.9807852804032304306, 1.000000000000000000, 0.9807852804032304306, 1.000000000000000000, 0.9807852804032304306, 1.000000000000000000, 0.9807852804032304306, 1.000000000000000000, 0.9807852804032304306, 1.000000000000000000, 0.9807852804032304306, 1.000000000000000000, 0.9807852804032304306, 1.000000000000000000, 0.9807852804032304306, 1.000000000000000000, 0.9807852804032304306, 1.000000000000000000, 0.9807852804032304306, 1.000000000000000000, 0.9807852804032304306, 1.000000000000000000, 0.9807852804032304306, 1.000000000000000000, 0.9807852804032304306, 1.000000000000000000, 0.9807852804032304306, 1.000000000000000000, 0.9807852804032304306, 1.000000000000000000, 0.9807852804032304306, 1.000000000000000000, 0.9807852804032304306, 1.000000000000000000, 0.9807852804032304306, 1.000000000000000000, 0.9807852804032304306, 1.000000000000000000, 0.9807852804032304306, 1.000000000000000000, 0.9807852804032304306, 1.000000000000000000, 0.9807852804032304306, 1.000000000000000000, 0.9807852804032304306, 1.000000000000000000, 0.9807852804032304306, 1.000000000000000000, 0.9807852804032304306, 1.000000000000000000, 0.9807852804032304306, 1.000000000000000000, 0.9807852804032304306, 1.000000000000000000, 0.9807852804032304306, 1.000000000000000000, 0.9807852804032304306, 1.000000000000000000, 0.9807852804032304306, 1.000000000000000000, 0.9807852804032304306, 1.000000000000000000, 0.9807852804032304306, 1.000000000000000000, 0.9807852804032304306, 1.000000000000000000, 0.9807852804032304306, 1.000000000000000000, 0.9807852804032304306, 1.000000000000000000, 0.9807852804032304306, 1.000000000000000000, 0.9807852804032304306, 1.000000000000000000, 0.9807852804032304306, 1.000000000000000000, 0.9807852804032304306, 1.000000000000000000, 0.9807852804032304306, 1.000000000000000000, 0.9807852804032304306, 1.000000000000000000, 0.9807852804032304306, 1.000000000000000000, 0.9807852804032304306, 1.000000000000000000, 0.9807852804032304306, 1.000000000000000000, 0.9807852804032304306, 1.000000000000000000, 0.9807852804032304306, 1.000000000000000000, 0.9807852804032304306, 1.000000000000000000, 0.9807852804032304306, 1.000000000000000000, 0.9807852804032304306, 1.000000000000000000, 0.9807852804032304306, 1.000000000000000000, 0.9807852804032304306, 1.000000000000000000, 0.9807852804032304306, 1.000000000000000000, 0.9807852804032304306, 1.000000000000000000, 0.9807852804032304306, 1.000000000000000000, 0.9807852804032304306, 1.000000000000000000 ) ) 
 REPRESENTATION_ITEM ( '' )  );
#14130=CARTESIAN_POINT ( 'NONE',  ( 12.72792205982779734, -12.72792206288791128, -24.54292499981968945 ) ) ;
#14140=EDGE_CURVE ( 'NONE', #1332, #13598, #10604, .T. ) ;
#14149=CARTESIAN_POINT ( 'NONE',  ( 7.500000000000000888, -1.491842755816072952, 10.09333125008778964 ) ) ;
#14155=AXIS2_PLACEMENT_3D ( 'NONE', #10640, #13502, #12007 ) ;
#14160=CARTESIAN_POINT ( 'NONE',  ( 12.72792205982779734, -12.72792206288791128, -13.21332499981968667 ) ) ;
#14163=ORIENTED_EDGE ( 'NONE', *, *, #13772, .F. ) ;
#14176=CARTESIAN_POINT ( 'NONE',  ( -2.943691928843437999, -14.79893867722910450, -9.883926831158460047 ) ) ;
#14181=CARTESIAN_POINT ( 'NONE',  ( -4.248408730893246776, -6.358192987158592047, -24.66135624981969698 ) ) ;
#14182=CARTESIAN_POINT ( 'NONE',  ( -18.00000000043040771, -3.580422610670021211, 6.971918750180310376 ) ) ;
#14192=CARTESIAN_POINT ( 'NONE',  ( -17.99999999999999645, 2.163826221265758470E-09, -11.58354999981969158 ) ) ;
#14197=CARTESIAN_POINT ( 'NONE',  ( 17.50000000000000355, -2.143131898507868643E-15, -40.00000000000000000 ) ) ;
#14200=CARTESIAN_POINT ( 'NONE',  ( 10.19618095047498052, -15.25966317163203456, -3.493793749819690486 ) ) ;
#14204=CARTESIAN_POINT ( 'NONE',  ( 6.330490856366289165, -9.474249098604506258, -26.85745350028680534 ) ) ;
#14205=ORIENTED_EDGE ( 'NONE', *, *, #1832, .T. ) ;
#14221=CARTESIAN_POINT ( 'NONE',  ( -9.474249097082500626, 6.330490858644140850, -6.186296499352570422 ) ) ;
#14222=CARTESIAN_POINT ( 'NONE',  ( 6.358192987158590270, -4.248408730893245000, -17.59260624981969201 ) ) ;
#14229=CARTESIAN_POINT ( 'NONE',  ( -17.99999999956958519, 3.580422614997674113, -20.71401874981969016 ) ) ;
#14234=CARTESIAN_POINT ( 'NONE',  ( 6.358192987158592047, -4.248408730893246776, -8.167606249819693076 ) ) ;
#14236=CARTESIAN_POINT ( 'NONE',  ( -6.358192987158592047, 4.248408730893246776, -3.455106249819692277 ) ) ;
#14252=CARTESIAN_POINT ( 'NONE',  ( -7.500000000000009770, 9.706494115329868228E-15, -7.498799999997683763 ) ) ;
#14255=CARTESIAN_POINT ( 'NONE',  ( -2.163827323447878234E-09, -18.00000000000000000, -12.03519999981969235 ) ) ;
#14268=CARTESIAN_POINT ( 'NONE',  ( -5.663308646854337880, 13.67243654778935991, -15.48002058115845792 ) ) ;
#14270=CARTESIAN_POINT ( 'NONE',  ( -1.491842756249031954, -7.499999999820663454, -15.82541874981969698 ) ) ;
#14282=EDGE_CURVE ( 'NONE', #15394, #6717, #15903, .T. ) ;
#14283=CARTESIAN_POINT ( 'NONE',  ( 6.249999999999902300, -10.82531754730554496, -40.00000000000000000 ) ) ;
#14289=CARTESIAN_POINT ( 'NONE',  ( 15.25966317163202568, 10.19618095047498230, -7.754643749819691401 ) ) ;
#14299=ADVANCED_FACE ( 'NONE', ( #17580 ), #17679, .T. ) ;
#14300=CARTESIAN_POINT ( 'NONE',  ( -10.19618095047498230, 15.25966317163203279, 10.64370625018030836 ) ) ;
#14305=CARTESIAN_POINT ( 'NONE',  ( 4.276731812588566939, -10.32494394809438809, -26.56292225028680676 ) ) ;
#14308=AXIS2_PLACEMENT_3D ( 'NONE', #10268, #9678, #4793 ) ;
#14331=CARTESIAN_POINT ( 'NONE',  ( -9.474249097082500626, 6.330490858644140850, -15.61129649935257646 ) ) ;
#14332=CARTESIAN_POINT ( 'NONE',  ( -6.330490856366290053, 9.474249098604506258, 15.55504649971320141 ) ) ;
#14340=CARTESIAN_POINT ( 'NONE',  ( -2.163827323447878234E-09, -18.00000000000000000, -13.93979999981969087 ) ) ;
#14349=CARTESIAN_POINT ( 'NONE',  ( 5.303300859536631329, 5.303300858261585482, -0.8043249998196909667 ) ) ;
#14380=EDGE_CURVE ( 'NONE', #7721, #1433, #8725, .T. ) ;
#14384=CARTESIAN_POINT ( 'NONE',  ( 10.32494394809439875, 4.276731812588567827, 25.32854725064742851 ) ) ;
#14387=FACE_BOUND ( 'NONE', #3860, .T. ) ;
#14389=CARTESIAN_POINT ( 'NONE',  ( -6.358192988180015881, -4.248408729364577141, -24.07229374981969627 ) ) ;
#14408=CARTESIAN_POINT ( 'NONE',  ( -3.580422614997675890, -17.99999999956958519, -21.16566874981969093 ) ) ;
#14413=CARTESIAN_POINT ( 'NONE',  ( 13.67243654642774686, -5.663308650141536837, -8.138729418480927791 ) ) ;
#14416=VERTEX_POINT ( 'NONE', #14051 ) ;
#14421=EDGE_CURVE ( 'NONE', #6083, #13598, #2801, .T. ) ;
#14436=CARTESIAN_POINT ( 'NONE',  ( 2.222972771497741640, 11.17563879704982988, -4.419108999352573619 ) ) ;
#14437=CARTESIAN_POINT ( 'NONE',  ( 6.929096494179676213, 2.870125741905210415, -19.06526249981969201 ) ) ;
#14443=FACE_OUTER_BOUND ( 'NONE', #13719, .T. ) ;
#14446=CARTESIAN_POINT ( 'NONE',  ( 16.62983158603122291, 6.888301780572502864, -16.88511249981969087 ) ) ;
#14448=ORIENTED_EDGE ( 'NONE', *, *, #14282, .F. ) ;
#14451=AXIS2_PLACEMENT_3D ( 'NONE', #11276, #2806, #7571 ) ;
#14479=EDGE_LOOP ( 'NONE', ( #4814, #11131, #9930, #1800, #18154, #2853, #2190, #20399, #15880, #18043, #13521, #3509, #20204 ) ) ;
#14480=LINE ( 'NONE', #9892, #10616 ) ;
#14489=CARTESIAN_POINT ( 'NONE',  ( -12.54593441764187745, -8.382925368423274293, -18.13080183115846111 ) ) ;
#14492=CARTESIAN_POINT ( 'NONE',  ( 5.303300858261583706, -5.303300859536632217, -17.29807499981969343 ) ) ;
#14513=CARTESIAN_POINT ( 'NONE',  ( 10.19618095047498052, -15.25966317163203456, -22.34379374981969235 ) ) ;
#14517=CARTESIAN_POINT ( 'NONE',  ( -14.79893867722910095, 2.943691928843434891, -3.720760668480927347 ) ) ;
#14522=CARTESIAN_POINT ( 'NONE',  ( -5.303300858261589035, 5.303300859536635770, 21.95432500018031874 ) ) ;
#14537=CARTESIAN_POINT ( 'NONE',  ( 6.929096494179683319, 2.870125741905213079, 15.47463750018031625 ) ) ;
#14538=CARTESIAN_POINT ( 'NONE',  ( 2.222972768810837163, -11.17563879758427525, 2.006608999713197949 ) ) ;
#14547=CARTESIAN_POINT ( 'NONE',  ( -15.25966317163203279, -10.19618095047498052, 17.71245625018031689 ) ) ;
#14564=CARTESIAN_POINT ( 'NONE',  ( -2.870125741905209971, 6.929096494179676213, 6.853487500180312608 ) ) ;
#14574=FACE_OUTER_BOUND ( 'NONE', #2360, .T. ) ;
#14580=CARTESIAN_POINT ( 'NONE',  ( 7.500000000000000000, 9.184850993605147944E-16, -40.00000000000000000 ) ) ;
#14582=CARTESIAN_POINT ( 'NONE',  ( 10.46442989202484064, -10.46442989454075878, -20.78158308115845898 ) ) ;
#14586=ORIENTED_EDGE ( 'NONE', *, *, #294, .F. ) ;
#14587=CARTESIAN_POINT ( 'NONE',  ( 7.500000000000000000, 9.184850993605147944E-16, 40.00000000000000000 ) ) ;
#14588=CARTESIAN_POINT ( 'NONE',  ( 16.62983158603122291, 6.888301780572502864, 22.71948750018031404 ) ) ;
#14597=CARTESIAN_POINT ( 'NONE',  ( 2.870125743571140475, 6.929096493489632635, -4.553487499819687478 ) ) ;
#14602=CARTESIAN_POINT ( 'NONE',  ( 15.25966317163203101, 10.19618095047498585, -5.850043749819691996 ) ) ;
#14608=CARTESIAN_POINT ( 'NONE',  ( 10.46442989454075168, 10.46442989202483886, -0.4809169184809246600 ) ) ;
#14629=CARTESIAN_POINT ( 'NONE',  ( 11.17563879704982632, -2.222972771497745637, -20.91285899935257930 ) ) ;
#14631=CARTESIAN_POINT ( 'NONE',  ( -6.330490856366290053, 9.474249098604506258, -3.294953500286802228 ) ) ;
#14634=FACE_OUTER_BOUND ( 'NONE', #1463, .T. ) ;
#14637=CARTESIAN_POINT ( 'NONE',  ( 3.580422610670020322, -18.00000000043041126, 6.520268750180314044 ) ) ;
#14655=DIRECTION ( 'NONE',  ( -0.000000000000000000, -0.000000000000000000, -1.000000000000000000 ) ) ;
#14657=CARTESIAN_POINT ( 'NONE',  ( 6.358192987158590270, -4.248408730893245000, 10.68239375018031190 ) ) ;
#14666=CARTESIAN_POINT ( 'NONE',  ( 15.25966316918061416, -10.19618095414378622, -22.93285624981968951 ) ) ;
#14668=CARTESIAN_POINT ( 'NONE',  ( 6.888301784570728614, 16.62983158437510056, 19.63676250018031766 ) ) ;
#14674=( BOUNDED_SURFACE ( )  B_SPLINE_SURFACE ( 3, 2, ( 
 ( #4907, #2032, #9982, #17852, #3511, #451, #19425, #11783, #11375, #8093, #16446, #16548, #8391, #3617, #6483, #241, #13174, #19622, #3712, #16345, #5101, #13070, #3321, #19529, #11572, #9781, #16151, #1933, #1836, #14657, #6789, #10091, #14864, #338, #6901, #135, #6587, #5314, #13275, #16247, #1645, #19731, #14564, #9878, #5214, #31, #12970, #11677, #18145, #8483, #5013, #3410, #11474, #8287, #13386, #10505, #13805, #15269, #2140, #19930, #7207, #757, #18350, #12103, #10302, #13580, #10408, #15072, #5723, #5407, #18665, #2448, #20137, #4135, #3816, #980, #11879, #13901, #15490, #10622, #9028, #13693, #651, #7423, #5622, #4028, #8912, #16965, #555, #20251, #16870, #11992, #15383, #16760, #17081, #866, #2242, #18569, #20350, #13487, #5835, #8704, #8599, #7318, #2564, #12196, #12312, #7005, #18782, #10189, #16653, #15173, #2346, #7100, #20029, #5511, #18457, #8795, #3924, #4250, #7749, #4460, #17293, #15904, #12744, #14222, #19100, #9544, #2769, #9234, #14437, #20667, #14015, #6365, #9445, #17196, #18986, #2984, #20883, #10731, #1401, #9339, #11034, #9130, #12524, #20466, #15697, #1513, #4572, #7851, #15802, #2670, #5944, #1306, #6150, #12419, #12638, #4360, #7641, #10928, #15587 ),
 ( #19198, #18894, #16014, #10825, #7964, #12845, #4678, #3079, #17511, #1194, #1084, #14332, #20779, #6261, #11139, #17609, #17405, #7529, #14121, #20574, #6050, #2874, #19603, #213, #13249, #19702, #19394, #16529, #9956, #14737, #317, #6769, #5181, #8462, #6670, #18124, #8069, #10069, #11456, #19500, #4989, #4884, #18016, #11653, #6565, #3385, #3591, #2013, #14943, #11352, #4772, #5078, #19288, #16124, #421, #6872, #11239, #14538, #8371, #17717, #3190, #9659, #1616, #17824, #13153, #4, #6458, #12944, #17924, #3296, #9759, #16224, #1708, #11543, #8158, #14631, #110, #13047, #3482, #9850, #16318, #1810, #8264, #16420, #1906, #14842, #20118, #20230, #2114, #633, #7186, #16942, #8887, #19910, #8777, #8675, #17057, #10381, #6977, #5597, #15247, #2543, #13359, #7297, #18548, #13466, #530, #12078, #961, #5388, #2324, #8572, #845, #4003, #19807, #10486, #11762, #9004, #15470, #3693, #5289, #731, #15048, #5702, #11857, #18326, #15151, #3793, #18228, #11967, #10165, #18437, #16626, #3901, #5489, #10274, #7079, #16737, #2218, #13559, #20005, #16846, #2424, #13669, #10595, #15361, #13779, #18643, #12175, #4111, #9520, #20446, #15883, #17170, #14305, #14204, #6236, #4655, #2745, #9427, #10707 ),
 ( #12606, #20324, #1174, #6127, #17590, #7403, #19073, #12504, #20647, #12286, #15671, #11119, #7731, #11007, #18966, #5810, #2653, #4438, #10904, #15565, #9317, #7503, #10808, #7618, #18761, #2961, #9110, #1379, #4548, #17379, #7826, #1058, #19173, #13990, #3057, #12720, #20749, #15986, #2850, #18868, #13880, #15780, #1282, #17486, #4229, #5925, #14098, #12396, #4342, #17272, #9211, #20550, #6032, #3362, #16396, #1881, #1591, #19673, #13130, #17901, #3459, #9929, #8344, #11627, #9825, #293, #11216, #13224, #14608, #1687, #8135, #8044, #186, #14820, #9735, #6541, #6743, #5152, #18100, #14517, #12826, #11517, #83, #3267, #8238, #17691, #3564, #16293, #3164, #1782, #10044, #4748, #1489, #9636, #14413, #14715, #7938, #6646, #20857, #19269, #13024, #19476, #4961, #6341, #11431, #19579, #19369, #16099, #4859, #5054, #12016, #6434, #17991, #12918, #11329, #17797, #16200, #5464, #10353, #821, #8542, #15024, #5679, #19981, #5264, #18619, #705, #8440, #10247, #15223, #12151, #16510, #7160, #614, #2304, #392, #3766, #11737, #6953, #18206, #7267, #8648, #16711, #2192, #16597, #13642, #3983, #15127, #7057, #13747, #20202, #2400, #2087, #6844, #5568, #13537, #18300, #8756, #3670, #8860, #16822 ),
 ( #11937, #507, #18411, #4082, #13441, #1992, #10145, #3875, #20090, #14916, #13334, #19892, #12049, #19784, #5366, #11835, #18520, #10462, #16919, #15332, #15754, #14072, #7708, #6099, #1030, #17350, #7376, #10680, #15537, #1254, #4315, #2625, #2824, #15645, #18838, #4410, #10877, #7594, #20297, #7478, #20623, #9086, #13961, #20415, #17030, #20523, #10565, #13852, #4520, #14182, #15438, #5780, #9293, #12577, #10985, #2517, #8974, #5900, #6005, #18730, #4203, #930, #12477, #12372, #12256, #17140, #10783, #17245, #2715, #9183, #18941, #19045, #1143, #18692, #15091, #889, #579, #8818, #18266, #5335, #15293, #15405, #3732, #16780, #2367, #12122, #4050, #7029, #3946, #3840, #12222, #5534, #2162, #781, #10431, #4163, #8507, #2476, #13713, #8617, #16675, #20269, #19949, #11898, #2268, #14988, #7229, #473, #11802, #10647, #16989, #6922, #10211, #18590, #8936, #17103, #13406, #19857, #13506, #16891, #5428, #18372, #10321, #670, #8728, #15193, #7343, #7123, #20159, #13826, #10530, #13603, #20052, #5646, #12013, #18479, #5747, #9150, #2897, #12336, #20377, #9363, #9464, #18803, #10845, #17429, #6173, #19120, #15607, #19007, #18912, #6281, #20593, #17215, #15826, #4484, #12769, #2585, #17535, #7769, #2689 ) ),
 .UNSPECIFIED., .F., .F., .T. ) 
 B_SPLINE_SURFACE_WITH_KNOTS ( ( 4, 4 ),
 ( 3, 2, 2, 2, 2, 2, 2, 2, 2, 2, 2, 2, 2, 2, 2, 2, 2, 2, 2, 2, 2, 2, 2, 2, 2, 2, 2, 2, 2, 2, 2, 2, 2, 2, 2, 2, 2, 2, 2, 2, 2, 2, 2, 2, 2, 2, 2, 2, 2, 2, 2, 2, 2, 2, 2, 2, 2, 2, 2, 2, 2, 2, 2, 2, 2, 2, 2, 2, 2, 2, 2, 2, 2, 2, 2, 2, 2, 2, 2, 2, 3 ),
 ( 0.000000000000000000, 1.000000000000000000 ),
 ( 0.000000000000000000, 0.01250000000000000069, 0.02500000000000000139, 0.03749999999999999861, 0.05000000000000000278, 0.06250000000000000000, 0.07499999999999999722, 0.08749999999999999445, 0.1000000000000000056, 0.1125000000000000028, 0.1250000000000000000, 0.1375000000000000111, 0.1499999999999999944, 0.1625000000000000056, 0.1749999999999999889, 0.1875000000000000000, 0.2000000000000000111, 0.2124999999999999944, 0.2250000000000000056, 0.2374999999999999889, 0.2500000000000000000, 0.2625000000000000111, 0.2750000000000000222, 0.2874999999999999778, 0.2999999999999999889, 0.3125000000000000000, 0.3250000000000000111, 0.3375000000000000222, 0.3499999999999999778, 0.3624999999999999889, 0.3750000000000000000, 0.3875000000000000111, 0.4000000000000000222, 0.4124999999999999778, 0.4249999999999999889, 0.4375000000000000000, 0.4500000000000000111, 0.4625000000000000222, 0.4749999999999999778, 0.4874999999999999889, 0.5000000000000000000, 0.5124999999999999556, 0.5250000000000000222, 0.5374999999999999778, 0.5500000000000000444, 0.5625000000000000000, 0.5749999999999999556, 0.5875000000000000222, 0.5999999999999999778, 0.6125000000000000444, 0.6250000000000000000, 0.6374999999999999556, 0.6500000000000000222, 0.6624999999999999778, 0.6750000000000000444, 0.6875000000000000000, 0.6999999999999999556, 0.7125000000000000222, 0.7249999999999999778, 0.7375000000000000444, 0.7500000000000000000, 0.7624999999999999556, 0.7750000000000000222, 0.7874999999999999778, 0.8000000000000000444, 0.8125000000000000000, 0.8249999999999999556, 0.8375000000000000222, 0.8499999999999999778, 0.8625000000000000444, 0.8750000000000000000, 0.8874999999999999556, 0.9000000000000000222, 0.9124999999999999778, 0.9250000000000000444, 0.9375000000000000000, 0.9499999999999999556, 0.9625000000000000222, 0.9749999999999999778, 0.9875000000000000444, 1.000000000000000000 ),
 .UNSPECIFIED. ) 
 GEOMETRIC_REPRESENTATION_ITEM ( )  RATIONAL_B_SPLINE_SURFACE ( (
 ( 1.000000000000000000, 0.9807852804032304306, 1.000000000000000000, 0.9807852804032304306, 1.000000000000000000, 0.9807852804032304306, 1.000000000000000000, 0.9807852804032304306, 1.000000000000000000, 0.9807852804032304306, 1.000000000000000000, 0.9807852804032304306, 1.000000000000000000, 0.9807852804032304306, 1.000000000000000000, 0.9807852804032304306, 1.000000000000000000, 0.9807852804032304306, 1.000000000000000000, 0.9807852804032304306, 1.000000000000000000, 0.9807852804032304306, 1.000000000000000000, 0.9807852804032304306, 1.000000000000000000, 0.9807852804032304306, 1.000000000000000000, 0.9807852804032304306, 1.000000000000000000, 0.9807852804032304306, 1.000000000000000000, 0.9807852804032304306, 1.000000000000000000, 0.9807852804032304306, 1.000000000000000000, 0.9807852804032304306, 1.000000000000000000, 0.9807852804032304306, 1.000000000000000000, 0.9807852804032304306, 1.000000000000000000, 0.9807852804032304306, 1.000000000000000000, 0.9807852804032304306, 1.000000000000000000, 0.9807852804032304306, 1.000000000000000000, 0.9807852804032304306, 1.000000000000000000, 0.9807852804032304306, 1.000000000000000000, 0.9807852804032304306, 1.000000000000000000, 0.9807852804032304306, 1.000000000000000000, 0.9807852804032304306, 1.000000000000000000, 0.9807852804032304306, 1.000000000000000000, 0.9807852804032304306, 1.000000000000000000, 0.9807852804032304306, 1.000000000000000000, 0.9807852804032304306, 1.000000000000000000, 0.9807852804032304306, 1.000000000000000000, 0.9807852804032304306, 1.000000000000000000, 0.9807852804032304306, 1.000000000000000000, 0.9807852804032304306, 1.000000000000000000, 0.9807852804032304306, 1.000000000000000000, 0.9807852804032304306, 1.000000000000000000, 0.9807852804032304306, 1.000000000000000000, 0.9807852804032304306, 1.000000000000000000, 0.9807852804032304306, 1.000000000000000000, 0.9807852804032304306, 1.000000000000000000, 0.9807852804032304306, 1.000000000000000000, 0.9807852804032304306, 1.000000000000000000, 0.9807852804032304306, 1.000000000000000000, 0.9807852804032304306, 1.000000000000000000, 0.9807852804032304306, 1.000000000000000000, 0.9807852804032304306, 1.000000000000000000, 0.9807852804032304306, 1.000000000000000000, 0.9807852804032304306, 1.000000000000000000, 0.9807852804032304306, 1.000000000000000000, 0.9807852804032304306, 1.000000000000000000, 0.9807852804032304306, 1.000000000000000000, 0.9807852804032304306, 1.000000000000000000, 0.9807852804032304306, 1.000000000000000000, 0.9807852804032304306, 1.000000000000000000, 0.9807852804032304306, 1.000000000000000000, 0.9807852804032304306, 1.000000000000000000, 0.9807852804032304306, 1.000000000000000000, 0.9807852804032304306, 1.000000000000000000, 0.9807852804032304306, 1.000000000000000000, 0.9807852804032304306, 1.000000000000000000, 0.9807852804032304306, 1.000000000000000000, 0.9807852804032304306, 1.000000000000000000, 0.9807852804032304306, 1.000000000000000000, 0.9807852804032304306, 1.000000000000000000, 0.9807852804032304306, 1.000000000000000000, 0.9807852804032304306, 1.000000000000000000, 0.9807852804032304306, 1.000000000000000000, 0.9807852804032304306, 1.000000000000000000, 0.9807852804032304306, 1.000000000000000000, 0.9807852804032304306, 1.000000000000000000, 0.9807852804032304306, 1.000000000000000000, 0.9807852804032304306, 1.000000000000000000, 0.9807852804032304306, 1.000000000000000000, 0.9807852804032304306, 1.000000000000000000, 0.9807852804032304306, 1.000000000000000000, 0.9807852804032304306, 1.000000000000000000, 0.9807852804032304306, 1.000000000000000000, 0.9807852804032304306, 1.000000000000000000),
 ( 0.9659702800374152520, 0.9474094319676833464, 0.9659702800374152520, 0.9474094319676833464, 0.9659702800374152520, 0.9474094319676833464, 0.9659702800374152520, 0.9474094319676833464, 0.9659702800374152520, 0.9474094319676833464, 0.9659702800374152520, 0.9474094319676833464, 0.9659702800374152520, 0.9474094319676833464, 0.9659702800374152520, 0.9474094319676833464, 0.9659702800374152520, 0.9474094319676833464, 0.9659702800374152520, 0.9474094319676833464, 0.9659702800374152520, 0.9474094319676833464, 0.9659702800374152520, 0.9474094319676833464, 0.9659702800374152520, 0.9474094319676833464, 0.9659702800374152520, 0.9474094319676833464, 0.9659702800374152520, 0.9474094319676833464, 0.9659702800374152520, 0.9474094319676833464, 0.9659702800374152520, 0.9474094319676833464, 0.9659702800374152520, 0.9474094319676833464, 0.9659702800374152520, 0.9474094319676833464, 0.9659702800374152520, 0.9474094319676833464, 0.9659702800374152520, 0.9474094319676833464, 0.9659702800374152520, 0.9474094319676833464, 0.9659702800374152520, 0.9474094319676833464, 0.9659702800374152520, 0.9474094319676833464, 0.9659702800374152520, 0.9474094319676833464, 0.9659702800374152520, 0.9474094319676833464, 0.9659702800374152520, 0.9474094319676833464, 0.9659702800374152520, 0.9474094319676833464, 0.9659702800374152520, 0.9474094319676833464, 0.9659702800374152520, 0.9474094319676833464, 0.9659702800374152520, 0.9474094319676833464, 0.9659702800374152520, 0.9474094319676833464, 0.9659702800374152520, 0.9474094319676833464, 0.9659702800374152520, 0.9474094319676833464, 0.9659702800374152520, 0.9474094319676833464, 0.9659702800374152520, 0.9474094319676833464, 0.9659702800374152520, 0.9474094319676833464, 0.9659702800374152520, 0.9474094319676833464, 0.9659702800374152520, 0.9474094319676833464, 0.9659702800374152520, 0.9474094319676833464, 0.9659702800374152520, 0.9474094319676833464, 0.9659702800374152520, 0.9474094319676833464, 0.9659702800374152520, 0.9474094319676833464, 0.9659702800374152520, 0.9474094319676833464, 0.9659702800374152520, 0.9474094319676833464, 0.9659702800374152520, 0.9474094319676833464, 0.9659702800374152520, 0.9474094319676833464, 0.9659702800374152520, 0.9474094319676833464, 0.9659702800374152520, 0.9474094319676833464, 0.9659702800374152520, 0.9474094319676833464, 0.9659702800374152520, 0.9474094319676833464, 0.9659702800374152520, 0.9474094319676833464, 0.9659702800374152520, 0.9474094319676833464, 0.9659702800374152520, 0.9474094319676833464, 0.9659702800374152520, 0.9474094319676833464, 0.9659702800374152520, 0.9474094319676833464, 0.9659702800374152520, 0.9474094319676833464, 0.9659702800374152520, 0.9474094319676833464, 0.9659702800374152520, 0.9474094319676833464, 0.9659702800374152520, 0.9474094319676833464, 0.9659702800374152520, 0.9474094319676833464, 0.9659702800374152520, 0.9474094319676833464, 0.9659702800374152520, 0.9474094319676833464, 0.9659702800374152520, 0.9474094319676833464, 0.9659702800374152520, 0.9474094319676833464, 0.9659702800374152520, 0.9474094319676833464, 0.9659702800374152520, 0.9474094319676833464, 0.9659702800374152520, 0.9474094319676833464, 0.9659702800374152520, 0.9474094319676833464, 0.9659702800374152520, 0.9474094319676833464, 0.9659702800374152520, 0.9474094319676833464, 0.9659702800374152520, 0.9474094319676833464, 0.9659702800374152520, 0.9474094319676833464, 0.9659702800374152520, 0.9474094319676833464, 0.9659702800374152520, 0.9474094319676833464, 0.9659702800374152520, 0.9474094319676833464, 0.9659702800374152520, 0.9474094319676833464, 0.9659702800374152520, 0.9474094319676833464, 0.9659702800374152520, 0.9474094319676833464, 0.9659702800374152520, 0.9474094319676833464, 0.9659702800374152520),
 ( 0.9659702800374152520, 0.9474094319676833464, 0.9659702800374152520, 0.9474094319676833464, 0.9659702800374152520, 0.9474094319676833464, 0.9659702800374152520, 0.9474094319676833464, 0.9659702800374152520, 0.9474094319676833464, 0.9659702800374152520, 0.9474094319676833464, 0.9659702800374152520, 0.9474094319676833464, 0.9659702800374152520, 0.9474094319676833464, 0.9659702800374152520, 0.9474094319676833464, 0.9659702800374152520, 0.9474094319676833464, 0.9659702800374152520, 0.9474094319676833464, 0.9659702800374152520, 0.9474094319676833464, 0.9659702800374152520, 0.9474094319676833464, 0.9659702800374152520, 0.9474094319676833464, 0.9659702800374152520, 0.9474094319676833464, 0.9659702800374152520, 0.9474094319676833464, 0.9659702800374152520, 0.9474094319676833464, 0.9659702800374152520, 0.9474094319676833464, 0.9659702800374152520, 0.9474094319676833464, 0.9659702800374152520, 0.9474094319676833464, 0.9659702800374152520, 0.9474094319676833464, 0.9659702800374152520, 0.9474094319676833464, 0.9659702800374152520, 0.9474094319676833464, 0.9659702800374152520, 0.9474094319676833464, 0.9659702800374152520, 0.9474094319676833464, 0.9659702800374152520, 0.9474094319676833464, 0.9659702800374152520, 0.9474094319676833464, 0.9659702800374152520, 0.9474094319676833464, 0.9659702800374152520, 0.9474094319676833464, 0.9659702800374152520, 0.9474094319676833464, 0.9659702800374152520, 0.9474094319676833464, 0.9659702800374152520, 0.9474094319676833464, 0.9659702800374152520, 0.9474094319676833464, 0.9659702800374152520, 0.9474094319676833464, 0.9659702800374152520, 0.9474094319676833464, 0.9659702800374152520, 0.9474094319676833464, 0.9659702800374152520, 0.9474094319676833464, 0.9659702800374152520, 0.9474094319676833464, 0.9659702800374152520, 0.9474094319676833464, 0.9659702800374152520, 0.9474094319676833464, 0.9659702800374152520, 0.9474094319676833464, 0.9659702800374152520, 0.9474094319676833464, 0.9659702800374152520, 0.9474094319676833464, 0.9659702800374152520, 0.9474094319676833464, 0.9659702800374152520, 0.9474094319676833464, 0.9659702800374152520, 0.9474094319676833464, 0.9659702800374152520, 0.9474094319676833464, 0.9659702800374152520, 0.9474094319676833464, 0.9659702800374152520, 0.9474094319676833464, 0.9659702800374152520, 0.9474094319676833464, 0.9659702800374152520, 0.9474094319676833464, 0.9659702800374152520, 0.9474094319676833464, 0.9659702800374152520, 0.9474094319676833464, 0.9659702800374152520, 0.9474094319676833464, 0.9659702800374152520, 0.9474094319676833464, 0.9659702800374152520, 0.9474094319676833464, 0.9659702800374152520, 0.9474094319676833464, 0.9659702800374152520, 0.9474094319676833464, 0.9659702800374152520, 0.9474094319676833464, 0.9659702800374152520, 0.9474094319676833464, 0.9659702800374152520, 0.9474094319676833464, 0.9659702800374152520, 0.9474094319676833464, 0.9659702800374152520, 0.9474094319676833464, 0.9659702800374152520, 0.9474094319676833464, 0.9659702800374152520, 0.9474094319676833464, 0.9659702800374152520, 0.9474094319676833464, 0.9659702800374152520, 0.9474094319676833464, 0.9659702800374152520, 0.9474094319676833464, 0.9659702800374152520, 0.9474094319676833464, 0.9659702800374152520, 0.9474094319676833464, 0.9659702800374152520, 0.9474094319676833464, 0.9659702800374152520, 0.9474094319676833464, 0.9659702800374152520, 0.9474094319676833464, 0.9659702800374152520, 0.9474094319676833464, 0.9659702800374152520, 0.9474094319676833464, 0.9659702800374152520, 0.9474094319676833464, 0.9659702800374152520, 0.9474094319676833464, 0.9659702800374152520, 0.9474094319676833464, 0.9659702800374152520, 0.9474094319676833464, 0.9659702800374152520, 0.9474094319676833464, 0.9659702800374152520),
 ( 1.000000000000000000, 0.9807852804032304306, 1.000000000000000000, 0.9807852804032304306, 1.000000000000000000, 0.9807852804032304306, 1.000000000000000000, 0.9807852804032304306, 1.000000000000000000, 0.9807852804032304306, 1.000000000000000000, 0.9807852804032304306, 1.000000000000000000, 0.9807852804032304306, 1.000000000000000000, 0.9807852804032304306, 1.000000000000000000, 0.9807852804032304306, 1.000000000000000000, 0.9807852804032304306, 1.000000000000000000, 0.9807852804032304306, 1.000000000000000000, 0.9807852804032304306, 1.000000000000000000, 0.9807852804032304306, 1.000000000000000000, 0.9807852804032304306, 1.000000000000000000, 0.9807852804032304306, 1.000000000000000000, 0.9807852804032304306, 1.000000000000000000, 0.9807852804032304306, 1.000000000000000000, 0.9807852804032304306, 1.000000000000000000, 0.9807852804032304306, 1.000000000000000000, 0.9807852804032304306, 1.000000000000000000, 0.9807852804032304306, 1.000000000000000000, 0.9807852804032304306, 1.000000000000000000, 0.9807852804032304306, 1.000000000000000000, 0.9807852804032304306, 1.000000000000000000, 0.9807852804032304306, 1.000000000000000000, 0.9807852804032304306, 1.000000000000000000, 0.9807852804032304306, 1.000000000000000000, 0.9807852804032304306, 1.000000000000000000, 0.9807852804032304306, 1.000000000000000000, 0.9807852804032304306, 1.000000000000000000, 0.9807852804032304306, 1.000000000000000000, 0.9807852804032304306, 1.000000000000000000, 0.9807852804032304306, 1.000000000000000000, 0.9807852804032304306, 1.000000000000000000, 0.9807852804032304306, 1.000000000000000000, 0.9807852804032304306, 1.000000000000000000, 0.9807852804032304306, 1.000000000000000000, 0.9807852804032304306, 1.000000000000000000, 0.9807852804032304306, 1.000000000000000000, 0.9807852804032304306, 1.000000000000000000, 0.9807852804032304306, 1.000000000000000000, 0.9807852804032304306, 1.000000000000000000, 0.9807852804032304306, 1.000000000000000000, 0.9807852804032304306, 1.000000000000000000, 0.9807852804032304306, 1.000000000000000000, 0.9807852804032304306, 1.000000000000000000, 0.9807852804032304306, 1.000000000000000000, 0.9807852804032304306, 1.000000000000000000, 0.9807852804032304306, 1.000000000000000000, 0.9807852804032304306, 1.000000000000000000, 0.9807852804032304306, 1.000000000000000000, 0.9807852804032304306, 1.000000000000000000, 0.9807852804032304306, 1.000000000000000000, 0.9807852804032304306, 1.000000000000000000, 0.9807852804032304306, 1.000000000000000000, 0.9807852804032304306, 1.000000000000000000, 0.9807852804032304306, 1.000000000000000000, 0.9807852804032304306, 1.000000000000000000, 0.9807852804032304306, 1.000000000000000000, 0.9807852804032304306, 1.000000000000000000, 0.9807852804032304306, 1.000000000000000000, 0.9807852804032304306, 1.000000000000000000, 0.9807852804032304306, 1.000000000000000000, 0.9807852804032304306, 1.000000000000000000, 0.9807852804032304306, 1.000000000000000000, 0.9807852804032304306, 1.000000000000000000, 0.9807852804032304306, 1.000000000000000000, 0.9807852804032304306, 1.000000000000000000, 0.9807852804032304306, 1.000000000000000000, 0.9807852804032304306, 1.000000000000000000, 0.9807852804032304306, 1.000000000000000000, 0.9807852804032304306, 1.000000000000000000, 0.9807852804032304306, 1.000000000000000000, 0.9807852804032304306, 1.000000000000000000, 0.9807852804032304306, 1.000000000000000000, 0.9807852804032304306, 1.000000000000000000, 0.9807852804032304306, 1.000000000000000000, 0.9807852804032304306, 1.000000000000000000, 0.9807852804032304306, 1.000000000000000000, 0.9807852804032304306, 1.000000000000000000) ) ) 
 REPRESENTATION_ITEM ( '' )  SURFACE ( )  );
#14684=CARTESIAN_POINT ( 'NONE',  ( 13.67243654778935991, 5.663308646854338768, -13.12377058115845863 ) ) ;
#14687=EDGE_CURVE ( 'NONE', #19384, #10000, #1496, .T. ) ;
#14692=CARTESIAN_POINT ( 'NONE',  ( -10.19618095047498052, 15.25966317163203101, 20.06870625018031262 ) ) ;
#14710=CARTESIAN_POINT ( 'NONE',  ( -2.163827323447878648E-09, -18.00000000000000355, -12.03519999981969590 ) ) ;
#14713=CARTESIAN_POINT ( 'NONE',  ( -7.500000000000000888, -3.289131931895657122E-15, 5.086300000002307087 ) ) ;
#14715=CARTESIAN_POINT ( 'NONE',  ( 14.79893867722909917, -2.943691928843437111, -8.433260668480928146 ) ) ;
#14732=CARTESIAN_POINT ( 'NONE',  ( 10.19618095414378978, 15.25966316918061771, -15.86410624981969697 ) ) ;
#14735=CARTESIAN_POINT ( 'NONE',  ( 7.500000000179346316, 1.491842754445843244, 15.76916875018031305 ) ) ;
#14737=CARTESIAN_POINT ( 'NONE',  ( 9.474249097082495297, -6.330490858644137298, 10.25348399971320035 ) ) ;
#14743=CARTESIAN_POINT ( 'NONE',  ( -17.99999999956958519, 3.580422614997674113, 9.465581250180312267 ) ) ;
#14746=CARTESIAN_POINT ( 'NONE',  ( -12.50000000000000533, 0.000000000000000000, -40.00000000000000000 ) ) ;
#14748=DIRECTION ( 'NONE',  ( 0.000000000000000000, 0.000000000000000000, 1.000000000000000000 ) ) ;
#14762=FACE_OUTER_BOUND ( 'NONE', #20586, .T. ) ;
#14785=CARTESIAN_POINT ( 'NONE',  ( -2.222972768810837607, 11.17563879758428769, 4.416828500647428157 ) ) ;
#14814=CARTESIAN_POINT ( 'NONE',  ( -16.62983158437510411, 6.888301784570731279, -18.51488749981969306 ) ) ;
#14817=CARTESIAN_POINT ( 'NONE',  ( -12.50000000000000533, 0.000000000000000000, 40.00000000000000000 ) ) ;
#14820=CARTESIAN_POINT ( 'NONE',  ( -2.943691925285395694, 14.79893867793683349, -1.953573168480927214 ) ) ;
#14841=CARTESIAN_POINT ( 'NONE',  ( 2.870125741905214412, -6.929096494179682431, 17.83088750018031732 ) ) ;
#14842=CARTESIAN_POINT ( 'NONE',  ( -6.330490858644137298, -9.474249097082495297, -6.240266000286802672 ) ) ;
#14847=CARTESIAN_POINT ( 'NONE',  ( -15.25966317163203279, -10.19618095047498052, 8.287456250180312622 ) ) ;
#14859=FILL_AREA_STYLE ('',( #6897 ) ) ;
#14864=CARTESIAN_POINT ( 'NONE',  ( 7.500000000000000888, -9.015933403756337545E-10, 9.798800000180312608 ) ) ;
#14866=DIRECTION ( 'NONE',  ( -0.000000000000000000, -0.000000000000000000, -1.000000000000000000 ) ) ;
#14877=FACE_BOUND ( 'NONE', #57, .T. ) ;
#14882=VECTOR ( 'NONE', #4059, 1000.000000000000000 ) ;
#14884=CARTESIAN_POINT ( 'NONE',  ( 11.17563879758428769, 2.222972768810838939, 6.773078500647428335 ) ) ;
#14893=CARTESIAN_POINT ( 'NONE',  ( 2.163825119083639534E-09, 18.00000000000000000, 2.102300000180311823 ) ) ;
#14908=CARTESIAN_POINT ( 'NONE',  ( 2.943691925285398803, -14.79893867793684059, 8.377010668841545993 ) ) ;
#14910=ORIENTED_EDGE ( 'NONE', *, *, #2506, .F. ) ;
#14916=CARTESIAN_POINT ( 'NONE',  ( -3.580422610670017658, 18.00000000043040771, 18.75316875018031126 ) ) ;
#14928=CARTESIAN_POINT ( 'NONE',  ( -17.99999999999999645, 2.163826221265758470E-09, -2.158549999819691312 ) ) ;
#14938=CARTESIAN_POINT ( 'NONE',  ( 15.25966317163203101, 10.19618095047498585, 22.42495625018030836 ) ) ;
#14942=CARTESIAN_POINT ( 'NONE',  ( 5.303300859536635770, 5.303300858261589923, 14.88557500018031554 ) ) ;
#14943=CARTESIAN_POINT ( 'NONE',  ( -11.17563879731704723, 1.343452237168308679E-09, 4.657390249713198926 ) ) ;
#14947=AXIS2_PLACEMENT_3D ( 'NONE', #12373, #4317, #10785 ) ;
#14950=CARTESIAN_POINT ( 'NONE',  ( 16.62983158603122291, 6.888301780572502864, 22.71948750018031404 ) ) ;
#14958=VERTEX_POINT ( 'NONE', #8618 ) ;
#14968=FACE_OUTER_BOUND ( 'NONE', #8317, .T. ) ;
#14988=CARTESIAN_POINT ( 'NONE',  ( -3.580422610670017658, 18.00000000043040771, -9.521831249819690868 ) ) ;
#14991=CARTESIAN_POINT ( 'NONE',  ( -6.330490856366295382, 9.474249098604511587, 13.25276600064742993 ) ) ;
#14999=EDGE_CURVE ( 'NONE', #17243, #7832, #5647, .T. ) ;
#15000=CARTESIAN_POINT ( 'NONE',  ( -12.72792205982779912, 12.72792206288790950, 0.9241750001803133996 ) ) ;
#15017=CARTESIAN_POINT ( 'NONE',  ( 13.67243654778935991, 5.663308646854338768, 15.15122941884154883 ) ) ;
#15024=CARTESIAN_POINT ( 'NONE',  ( 2.943691925285397470, -14.79893867793683349, -16.09107316848092140 ) ) ;
#15025=AXIS2_PLACEMENT_3D ( 'NONE', #4290, #1126, #15938 ) ;
#15036=CARTESIAN_POINT ( 'NONE',  ( 16.62983158437509346, -6.888301784570737496, 3.143012500180311086 ) ) ;
#15037=EDGE_CURVE ( 'NONE', #6083, #8981, #11986, .T. ) ;
#15039=ORIENTED_EDGE ( 'NONE', *, *, #7940, .T. ) ;
#15045=CARTESIAN_POINT ( 'NONE',  ( -3.580422610670018990, 18.00000000043041481, 20.65776875018030978 ) ) ;
#15047=CARTESIAN_POINT ( 'NONE',  ( 6.358192987158595599, -4.248408730893249441, 7.522293750180316430 ) ) ;
#15048=CARTESIAN_POINT ( 'NONE',  ( 4.276731812588566939, -10.32494394809438809, -17.13792225028680249 ) ) ;
#15055=CARTESIAN_POINT ( 'NONE',  ( 3.580422610670020322, -18.00000000043041126, -2.904731249819686223 ) ) ;
#15071=DIRECTION ( 'NONE',  ( 0.000000000000000000, 0.000000000000000000, -1.000000000000000000 ) ) ;
#15072=CARTESIAN_POINT ( 'NONE',  ( 6.358192988180013216, 4.248408729364577141, -0.5097937498196903894 ) ) ;
#15080=CARTESIAN_POINT ( 'NONE',  ( 3.580422614997668340, 17.99999999956958519, 0.4922312501803131624 ) ) ;
#15091=CARTESIAN_POINT ( 'NONE',  ( -6.888301780572500199, 16.62983158603121936, -0.3913624998196918447 ) ) ;
#15094=DIRECTION ( 'NONE',  ( -0.000000000000000000, -0.000000000000000000, 1.000000000000000000 ) ) ;
#15095=CARTESIAN_POINT ( 'NONE',  ( 10.32494394809439875, 4.276731812588567827, 6.478547250647427980 ) ) ;
#15100=CARTESIAN_POINT ( 'NONE',  ( 12.92641286132474931, -1.553915700095510638E-09, 25.24826151322289647 ) ) ;
#15101=EDGE_LOOP ( 'NONE', ( #18759, #15683 ) ) ;
#15104=CARTESIAN_POINT ( 'NONE',  ( -16.62983158437510056, 6.888301784570729502, 0.3351125001803123560 ) ) ;
#15116=EDGE_CURVE ( 'NONE', #7136, #1316, #6238, .T. ) ;
#15121=CARTESIAN_POINT ( 'NONE',  ( -13.67243654778936168, -5.663308646854336992, 10.43872941884154493 ) ) ;
#15122=ORIENTED_EDGE ( 'NONE', *, *, #18433, .T. ) ;
#15125=DIRECTION ( 'NONE',  ( 0.000000000000000000, 0.000000000000000000, 1.000000000000000000 ) ) ;
#15127=CARTESIAN_POINT ( 'NONE',  ( -12.54593441764187034, -8.382925368423267187, -23.74888566848093774 ) ) ;
#15133=ORIENTED_EDGE ( 'NONE', *, *, #17892, .T. ) ;
#15135=DIRECTION ( 'NONE',  ( 0.000000000000000000, 0.000000000000000000, 1.000000000000000000 ) ) ;
#15136=CARTESIAN_POINT ( 'NONE',  ( -10.19618095414378445, -15.25966316918061239, 5.793793750180310731 ) ) ;
#15137=CIRCLE ( 'NONE', #16817, 17.00000000000002842 ) ;
#15145=CARTESIAN_POINT ( 'NONE',  ( 6.888301784570730391, 16.62983158437510411, 21.54136250018031262 ) ) ;
#15147=CARTESIAN_POINT ( 'NONE',  ( -9.015947181032835626E-10, -7.500000000000007994, -0.4300499998196871676 ) ) ;
#15151=CARTESIAN_POINT ( 'NONE',  ( 10.32494394706615637, -4.276731815070946574, -18.31604725028681102 ) ) ;
#15158=CARTESIAN_POINT ( 'NONE',  ( -12.72792205982779912, 12.72792206288790950, 0.9241750001803133996 ) ) ;
#15173=CARTESIAN_POINT ( 'NONE',  ( -7.499999999820661678, 1.491842756249031288, -13.46916874981968881 ) ) ;
#15180=LINE ( 'NONE', #6908, #4796 ) ;
#15181=VERTEX_POINT ( 'NONE', #5098 ) ;
#15183=CARTESIAN_POINT ( 'NONE',  ( 17.99999999956958163, -3.580422614997676334, 12.27348125018031411 ) ) ;
#15186=CARTESIAN_POINT ( 'NONE',  ( -7.500000000000000000, 0.000000000000000000, 40.00000000000000000 ) ) ;
#15193=CARTESIAN_POINT ( 'NONE',  ( 15.25966316918061239, -10.19618095414378445, -15.41245624981969087 ) ) ;
#15197=CARTESIAN_POINT ( 'NONE',  ( 10.32494394706616347, -4.276731815070950127, 17.08167225064743278 ) ) ;
#15205=CARTESIAN_POINT ( 'NONE',  ( 12.72792206288790950, 12.72792205982780089, 12.70542500018031262 ) ) ;
#15215=DIRECTION ( 'NONE',  ( -0.000000000000000000, -0.000000000000000000, -1.000000000000000000 ) ) ;
#15218=CARTESIAN_POINT ( 'NONE',  ( 12.54593441562640876, -8.382925371439629458, 16.62388566884154528 ) ) ;
#15223=CARTESIAN_POINT ( 'NONE',  ( 14.79893867793683349, 2.943691925285396582, -18.44732316848092779 ) ) ;
#15234=CARTESIAN_POINT ( 'NONE',  ( -16.62983158437509701, 6.888301784570728614, -1.569487499819690379 ) ) ;
#15236=ORIENTED_EDGE ( 'NONE', *, *, #6643, .T. ) ;
#15242=CARTESIAN_POINT ( 'NONE',  ( 18.00000000000000355, -2.163824016901520597E-09, 23.30855000018031120 ) ) ;
#15244=CARTESIAN_POINT ( 'NONE',  ( -7.500000000179346316, -1.491842754445844355, 1.631668750180312877 ) ) ;
#15247=CARTESIAN_POINT ( 'NONE',  ( 7.902369978624323110, 7.902369976724394895, -10.65823475028680356 ) ) ;
#15253=AXIS2_PLACEMENT_3D ( 'NONE', #15100, #19758, #19957 ) ;
#15254=CARTESIAN_POINT ( 'NONE',  ( 15.25966317163202746, 10.19618095047498407, -5.850043749819688443 ) ) ;
#15269=CARTESIAN_POINT ( 'NONE',  ( 1.491842754445842134, -7.500000000179339210, 2.435518750180311276 ) ) ;
#15277=CARTESIAN_POINT ( 'NONE',  ( -15.25966317163203279, -10.19618095047498052, 6.382856250180313218 ) ) ;
#15292=CARTESIAN_POINT ( 'NONE',  ( 7.500000000000004441, -8.788009017158368372E-15, -9.051199999997692203 ) ) ;
#15293=CARTESIAN_POINT ( 'NONE',  ( -17.99999999999999645, 2.163826221265758470E-09, -2.158549999819691312 ) ) ;
#15297=CARTESIAN_POINT ( 'NONE',  ( -6.330490856366295382, 9.474249098604511587, -5.597233999352570599 ) ) ;
#15307=CARTESIAN_POINT ( 'NONE',  ( 12.72792206288790950, 12.72792205982780089, 3.280425000180314132 ) ) ;
#15327=CARTESIAN_POINT ( 'NONE',  ( 5.663308650141532397, 13.67243654642775574, 23.39810441884155168 ) ) ;
#15332=CARTESIAN_POINT ( 'NONE',  ( -15.25966317163202923, -10.19618095047497874, 15.80785625018031304 ) ) ;
#15344=CARTESIAN_POINT ( 'NONE',  ( -6.888301784570736608, -16.62983158437509346, 5.499262500180311264 ) ) ;
#15353=CARTESIAN_POINT ( 'NONE',  ( -18.00000000000000355, 2.163826221265759298E-09, 18.59605000018030907 ) ) ;
#15359=CARTESIAN_POINT ( 'NONE',  ( 1.491842754445843688, -7.500000000179346316, 8.700418750180315186 ) ) ;
#15361=CARTESIAN_POINT ( 'NONE',  ( -11.17563879758427525, -2.222972768810838051, -23.91214100028680889 ) ) ;
#15367=CARTESIAN_POINT ( 'NONE',  ( 3.580422610670020322, -18.00000000043041126, -12.32973124981968560 ) ) ;
#15383=CARTESIAN_POINT ( 'NONE',  ( 5.303300858261582817, -5.303300859536631329, -7.873074999819689168 ) ) ;
#15391=CARTESIAN_POINT ( 'NONE',  ( 10.19618095414378800, 15.25966316918061416, 10.50629375018031375 ) ) ;
#15394=VERTEX_POINT ( 'NONE', #17078 ) ;
#15405=CARTESIAN_POINT ( 'NONE',  ( -18.00000000043040771, -3.580422610670021211, -2.453081249819692111 ) ) ;
#15408=CARTESIAN_POINT ( 'NONE',  ( 10.32494394706616347, -4.276731815070950127, -1.768327749352573308 ) ) ;
#15411=DIRECTION ( 'NONE',  ( -0.000000000000000000, -0.000000000000000000, 1.000000000000000000 ) ) ;
#15417=CARTESIAN_POINT ( 'NONE',  ( 16.62983158437509346, -6.888301784570739272, -4.377387499819689332 ) ) ;
#15431=CARTESIAN_POINT ( 'NONE',  ( 10.46442989454075700, 10.46442989202484419, 5.137166918841548302 ) ) ;
#15438=CARTESIAN_POINT ( 'NONE',  ( -16.62983158603121936, -6.888301780572499311, 6.677387500180310020 ) ) ;
#15452=CARTESIAN_POINT ( 'NONE',  ( 16.62983158603121936, 6.888301780572501976, -16.88511249981969442 ) ) ;
#15460=CARTESIAN_POINT ( 'NONE',  ( 7.500000000000009770, -8.788009017158368372E-15, -2.786299999997682519 ) ) ;
#15464=CARTESIAN_POINT ( 'NONE',  ( -12.72792206288791483, -12.72792205982780089, 7.992925000180310491 ) ) ;
#15467=CARTESIAN_POINT ( 'NONE',  ( 6.929096494179683319, 2.870125741905213079, -3.375362499819685613 ) ) ;
#15470=CARTESIAN_POINT ( 'NONE',  ( -4.276731815070945686, -10.32494394706615637, -15.95979725028680996 ) ) ;
#15475=CARTESIAN_POINT ( 'NONE',  ( 7.500000000000000000, 9.184850993605147944E-16, 40.00000000000000000 ) ) ;
#15476=CARTESIAN_POINT ( 'NONE',  ( -18.00000000043041126, -3.580422610670022543, -9.973481249819688088 ) ) ;
#15480=CIRCLE ( 'NONE', #8360, 2.649999999999999467 ) ;
#15490=CARTESIAN_POINT ( 'NONE',  ( -6.929096493489625530, 2.870125743571138255, -3.749637499819689079 ) ) ;
#15498=CARTESIAN_POINT ( 'NONE',  ( 18.00000000000000000, -2.163824016901520184E-09, 11.97895000018031375 ) ) ;
#15519=CARTESIAN_POINT ( 'NONE',  ( 18.00000000000000000, -2.163824016901520184E-09, -4.966449999819686489 ) ) ;
#15531=CARTESIAN_POINT ( 'NONE',  ( 14.79893867758297610, -1.779016607511492805E-09, 6.315291918841546170 ) ) ;
#15535=EDGE_CURVE ( 'NONE', #2751, #10315, #1191, .T. ) ;
#15537=CARTESIAN_POINT ( 'NONE',  ( 12.72792205982779379, -12.72792206288790950, 13.15707500018031162 ) ) ;
#15546=CARTESIAN_POINT ( 'NONE',  ( -16.62983158603121936, -6.888301780572499311, -12.17261249981969229 ) ) ;
#15556=CARTESIAN_POINT ( 'NONE',  ( -10.19618095414378800, -15.25966316918061771, -1.726606249819691463 ) ) ;
#15560=CARTESIAN_POINT ( 'NONE',  ( 5.303300859536635770, 5.303300858261589923, -13.38942499981969014 ) ) ;
#15564=CARTESIAN_POINT ( 'NONE',  ( 1.491842754445843688, -7.500000000179346316, 18.12541875018031945 ) ) ;
#15565=CARTESIAN_POINT ( 'NONE',  ( -12.54593441764187034, -8.382925368423267187, 13.95111433151907754 ) ) ;
#15569=CARTESIAN_POINT ( 'NONE',  ( -10.19618095047498052, 15.25966317163203101, -17.63129374981969022 ) ) ;
#15573=EDGE_CURVE ( 'NONE', #197, #1438, #17721, .T. ) ;
#15587=CARTESIAN_POINT ( 'NONE',  ( 7.500000000000000888, -9.015933403756337545E-10, -27.90119999981969556 ) ) ;
#15588=AXIS2_PLACEMENT_3D ( 'NONE', #10219, #2059, #8625 ) ;
#15589=DIRECTION ( 'NONE',  ( 1.000000000000000000, 0.000000000000000000, 0.000000000000000000 ) ) ;
#15595=CARTESIAN_POINT ( 'NONE',  ( -16.62983158437510056, 6.888301784570729502, -20.41948749981968803 ) ) ;
#15607=CARTESIAN_POINT ( 'NONE',  ( -12.72792206288790950, -12.72792205982779556, -22.18667499981969726 ) ) ;
#15621=CARTESIAN_POINT ( 'NONE',  ( -10.19618095047498052, 15.25966317163203101, -17.63129374981968667 ) ) ;
#15634=CYLINDRICAL_SURFACE ( 'NONE', #20418, 7.500000000000000000 ) ;
#15636=CARTESIAN_POINT ( 'NONE',  ( -14.79893867793684059, -2.943691925285399691, 1.308260668841543461 ) ) ;
#15645=CARTESIAN_POINT ( 'NONE',  ( 18.00000000043040771, 3.580422610670018546, 11.68441875018031162 ) ) ;
#15656=CARTESIAN_POINT ( 'NONE',  ( 12.72792206288790773, 12.72792205982779912, -17.47417499981969513 ) ) ;
#15660=CARTESIAN_POINT ( 'NONE',  ( -7.500000000000009770, -1.491842754878800248, -7.793331249912205827 ) ) ;
#15665=CARTESIAN_POINT ( 'NONE',  ( -15.25966316918061949, 10.19618095414378800, 0.6296437501803093806 ) ) ;
#15666=CARTESIAN_POINT ( 'NONE',  ( -7.499999999820669672, 1.491842756249032620, -16.62926874981969050 ) ) ;
#15670=AXIS2_PLACEMENT_3D ( 'NONE', #3422, #16358, #16257 ) ;
#15671=CARTESIAN_POINT ( 'NONE',  ( -5.663308646854335215, 13.67243654778934925, 16.60189558151908074 ) ) ;
#15683=ORIENTED_EDGE ( 'NONE', *, *, #15037, .T. ) ;
#15697=CARTESIAN_POINT ( 'NONE',  ( -6.929096494179677101, -2.870125741905209527, -23.77776249981969414 ) ) ;
#15708=CARTESIAN_POINT ( 'NONE',  ( -10.19618095414378622, -15.25966316918061416, -22.48120624981968874 ) ) ;
#15723=DIRECTION ( 'NONE',  ( 0.000000000000000000, 0.000000000000000000, 1.000000000000000000 ) ) ;
#15734=CARTESIAN_POINT ( 'NONE',  ( -12.72792206288791128, -12.72792205982779912, -10.85707499981969093 ) ) ;
#15748=CARTESIAN_POINT ( 'NONE',  ( -14.79893867722910628, 2.943691928843437111, -7.527676831158455428 ) ) ;
#15753=CARTESIAN_POINT ( 'NONE',  ( -5.303300859536632217, -5.303300858261584594, -24.36682499981969841 ) ) ;
#15754=CARTESIAN_POINT ( 'NONE',  ( -12.72792206288790950, -12.72792205982779556, 15.51332500018031268 ) ) ;
#15755=CARTESIAN_POINT ( 'NONE',  ( 7.500000000000004441, -8.788009009181406898E-15, -18.47619999999769647 ) ) ;
#15766=CARTESIAN_POINT ( 'NONE',  ( 3.580422614997667896, 17.99999999956958163, -8.932768749819693710 ) ) ;
#15771=FACE_OUTER_BOUND ( 'NONE', #4058, .T. ) ;
#15774=CARTESIAN_POINT ( 'NONE',  ( -15.25966317163203456, -10.19618095047498230, -1.137543749819690087 ) ) ;
#15780=CARTESIAN_POINT ( 'NONE',  ( -2.943691925285395694, 14.79893867793683349, 7.471426831519076828 ) ) ;
#15801=CARTESIAN_POINT ( 'NONE',  ( -4.276731815070949239, -10.32494394706616347, -8.837077749352573619 ) ) ;
#15802=CARTESIAN_POINT ( 'NONE',  ( -2.870125743571140919, -6.929096493489624642, -24.95588749981968846 ) ) ;
#15813=CARTESIAN_POINT ( 'NONE',  ( 6.888301780572507305, -16.62983158603121936, -14.52886249981968625 ) ) ;
#15825=FACE_OUTER_BOUND ( 'NONE', #16632, .T. ) ;
#15826=CARTESIAN_POINT ( 'NONE',  ( 6.888301780572505528, -16.62983158603121581, -23.95386249981969229 ) ) ;
#15843=CARTESIAN_POINT ( 'NONE',  ( 6.888301784570728614, 16.62983158437510056, -6.733637499819689509 ) ) ;
#15854=EDGE_CURVE ( 'NONE', #18811, #8415, #13191, .T. ) ;
#15857=CARTESIAN_POINT ( 'NONE',  ( 14.79893867793684059, 2.943691925285398359, -3.404239331158455339 ) ) ;
#15859=CARTESIAN_POINT ( 'NONE',  ( -6.358192988180015881, -4.248408729364577141, -14.64729374981969379 ) ) ;
#15861=ORIENTED_EDGE ( 'NONE', *, *, #5075, .F. ) ;
#15871=CARTESIAN_POINT ( 'NONE',  ( -12.72792205982779556, 12.72792206288790773, -10.40542499981968838 ) ) ;
#15873=CARTESIAN_POINT ( 'NONE',  ( 1.491842754445843688, -7.500000000179346316, -10.14958124981968268 ) ) ;
#15875=FACE_OUTER_BOUND ( 'NONE', #2611, .T. ) ;
#15876=DIRECTION ( 'NONE',  ( 1.000000000000000000, 0.000000000000000000, 0.000000000000000000 ) ) ;
#15878=CARTESIAN_POINT ( 'NONE',  ( 18.00000000043041481, 3.580422610670020322, 4.164018750180309425 ) ) ;
#15879=CARTESIAN_POINT ( 'NONE',  ( 2.870125743571140475, 6.929096493489632635, -13.97848749981969085 ) ) ;
#15880=ORIENTED_EDGE ( 'NONE', *, *, #693, .F. ) ;
#15883=CARTESIAN_POINT ( 'NONE',  ( -1.343452921478823292E-09, -11.17563879731704723, -25.97385975028680605 ) ) ;
#15888=CARTESIAN_POINT ( 'NONE',  ( -17.99999999956958519, 3.580422614997674113, -18.80941874981968809 ) ) ;
#15897=CARTESIAN_POINT ( 'NONE',  ( -15.15000000000000568, 3.245314017740485469E-16, 40.00000000000000000 ) ) ;
#15902=CARTESIAN_POINT ( 'NONE',  ( -4.276731812588566939, 10.32494394809439875, -14.72770274935257362 ) ) ;
#15903=( BOUNDED_CURVE ( )  B_SPLINE_CURVE ( 2, ( #4583, #19383, #16211, #12836, #1894, #5065, #13035, #6445, #18004, #19687, #12933, #5167, #18111, #4871, #16000, #1502, #17811, #6553, #3281, #9749, #19489, #10366, #19793, #6857, #16833, #16928, #5275, #18312, #3886, #13654, #5581, #12061, #3779, #18217, #3993, #11748, #7067, #3681, #10473, #13760, #10055, #20212, #11950, #8870, #10155, #832, #2204, #10260, #16722, #16610, #8765, #18532, #8661, #15136, #15344, #5689, #2410, #2100, #404, #20103, #623, #8556, #15036, #11845, #518, #12161, #13547, #18628, #19992, #2003, #5476, #18424, #6964, #2313, #16519, #13452, #8452, #19901, #15234, #716, #14928, #7173, #7280, #5377, #13347, #7488, #6112, #10795, #5911, #13972, #1154, #20733, #20428, #18952, #14084, #4422, #9415, #17152, #2638, #14289, #7605, #13863, #12382, #15766, #6218, #1367, #18744, #6018, #15871, #17041, #19055, #9195, #14192, #12490, #15546, #1042, #2529, #5792, #7813, #18850, #12588, #9096, #4327, #12706, #20535, #20310, #4092, #9303, #8986, #17256, #15452, #2726, #15656, #7719, #10888, #17362, #943, #2835, #12268, #1267, #10578, #20635, #7386, #4215, #10692, #4531, #10994, #17471, #2947, #19161, #13115, #4740, #9720, #174, #4948, #13013, #11206, #20844, #19568, #16281, #4638 ),
 .UNSPECIFIED., .F., .T. ) 
 B_SPLINE_CURVE_WITH_KNOTS ( ( 3, 2, 2, 2, 2, 2, 2, 2, 2, 2, 2, 2, 2, 2, 2, 2, 2, 2, 2, 2, 2, 2, 2, 2, 2, 2, 2, 2, 2, 2, 2, 2, 2, 2, 2, 2, 2, 2, 2, 2, 2, 2, 2, 2, 2, 2, 2, 2, 2, 2, 2, 2, 2, 2, 2, 2, 2, 2, 2, 2, 2, 2, 2, 2, 2, 2, 2, 2, 2, 2, 2, 2, 2, 2, 2, 2, 2, 2, 2, 2, 3 ),
 ( 0.000000000000000000, 0.01250000000000000069, 0.02500000000000000139, 0.03749999999999999861, 0.05000000000000000278, 0.06250000000000000000, 0.07499999999999999722, 0.08749999999999999445, 0.1000000000000000056, 0.1125000000000000028, 0.1250000000000000000, 0.1375000000000000111, 0.1499999999999999944, 0.1625000000000000056, 0.1749999999999999889, 0.1875000000000000000, 0.2000000000000000111, 0.2124999999999999944, 0.2250000000000000056, 0.2374999999999999889, 0.2500000000000000000, 0.2625000000000000111, 0.2750000000000000222, 0.2874999999999999778, 0.2999999999999999889, 0.3125000000000000000, 0.3250000000000000111, 0.3375000000000000222, 0.3499999999999999778, 0.3624999999999999889, 0.3750000000000000000, 0.3875000000000000111, 0.4000000000000000222, 0.4124999999999999778, 0.4249999999999999889, 0.4375000000000000000, 0.4500000000000000111, 0.4625000000000000222, 0.4749999999999999778, 0.4874999999999999889, 0.5000000000000000000, 0.5124999999999999556, 0.5250000000000000222, 0.5374999999999999778, 0.5500000000000000444, 0.5625000000000000000, 0.5749999999999999556, 0.5875000000000000222, 0.5999999999999999778, 0.6125000000000000444, 0.6250000000000000000, 0.6374999999999999556, 0.6500000000000000222, 0.6624999999999999778, 0.6750000000000000444, 0.6875000000000000000, 0.6999999999999999556, 0.7125000000000000222, 0.7249999999999999778, 0.7375000000000000444, 0.7500000000000000000, 0.7624999999999999556, 0.7750000000000000222, 0.7874999999999999778, 0.8000000000000000444, 0.8125000000000000000, 0.8249999999999999556, 0.8375000000000000222, 0.8499999999999999778, 0.8625000000000000444, 0.8750000000000000000, 0.8874999999999999556, 0.9000000000000000222, 0.9124999999999999778, 0.9250000000000000444, 0.9375000000000000000, 0.9499999999999999556, 0.9625000000000000222, 0.9749999999999999778, 0.9875000000000000444, 1.000000000000000000 ),
 .UNSPECIFIED. ) 
 CURVE ( )  GEOMETRIC_REPRESENTATION_ITEM ( )  RATIONAL_B_SPLINE_CURVE ( ( 1.000000000000000000, 0.9807852804032304306, 1.000000000000000000, 0.9807852804032304306, 1.000000000000000000, 0.9807852804032304306, 1.000000000000000000, 0.9807852804032304306, 1.000000000000000000, 0.9807852804032304306, 1.000000000000000000, 0.9807852804032304306, 1.000000000000000000, 0.9807852804032304306, 1.000000000000000000, 0.9807852804032304306, 1.000000000000000000, 0.9807852804032304306, 1.000000000000000000, 0.9807852804032304306, 1.000000000000000000, 0.9807852804032304306, 1.000000000000000000, 0.9807852804032304306, 1.000000000000000000, 0.9807852804032304306, 1.000000000000000000, 0.9807852804032304306, 1.000000000000000000, 0.9807852804032304306, 1.000000000000000000, 0.9807852804032304306, 1.000000000000000000, 0.9807852804032304306, 1.000000000000000000, 0.9807852804032304306, 1.000000000000000000, 0.9807852804032304306, 1.000000000000000000, 0.9807852804032304306, 1.000000000000000000, 0.9807852804032304306, 1.000000000000000000, 0.9807852804032304306, 1.000000000000000000, 0.9807852804032304306, 1.000000000000000000, 0.9807852804032304306, 1.000000000000000000, 0.9807852804032304306, 1.000000000000000000, 0.9807852804032304306, 1.000000000000000000, 0.9807852804032304306, 1.000000000000000000, 0.9807852804032304306, 1.000000000000000000, 0.9807852804032304306, 1.000000000000000000, 0.9807852804032304306, 1.000000000000000000, 0.9807852804032304306, 1.000000000000000000, 0.9807852804032304306, 1.000000000000000000, 0.9807852804032304306, 1.000000000000000000, 0.9807852804032304306, 1.000000000000000000, 0.9807852804032304306, 1.000000000000000000, 0.9807852804032304306, 1.000000000000000000, 0.9807852804032304306, 1.000000000000000000, 0.9807852804032304306, 1.000000000000000000, 0.9807852804032304306, 1.000000000000000000, 0.9807852804032304306, 1.000000000000000000, 0.9807852804032304306, 1.000000000000000000, 0.9807852804032304306, 1.000000000000000000, 0.9807852804032304306, 1.000000000000000000, 0.9807852804032304306, 1.000000000000000000, 0.9807852804032304306, 1.000000000000000000, 0.9807852804032304306, 1.000000000000000000, 0.9807852804032304306, 1.000000000000000000, 0.9807852804032304306, 1.000000000000000000, 0.9807852804032304306, 1.000000000000000000, 0.9807852804032304306, 1.000000000000000000, 0.9807852804032304306, 1.000000000000000000, 0.9807852804032304306, 1.000000000000000000, 0.9807852804032304306, 1.000000000000000000, 0.9807852804032304306, 1.000000000000000000, 0.9807852804032304306, 1.000000000000000000, 0.9807852804032304306, 1.000000000000000000, 0.9807852804032304306, 1.000000000000000000, 0.9807852804032304306, 1.000000000000000000, 0.9807852804032304306, 1.000000000000000000, 0.9807852804032304306, 1.000000000000000000, 0.9807852804032304306, 1.000000000000000000, 0.9807852804032304306, 1.000000000000000000, 0.9807852804032304306, 1.000000000000000000, 0.9807852804032304306, 1.000000000000000000, 0.9807852804032304306, 1.000000000000000000, 0.9807852804032304306, 1.000000000000000000, 0.9807852804032304306, 1.000000000000000000, 0.9807852804032304306, 1.000000000000000000, 0.9807852804032304306, 1.000000000000000000, 0.9807852804032304306, 1.000000000000000000, 0.9807852804032304306, 1.000000000000000000, 0.9807852804032304306, 1.000000000000000000, 0.9807852804032304306, 1.000000000000000000, 0.9807852804032304306, 1.000000000000000000, 0.9807852804032304306, 1.000000000000000000, 0.9807852804032304306, 1.000000000000000000, 0.9807852804032304306, 1.000000000000000000, 0.9807852804032304306, 1.000000000000000000, 0.9807852804032304306, 1.000000000000000000, 0.9807852804032304306, 1.000000000000000000 ) ) 
 REPRESENTATION_ITEM ( '' )  );
#15904=CARTESIAN_POINT ( 'NONE',  ( 4.248408729364575365, -6.358192988180014993, -17.00354374981968775 ) ) ;
#15910=DIRECTION ( 'NONE',  ( -0.000000000000000000, -0.000000000000000000, -1.000000000000000000 ) ) ;
#15912=CARTESIAN_POINT ( 'NONE',  ( -12.72792206288791128, -12.72792205982779912, -22.18667499981969371 ) ) ;
#15930=CARTESIAN_POINT ( 'NONE',  ( 2.870125741905214412, -6.929096494179682431, -1.019112499819684770 ) ) ;
#15938=DIRECTION ( 'NONE',  ( 1.000000000000000000, 0.000000000000000000, 0.000000000000000000 ) ) ;
#15940=ADVANCED_FACE ( 'NONE', ( #2319 ), #181, .F. ) ;
#15950=CARTESIAN_POINT ( 'NONE',  ( 12.54593441562640876, -8.382925371439629458, -21.07611433115846111 ) ) ;
#15952=CARTESIAN_POINT ( 'NONE',  ( 1.491842754445842578, -7.500000000179340987, -16.41448124981969059 ) ) ;
#15959=CARTESIAN_POINT ( 'NONE',  ( -4.248408729364577141, 6.358192988180014993, -21.71604374981969343 ) ) ;
#15968=ORIENTED_EDGE ( 'NONE', *, *, #2538, .T. ) ;
#15981=CARTESIAN_POINT ( 'NONE',  ( -6.888301784570739272, -16.62983158437509701, -20.87113749981968880 ) ) ;
#15983=CARTESIAN_POINT ( 'NONE',  ( 1.491842754445843688, -7.500000000179346316, -10.14958124981968268 ) ) ;
#15986=CARTESIAN_POINT ( 'NONE',  ( 8.382925371439627682, 12.54593441562639988, 8.649551831519074696 ) ) ;
#16000=CARTESIAN_POINT ( 'NONE',  ( -16.62983158437509701, 6.888301784570728614, 17.28051250018031126 ) ) ;
#16003=VERTEX_POINT ( 'NONE', #1685 ) ;
#16007=DIRECTION ( 'NONE',  ( -1.202124453834178081E-10, -1.000000000000000000, 6.477240929643252887E-26 ) ) ;
#16012=CARTESIAN_POINT ( 'NONE',  ( -11.17563879731705789, 1.343452237168309506E-09, -16.49489024935257575 ) ) ;
#16014=CARTESIAN_POINT ( 'NONE',  ( 10.32494394809438987, 4.276731812588564274, 18.20582774971320461 ) ) ;
#16019=EDGE_LOOP ( 'NONE', ( #1311, #14004, #2353, #1284 ) ) ;
#16022=CARTESIAN_POINT ( 'NONE',  ( -17.99999999956958519, 3.580422614997674113, -11.28901874981968589 ) ) ;
#16034=EDGE_CURVE ( 'NONE', #8981, #6083, #12998, .T. ) ;
#16038=DIRECTION ( 'NONE',  ( 1.000000000000000000, 0.000000000000000000, 0.000000000000000000 ) ) ;
#16041=CARTESIAN_POINT ( 'NONE',  ( -9.015947181032828388E-10, -7.500000000000002665, 12.15505000018031012 ) ) ;
#16044=ORIENTED_EDGE ( 'NONE', *, *, #16077, .F. ) ;
#16064=CARTESIAN_POINT ( 'NONE',  ( -2.943691925285397470, 14.79893867793684059, -15.18548933115845401 ) ) ;
#16077=EDGE_CURVE ( 'NONE', #20036, #9398, #8835, .T. ) ;
#16087=ORIENTED_EDGE ( 'NONE', *, *, #1358, .F. ) ;
#16092=CARTESIAN_POINT ( 'NONE',  ( -15.25966316918061949, 10.19618095414378800, -8.795356249819690220 ) ) ;
#16099=CARTESIAN_POINT ( 'NONE',  ( -8.382925368423267187, 12.54593441764186856, -11.96763566848092530 ) ) ;
#16106=DIRECTION ( 'NONE',  ( 1.000000000000000000, 0.000000000000000000, 0.000000000000000000 ) ) ;
#16122=( NAMED_UNIT ( * ) SI_UNIT ( $, .STERADIAN. ) SOLID_ANGLE_UNIT ( ) );
#16123=CARTESIAN_POINT ( 'NONE',  ( -4.248408730893249441, -6.358192987158595599, 19.30354375018031732 ) ) ;
#16124=CARTESIAN_POINT ( 'NONE',  ( -6.330490858644137298, -9.474249097082495297, 3.184733999713198038 ) ) ;
#16132=CARTESIAN_POINT ( 'NONE',  ( -3.580422614997675002, -17.99999999956958163, 7.109331250180313866 ) ) ;
#16134=ORIENTED_EDGE ( 'NONE', *, *, #15854, .T. ) ;
#16151=CARTESIAN_POINT ( 'NONE',  ( 2.870125741905211747, -6.929096494179675325, 11.56598750018031296 ) ) ;
#16158=CARTESIAN_POINT ( 'NONE',  ( 18.00000000000000000, -2.163824016901520184E-09, -23.81644999981969235 ) ) ;
#16159=CARTESIAN_POINT ( 'NONE',  ( 12.72792206288790950, 12.72792205982780089, 20.22582500018031837 ) ) ;
#16163=FACE_BOUND ( 'NONE', #15101, .T. ) ;
#16172=CARTESIAN_POINT ( 'NONE',  ( 14.79893867722910450, -2.943691928843438443, -12.24017683115845578 ) ) ;
#16192=ORIENTED_EDGE ( 'NONE', *, *, #11853, .T. ) ;
#16196=CARTESIAN_POINT ( 'NONE',  ( -12.72792205982780089, 12.72792206288791128, -8.500824999819689864 ) ) ;
#16200=CARTESIAN_POINT ( 'NONE',  ( -10.46442989454075168, -10.46442989202483709, -14.61841691848093028 ) ) ;
#16205=CYLINDRICAL_SURFACE ( 'NONE', #11417, 2.649999999999999467 ) ;
#16209=ORIENTED_EDGE ( 'NONE', *, *, #19310, .F. ) ;
#16211=CARTESIAN_POINT ( 'NONE',  ( 16.62983158603121936, 6.888301780572501976, 20.81488750018031197 ) ) ;
#16219=CIRCLE ( 'NONE', #5369, 16.99999999999995026 ) ;
#16223=CARTESIAN_POINT ( 'NONE',  ( -5.303300859536636658, -5.303300858261589035, 10.17307500018031519 ) ) ;
#16224=CARTESIAN_POINT ( 'NONE',  ( 2.222972771497739419, 11.17563879704981922, -2.116828500286803028 ) ) ;
#16230=CARTESIAN_POINT ( 'NONE',  ( -18.00000000043041126, -3.580422610670022543, 8.876518750180315109 ) ) ;
#16247=CARTESIAN_POINT ( 'NONE',  ( 1.491842756249028845, 7.499999999820661678, 7.737081250180311898 ) ) ;
#16255=CARTESIAN_POINT ( 'NONE',  ( 0.000000000000000000, 0.000000000000000000, -40.00000000000000000 ) ) ;
#16257=DIRECTION ( 'NONE',  ( 1.000000000000000000, 0.000000000000000000, 0.000000000000000000 ) ) ;
#16266=CARTESIAN_POINT ( 'NONE',  ( -2.222972768810837607, 11.17563879758428769, 23.26682850064743491 ) ) ;
#16267=ORIENTED_EDGE ( 'NONE', *, *, #17932, .T. ) ;
#16273=DIRECTION ( 'NONE',  ( -0.000000000000000000, -0.000000000000000000, 1.000000000000000000 ) ) ;
#16281=CARTESIAN_POINT ( 'NONE',  ( 17.99999999956957808, -3.580422614997675446, -25.42651874981969584 ) ) ;
#16283=CARTESIAN_POINT ( 'NONE',  ( 6.358192987158596488, -4.248408730893249441, -11.32770624981968588 ) ) ;
#16287=CARTESIAN_POINT ( 'NONE',  ( 3.580422614997669228, 17.99999999956958874, -16.45316874981969590 ) ) ;
#16289=ORIENTED_EDGE ( 'NONE', *, *, #16077, .T. ) ;
#16290=CARTESIAN_POINT ( 'NONE',  ( -6.358192987158592047, 4.248408730893246776, 5.969893750180308878 ) ) ;
#16293=CARTESIAN_POINT ( 'NONE',  ( -2.943691928843435779, -14.79893867722909917, -6.077010668480928857 ) ) ;
#16314=CARTESIAN_POINT ( 'NONE',  ( 7.499999999820668783, -1.491842756249033508, 16.35823125018031376 ) ) ;
#16318=CARTESIAN_POINT ( 'NONE',  ( -11.17563879731704723, 1.343452237168308679E-09, -4.767609750286803560 ) ) ;
#16326=CARTESIAN_POINT ( 'NONE',  ( 18.00000000000000000, -2.163824016901520184E-09, 23.30855000018031475 ) ) ;
#16336=FACE_OUTER_BOUND ( 'NONE', #5790, .T. ) ;
#16345=CARTESIAN_POINT ( 'NONE',  ( -6.358192988180014993, -4.248408729364575365, 13.62770625018031367 ) ) ;
#16348=AXIS2_PLACEMENT_3D ( 'NONE', #18269, #15094, #7448 ) ;
#16355=CARTESIAN_POINT ( 'NONE',  ( 12.72792205982779734, -12.72792206288791128, 13.15707500018031517 ) ) ;
#16358=DIRECTION ( 'NONE',  ( -0.000000000000000000, -0.000000000000000000, 1.000000000000000000 ) ) ;
#16368=CARTESIAN_POINT ( 'NONE',  ( -13.67243654642775574, 5.663308650141533285, -16.65814558115846111 ) ) ;
#16375=CARTESIAN_POINT ( 'NONE',  ( 5.303300858261583706, -5.303300859536632217, -26.72307499981969414 ) ) ;
#16389=CARTESIAN_POINT ( 'NONE',  ( 7.500000000000009770, -8.788009009181406898E-15, -12.21129999999768501 ) ) ;
#16391=CARTESIAN_POINT ( 'NONE',  ( 6.888301784570730391, 16.62983158437510411, -6.733637499819693062 ) ) ;
#16396=CARTESIAN_POINT ( 'NONE',  ( -5.663308650141535949, -13.67243654642774686, 3.642520581519076650 ) ) ;
#16407=ORIENTED_EDGE ( 'NONE', *, *, #10651, .T. ) ;
#16418=CARTESIAN_POINT ( 'NONE',  ( 6.929096494179683319, 2.870125741905213079, 24.89963750018031519 ) ) ;
#16420=CARTESIAN_POINT ( 'NONE',  ( -9.474249098604506258, -6.330490856366290053, -5.651203500286803738 ) ) ;
#16421=FACE_OUTER_BOUND ( 'NONE', #13233, .T. ) ;
#16426=CARTESIAN_POINT ( 'NONE',  ( -3.580422610670018546, 18.00000000043041126, 20.65776875018031333 ) ) ;
#16446=CARTESIAN_POINT ( 'NONE',  ( -2.870125741905209971, 6.929096494179676213, 16.27848750018031154 ) ) ;
#16470=CARTESIAN_POINT ( 'NONE',  ( 5.303300859536631329, 5.303300858261585482, -10.22932499981969379 ) ) ;
#16473=MECHANICAL_DESIGN_GEOMETRIC_PRESENTATION_REPRESENTATION('',(#1642),#10046);
#16477=CARTESIAN_POINT ( 'NONE',  ( -4.276731815070949239, -10.32494394706616347, 10.01292225064742958 ) ) ;
#16482=VERTEX_POINT ( 'NONE', #8113 ) ;
#16486=CARTESIAN_POINT ( 'NONE',  ( 10.19618095414378800, 15.25966316918061416, 21.83589375018031475 ) ) ;
#16496=CARTESIAN_POINT ( 'NONE',  ( 6.358192987158596488, -4.248408730893249441, -20.75270624981968837 ) ) ;
#16505=CARTESIAN_POINT ( 'NONE',  ( -14.79893867722910628, 2.943691928843437111, 11.32232316884154777 ) ) ;
#16509=ORIENTED_EDGE ( 'NONE', *, *, #15116, .T. ) ;
#16510=CARTESIAN_POINT ( 'NONE',  ( 12.54593441764186679, 8.382925368423272516, -19.03638566848093205 ) ) ;
#16516=CARTESIAN_POINT ( 'NONE',  ( -9.015947181032835626E-10, -7.500000000000007994, 8.994950000180315541 ) ) ;
#16519=CARTESIAN_POINT ( 'NONE',  ( -6.888301780572500199, 16.62983158603121936, -0.3913624998196918447 ) ) ;
#16528=CARTESIAN_POINT ( 'NONE',  ( 1.491842754445843688, -7.500000000179346316, 18.12541875018031945 ) ) ;
#16529=CARTESIAN_POINT ( 'NONE',  ( 6.330490856366289165, -9.474249098604506258, 10.84254649971319751 ) ) ;
#16534=CARTESIAN_POINT ( 'NONE',  ( -2.163827323447878234E-09, -18.00000000000000000, 16.23980000018031333 ) ) ;
#16543=CARTESIAN_POINT ( 'NONE',  ( 0.000000000000000000, 0.000000000000000000, 40.00000000000000000 ) ) ;
#16548=CARTESIAN_POINT ( 'NONE',  ( -4.248408729364575365, 6.358192988180014105, 15.98395625018031474 ) ) ;
#16554=ORIENTED_EDGE ( 'NONE', *, *, #1398, .F. ) ;
#16565=CARTESIAN_POINT ( 'NONE',  ( 1.491842756249029289, 7.499999999820664343, -11.11291874981969485 ) ) ;
#16567=LINE ( 'NONE', #11394, #18394 ) ;
#16568=CARTESIAN_POINT ( 'NONE',  ( -9.474249097082500626, 6.330490858644140850, 12.66370350064742922 ) ) ;
#16575=VERTEX_POINT ( 'NONE', #5127 ) ;
#16577=CARTESIAN_POINT ( 'NONE',  ( -15.25966317163203279, -10.19618095047498052, -1.137543749819686756 ) ) ;
#16579=DIRECTION ( 'NONE',  ( -0.000000000000000000, -0.000000000000000000, 1.000000000000000000 ) ) ;
#16582=ADVANCED_FACE ( 'NONE', ( #1455, #7908, #14387, #20829, #8828 ), #7129, .F. ) ;
#16584=CARTESIAN_POINT ( 'NONE',  ( 6.250000000000054179, 10.82531754730546147, -43.00000000000000000 ) ) ;
#16590=CARTESIAN_POINT ( 'NONE',  ( -14.79893867793684059, -2.943691925285399691, 20.15826066884155310 ) ) ;
#16597=CARTESIAN_POINT ( 'NONE',  ( -14.79893867758296544, 1.779018419858780125E-09, -22.86529191848093490 ) ) ;
#16605=CARTESIAN_POINT ( 'NONE',  ( 2.870125743571138255, 6.929096493489627306, 17.45661250018030941 ) ) ;
#16610=CARTESIAN_POINT ( 'NONE',  ( -18.00000000043040771, -3.580422610670021211, 6.971918750180310376 ) ) ;
#16624=CARTESIAN_POINT ( 'NONE',  ( -4.248408729364580694, 6.358192988180020322, 3.398856250180315897 ) ) ;
#16626=CARTESIAN_POINT ( 'NONE',  ( 7.902369978624323110, 7.902369976724394895, -20.08323475028680605 ) ) ;
#16632=EDGE_LOOP ( 'NONE', ( #17087, #9143, #18363, #8353 ) ) ;
#16634=CARTESIAN_POINT ( 'NONE',  ( -6.888301780572501976, 16.62983158603122291, -7.911762499819688266 ) ) ;
#16647=PRESENTATION_STYLE_ASSIGNMENT (( #334 ) ) ;
#16653=CARTESIAN_POINT ( 'NONE',  ( -6.929096493489625530, 2.870125743571138255, -13.17463749981968846 ) ) ;
#16660=CARTESIAN_POINT ( 'NONE',  ( 16.62983158603122291, 6.888301780572502864, 1.964887500180312330 ) ) ;
#16674=CARTESIAN_POINT ( 'NONE',  ( -4.248408729364577141, 6.358192988180014993, -12.29104374981969094 ) ) ;
#16675=CARTESIAN_POINT ( 'NONE',  ( 12.72792206288790773, 12.72792205982779912, -8.049174999819690868 ) ) ;
#16678=CARTESIAN_POINT ( 'NONE',  ( 6.330490856366294494, -9.474249098604513364, 17.96526600064742851 ) ) ;
#16686=CARTESIAN_POINT ( 'NONE',  ( -18.00000000000000000, 2.163826221265758884E-09, 9.171050000180313688 ) ) ;
#16698=ADVANCED_FACE ( 'NONE', ( #13611 ), #3955, .F. ) ;
#16701=CARTESIAN_POINT ( 'NONE',  ( 1.779017513685136568E-09, 14.79893867758297610, 13.38404191884154670 ) ) ;
#16711=CARTESIAN_POINT ( 'NONE',  ( -13.67243654642775041, 5.663308650141531508, -22.27622941848092708 ) ) ;
#16719=CARTESIAN_POINT ( 'NONE',  ( 1.491842754445843688, -7.500000000179346316, 8.700418750180315186 ) ) ;
#16722=CARTESIAN_POINT ( 'NONE',  ( -17.99999999999999645, 2.163826221265758470E-09, 7.266450000180311619 ) ) ;
#16733=CARTESIAN_POINT ( 'NONE',  ( -1.491842754445842800, 7.500000000179346316, -14.86208124981968481 ) ) ;
#16736=CARTESIAN_POINT ( 'NONE',  ( -1.491842756249033064, -7.499999999820668783, -9.560518749819690854 ) ) ;
#16737=CARTESIAN_POINT ( 'NONE',  ( -2.222972768810836275, 11.17563879758427525, -21.55589100028680249 ) ) ;
#16743=CARTESIAN_POINT ( 'NONE',  ( 18.00000000000000000, -2.163824016901520184E-09, -4.966449999819686489 ) ) ;
#16745=EDGE_CURVE ( 'NONE', #13598, #1332, #7463, .T. ) ;
#16760=CARTESIAN_POINT ( 'NONE',  ( 6.358192987158590270, -4.248408730893245000, -8.167606249819691300 ) ) ;
#16766=CARTESIAN_POINT ( 'NONE',  ( 6.929096494179683319, 2.870125741905213079, 6.049637500180313765 ) ) ;
#16769=CARTESIAN_POINT ( 'NONE',  ( 18.00000000043041126, 3.580422610670019434, 11.68441875018031517 ) ) ;
#16779=LINE ( 'NONE', #2267, #605 ) ;
#16780=CARTESIAN_POINT ( 'NONE',  ( -15.25966317163202923, -10.19618095047497874, -3.042143749819689713 ) ) ;
#16784=CARTESIAN_POINT ( 'NONE',  ( -4.276731812588566939, 10.32494394809439875, 13.54729725064743384 ) ) ;
#16789=EDGE_CURVE ( 'NONE', #20492, #1625, #12550, .T. ) ;
#16792=LINE ( 'NONE', #18703, #14882 ) ;
#16794=CARTESIAN_POINT ( 'NONE',  ( -18.00000000043041126, -3.580422610670022099, -0.5484812498196891539 ) ) ;
#16809=FACE_OUTER_BOUND ( 'NONE', #2060, .T. ) ;
#16813=CARTESIAN_POINT ( 'NONE',  ( -10.46442989454075878, -10.46442989202484242, 9.849666918841547769 ) ) ;
#16817=AXIS2_PLACEMENT_3D ( 'NONE', #19262, #4742, #9920 ) ;
#16822=CARTESIAN_POINT ( 'NONE',  ( 14.79893867758296544, -1.779016607511491977E-09, -27.57779191848093703 ) ) ;
#16833=CARTESIAN_POINT ( 'NONE',  ( -2.163827323447877821E-09, -17.99999999999999645, 14.33520000018031126 ) ) ;
#16844=CARTESIAN_POINT ( 'NONE',  ( -6.929096493489632635, 2.870125743571140919, 2.515262500180314387 ) ) ;
#16846=CARTESIAN_POINT ( 'NONE',  ( -9.474249097082497073, 6.330490858644137298, -22.73401600028680747 ) ) ;
#16855=CARTESIAN_POINT ( 'NONE',  ( -3.580422610670018546, 18.00000000043041126, 1.807768750180311468 ) ) ;
#16862=ORIENTED_EDGE ( 'NONE', *, *, #7519, .T. ) ;
#16868=CARTESIAN_POINT ( 'NONE',  ( -12.50000000000000533, 0.000000000000000000, -43.00000000000000000 ) ) ;
#16870=CARTESIAN_POINT ( 'NONE',  ( 2.870125741905211747, -6.929096494179675325, -7.284012499819688458 ) ) ;
#16873=CARTESIAN_POINT ( 'NONE',  ( 6.250000000000054179, 10.82531754730546147, -40.00000000000000000 ) ) ;
#16877=CARTESIAN_POINT ( 'NONE',  ( 9.015937996181842420E-10, 7.500000000000007994, 4.282450000180314298 ) ) ;
#16879=EDGE_LOOP ( 'NONE', ( #4012, #15236, #18034, #9651 ) ) ;
#16880=CARTESIAN_POINT ( 'NONE',  ( 3.580422610670020322, -18.00000000043041126, 4.615668750180313751 ) ) ;
#16891=CARTESIAN_POINT ( 'NONE',  ( -3.580422614997674557, -17.99999999956957808, -13.64526874981969584 ) ) ;
#16893=CARTESIAN_POINT ( 'NONE',  ( -7.500000000000002665, -1.491842754878804023, 14.21676875008778751 ) ) ;
#16894=CARTESIAN_POINT ( 'NONE',  ( -7.902369978624331104, -7.902369976724401113, -17.67301524935258072 ) ) ;
#16903=CARTESIAN_POINT ( 'NONE',  ( -17.99999999956958519, 3.580422614997674113, 9.465581250180312267 ) ) ;
#16906=ORIENTED_EDGE ( 'NONE', *, *, #3954, .T. ) ;
#16909=CARTESIAN_POINT ( 'NONE',  ( -4.248408729364580694, 6.358192988180020322, 12.82385625018031483 ) ) ;
#16910=VERTEX_POINT ( 'NONE', #19317 ) ;
#16915=CARTESIAN_POINT ( 'NONE',  ( 2.943691928843431782, 14.79893867722910628, 23.10357316884154599 ) ) ;
#16916=ORIENTED_EDGE ( 'NONE', *, *, #18566, .T. ) ;
#16919=CARTESIAN_POINT ( 'NONE',  ( -16.62983158603121936, -6.888301780572499311, 16.10238750018030984 ) ) ;
#16928=CARTESIAN_POINT ( 'NONE',  ( 3.580422610670019878, -18.00000000043040771, 14.04066875018031091 ) ) ;
#16937=CARTESIAN_POINT ( 'NONE',  ( 7.500000000000009770, 1.491842754878799138, -12.50583124991220707 ) ) ;
#16939=CARTESIAN_POINT ( 'NONE',  ( -1.491842754445842800, 7.500000000179346316, -5.437081249819685880 ) ) ;
#16942=CARTESIAN_POINT ( 'NONE',  ( 6.330490856366289165, -9.474249098604506258, -8.007453500286802139 ) ) ;
#16946=DIRECTION ( 'NONE',  ( -0.000000000000000000, -0.000000000000000000, -1.000000000000000000 ) ) ;
#16947=CARTESIAN_POINT ( 'NONE',  ( 16.62983158437509346, -6.888301784570739272, -4.377387499819689332 ) ) ;
#16960=EDGE_CURVE ( 'NONE', #18276, #7721, #865, .T. ) ;
#16962=DIRECTION ( 'NONE',  ( 1.000000000000000000, 0.000000000000000000, 0.000000000000000000 ) ) ;
#16965=CARTESIAN_POINT ( 'NONE',  ( -1.491842756249031510, -7.499999999820660790, -6.400418749819690056 ) ) ;
#16973=CARTESIAN_POINT ( 'NONE',  ( 10.19618095414378800, 15.25966316918061416, 1.081293750180314372 ) ) ;
#16989=CARTESIAN_POINT ( 'NONE',  ( -16.62983158437509701, 6.888301784570728614, -10.99448749981968909 ) ) ;
#16994=CARTESIAN_POINT ( 'NONE',  ( -7.902369978624331104, -7.902369976724401113, -8.248015249352576461 ) ) ;
#17001=AXIS2_PLACEMENT_3D ( 'NONE', #3304, #15910, #4579 ) ;
#17003=CARTESIAN_POINT ( 'NONE',  ( -18.00000000043041126, -3.580422610670022099, 8.876518750180313333 ) ) ;
#17006=CARTESIAN_POINT ( 'NONE',  ( 4.924999999999924327, -8.530350227276771946, -43.00000000000000000 ) ) ;
#17023=CARTESIAN_POINT ( 'NONE',  ( -12.54593441764187745, -8.382925368423274293, -8.705801831158458626 ) ) ;
#17030=CARTESIAN_POINT ( 'NONE',  ( -12.72792205982779556, 12.72792206288790773, 8.444575000180309488 ) ) ;
#17036=CARTESIAN_POINT ( 'NONE',  ( 7.500000000000000000, 9.184850993605147944E-16, 40.00000000000000000 ) ) ;
#17040=CARTESIAN_POINT ( 'NONE',  ( 2.870125741905212635, -6.929096494179677101, 2.140987500180307368 ) ) ;
#17041=CARTESIAN_POINT ( 'NONE',  ( -15.25966316918061416, 10.19618095414378445, -10.69995624981968874 ) ) ;
#17050=CARTESIAN_POINT ( 'NONE',  ( -18.00000000000000355, 2.163826221265759298E-09, 9.171050000180310136 ) ) ;
#17054=CARTESIAN_POINT ( 'NONE',  ( -7.500000000000007994, 9.015942588607339023E-10, -7.498799999819685702 ) ) ;
#17057=CARTESIAN_POINT ( 'NONE',  ( 11.17563879731704723, -1.343450868547281106E-09, -9.480109750286803916 ) ) ;
#17059=AXIS2_PLACEMENT_3D ( 'NONE', #7555, #15723, #16038 ) ;
#17063=DIRECTION ( 'NONE',  ( -1.000000000000000000, 0.000000000000000000, 0.000000000000000000 ) ) ;
#17064=CARTESIAN_POINT ( 'NONE',  ( -3.580422610670018546, 18.00000000043041126, -7.617231249819687022 ) ) ;
#17070=CIRCLE ( 'NONE', #15025, 17.50000000000000355 ) ;
#17078=CARTESIAN_POINT ( 'NONE',  ( 17.99999999999999645, -2.163824016901520184E-09, 21.40395000018031268 ) ) ;
#17079=CYLINDRICAL_SURFACE ( 'NONE', #5211, 2.649999999999999467 ) ;
#17081=CARTESIAN_POINT ( 'NONE',  ( 6.929096493489624642, -2.870125743571141363, -8.462137499819689879 ) ) ;
#17087=ORIENTED_EDGE ( 'NONE', *, *, #12868, .F. ) ;
#17090=CARTESIAN_POINT ( 'NONE',  ( 6.888301784570728614, 16.62983158437510056, 10.21176250018031517 ) ) ;
#17103=CARTESIAN_POINT ( 'NONE',  ( -15.25966317163202923, -10.19618095047497874, -12.46714374981969264 ) ) ;
#17107=CARTESIAN_POINT ( 'NONE',  ( 10.32494394809439875, 4.276731812588567827, -12.37145274935257255 ) ) ;
#17110=CARTESIAN_POINT ( 'NONE',  ( 3.600000000000054712, 10.82531754730546147, 43.00000000000000000 ) ) ;
#17116=CARTESIAN_POINT ( 'NONE',  ( 16.62983158603122291, 6.888301780572502864, -14.98051249981969058 ) ) ;
#17133=CARTESIAN_POINT ( 'NONE',  ( -14.79893867793684059, -2.943691925285399691, -8.116739331158456139 ) ) ;
#17137=ADVANCED_FACE ( 'NONE', ( #18988 ), #10507, .F. ) ;
#17140=CARTESIAN_POINT ( 'NONE',  ( 18.00000000043040771, 3.580422610670018546, 2.259418750180309576 ) ) ;
#17150=CARTESIAN_POINT ( 'NONE',  ( -7.500000000000002665, -1.491842754878805355, 4.791768750087786799 ) ) ;
#17152=CARTESIAN_POINT ( 'NONE',  ( 18.00000000043040771, 3.580422610670018546, -7.165581249819689802 ) ) ;
#17163=CARTESIAN_POINT ( 'NONE',  ( -2.163827323447878648E-09, -18.00000000000000355, 6.814800000180309958 ) ) ;
#17166=CARTESIAN_POINT ( 'NONE',  ( -4.248408730893249441, -6.358192987158595599, -18.39645624981969263 ) ) ;
#17170=CARTESIAN_POINT ( 'NONE',  ( 2.222972768810837163, -11.17563879758427525, -26.26839100028680107 ) ) ;
#17176=CARTESIAN_POINT ( 'NONE',  ( -17.50000000000000355, 0.000000000000000000, -40.00000000000000000 ) ) ;
#17183=DIRECTION ( 'NONE',  ( 0.000000000000000000, 0.000000000000000000, 1.000000000000000000 ) ) ;
#17185=AXIS2_PLACEMENT_3D ( 'NONE', #8372, #3082, #4004 ) ;
#17196=CARTESIAN_POINT ( 'NONE',  ( 1.491842756249028845, 7.499999999820661678, -20.53791874981969556 ) ) ;
#17203=CARTESIAN_POINT ( 'NONE',  ( -3.580422610670018546, 18.00000000043041126, -18.94683124981968803 ) ) ;
#17208=DIRECTION ( 'NONE',  ( -1.000000000000000000, 0.000000000000000000, 0.000000000000000000 ) ) ;
#17211=ORIENTED_EDGE ( 'NONE', *, *, #504, .F. ) ;
#17212=CARTESIAN_POINT ( 'NONE',  ( 5.303300858261588147, -5.303300859536636658, -20.45817499981968624 ) ) ;
#17215=CARTESIAN_POINT ( 'NONE',  ( 3.580422610670019878, -18.00000000043040771, -23.65933124981969016 ) ) ;
#17217=CARTESIAN_POINT ( 'NONE',  ( 6.358192987158592047, -4.248408730893246776, 10.68239375018030834 ) ) ;
#17223=CIRCLE ( 'NONE', #19909, 17.50000000000000355 ) ;
#17227=CARTESIAN_POINT ( 'NONE',  ( 2.163825119083639534E-09, 18.00000000000000000, -7.322699999819687555 ) ) ;
#17233=CARTESIAN_POINT ( 'NONE',  ( 2.870125743571140475, 6.929096493489632635, 14.29651250018031661 ) ) ;
#17238=CARTESIAN_POINT ( 'NONE',  ( 5.663308650141532397, 13.67243654642775574, 4.548104418841546703 ) ) ;
#17243=VERTEX_POINT ( 'NONE', #13806 ) ;
#17245=CARTESIAN_POINT ( 'NONE',  ( 15.25966317163202568, 10.19618095047498230, 1.670356250180308422 ) ) ;
#17256=CARTESIAN_POINT ( 'NONE',  ( 18.00000000043040771, 3.580422610670018546, -16.59058124981969229 ) ) ;
#17261=DIRECTION ( 'NONE',  ( -0.000000000000000000, -0.000000000000000000, -1.000000000000000000 ) ) ;
#17264=CARTESIAN_POINT ( 'NONE',  ( 15.25966317163203101, 10.19618095047498585, 12.99995625018031120 ) ) ;
#17269=CARTESIAN_POINT ( 'NONE',  ( -4.248408729364580694, 6.358192988180020322, -15.45114374981968730 ) ) ;
#17272=CARTESIAN_POINT ( 'NONE',  ( -14.79893867793683349, -2.943691925285398359, 5.115176831519075762 ) ) ;
#17277=CARTESIAN_POINT ( 'NONE',  ( 17.99999999956958163, -3.580422614997676334, -23.52191874981969377 ) ) ;
#17280=CARTESIAN_POINT ( 'NONE',  ( -15.15000000000000568, -3.245314017740485469E-16, -43.00000000000000000 ) ) ;
#17290=DIRECTION ( 'NONE',  ( -0.000000000000000000, -0.000000000000000000, -1.000000000000000000 ) ) ;
#17292=CARTESIAN_POINT ( 'NONE',  ( 7.574999999999881162, -13.12028486733431976, -40.00000000000000000 ) ) ;
#17293=CARTESIAN_POINT ( 'NONE',  ( 2.870125741905211747, -6.929096494179675325, -16.70901249981968917 ) ) ;
#17295=DIRECTION ( 'NONE',  ( 1.000000000000000000, 0.000000000000000000, 0.000000000000000000 ) ) ;
#17296=CARTESIAN_POINT ( 'NONE',  ( 0.000000000000000000, 0.000000000000000000, 40.00000000000000000 ) ) ;
#17302=CARTESIAN_POINT ( 'NONE',  ( 3.580422610670020322, -18.00000000043041126, -14.23433124981968412 ) ) ;
#17308=CARTESIAN_POINT ( 'NONE',  ( 2.870125741905212635, -6.929096494179677101, -7.284012499819692010 ) ) ;
#17328=CARTESIAN_POINT ( 'NONE',  ( -12.72792206288791128, -12.72792205982779912, -20.28207499981969164 ) ) ;
#17329=CYLINDRICAL_SURFACE ( 'NONE', #14451, 2.649999999999999467 ) ;
#17342=CARTESIAN_POINT ( 'NONE',  ( -12.54593441562641054, 8.382925371439629458, 2.486385668841545993 ) ) ;
#17349=CARTESIAN_POINT ( 'NONE',  ( -7.500000000000004441, 9.706494107352906755E-15, -23.18869999999769860 ) ) ;
#17350=CARTESIAN_POINT ( 'NONE',  ( 3.580422610670019878, -18.00000000043040771, 14.04066875018031091 ) ) ;
#17358=EDGE_CURVE ( 'NONE', #13364, #16482, #2763, .T. ) ;
#17360=AXIS2_PLACEMENT_3D ( 'NONE', #4503, #7785, #9168 ) ;
#17362=CARTESIAN_POINT ( 'NONE',  ( 3.580422614997667896, 17.99999999956958163, -18.35776874981969442 ) ) ;
#17372=CARTESIAN_POINT ( 'NONE',  ( -6.888301784570739272, -16.62983158437509701, 7.403862500180310668 ) ) ;
#17374=CARTESIAN_POINT ( 'NONE',  ( -1.491842754445842800, 7.500000000179346316, -14.86208124981968481 ) ) ;
#17379=CARTESIAN_POINT ( 'NONE',  ( 12.54593441562639988, -8.382925371439625906, 11.00580183151907754 ) ) ;
#17402=( BOUNDED_CURVE ( )  B_SPLINE_CURVE ( 2, ( #2838, #15660, #12590, #1157, #7608, #4534, #10996, #17473, #2950, #15873, #3556, #11208, #20846, #16283, #8332, #177, #16389 ),
 .UNSPECIFIED., .F., .T. ) 
 B_SPLINE_CURVE_WITH_KNOTS ( ( 3, 2, 2, 2, 2, 2, 2, 2, 3 ),
 ( 0.7000000000038510972, 0.7125000000038511638, 0.7250000000038511194, 0.7375000000038511860, 0.7500000000038511416, 0.7625000000038510972, 0.7750000000038511638, 0.7875000000038511194, 0.8000000000038511860 ),
 .UNSPECIFIED. ) 
 CURVE ( )  GEOMETRIC_REPRESENTATION_ITEM ( )  RATIONAL_B_SPLINE_CURVE ( ( 0.9999999999940800688, 0.9807852804091503618, 1.000000000000000000, 0.9807852804032304306, 1.000000000000000000, 0.9807852804032304306, 1.000000000000000000, 0.9807852804032304306, 1.000000000000000000, 0.9807852804032304306, 1.000000000000000000, 0.9807852804032304306, 1.000000000000000000, 0.9807852804032304306, 1.000000000000000000, 0.9807852803973104994, 1.000000000005919931 ) ) 
 REPRESENTATION_ITEM ( '' )  );
#17405=CARTESIAN_POINT ( 'NONE',  ( -11.17563879731704723, 1.343452237168308679E-09, 14.08239024971319964 ) ) ;
#17409=DIRECTION ( 'NONE',  ( -0.000000000000000000, -0.000000000000000000, -1.000000000000000000 ) ) ;
#17416=CARTESIAN_POINT ( 'NONE',  ( 18.00000000000000000, -2.163824016901520184E-09, -16.29604999981969016 ) ) ;
#17426=ORIENTED_EDGE ( 'NONE', *, *, #5834, .T. ) ;
#17429=CARTESIAN_POINT ( 'NONE',  ( -18.00000000043040771, -3.580422610670021211, -21.30308124981969442 ) ) ;
#17434=LINE ( 'NONE', #11164, #12380 ) ;
#17440=CARTESIAN_POINT ( 'NONE',  ( -16.62983158603122291, -6.888301780572501087, -10.26801249981968844 ) ) ;
#17454=CARTESIAN_POINT ( 'NONE',  ( -1.779019326032424922E-09, -14.79893867758297610, -0.7534580811584571380 ) ) ;
#17456=VECTOR ( 'NONE', #5974, 1000.000000000000000 ) ;
#17461=CARTESIAN_POINT ( 'NONE',  ( -1.491842754445841690, 7.500000000179340987, -21.12698124981969272 ) ) ;
#17470=CARTESIAN_POINT ( 'NONE',  ( -4.248408730893246776, -6.358192987158592047, 3.613643750180308256 ) ) ;
#17471=CARTESIAN_POINT ( 'NONE',  ( -15.25966317163202923, -10.19618095047497874, -21.89214374981969513 ) ) ;
#17473=CARTESIAN_POINT ( 'NONE',  ( -1.491842756249033286, -7.499999999820668783, -9.560518749819689077 ) ) ;
#17477=CARTESIAN_POINT ( 'NONE',  ( 7.500000000000001776, -9.015933403756337545E-10, -24.76874999981969694 ) ) ;
#17479=CARTESIAN_POINT ( 'NONE',  ( 2.163825119083639947E-09, 18.00000000000000355, 2.102300000180308714 ) ) ;
#17480=CARTESIAN_POINT ( 'NONE',  ( 7.500000000000007994, -9.015933403756345817E-10, -12.21129999981968695 ) ) ;
#17486=CARTESIAN_POINT ( 'NONE',  ( -8.382925368423267187, 12.54593441764186856, 6.882364331519074341 ) ) ;
#17491=CARTESIAN_POINT ( 'NONE',  ( 18.00000000000000000, -2.163824016901520184E-09, -23.81644999981969235 ) ) ;
#17504=AXIS2_PLACEMENT_3D ( 'NONE', #19765, #16579, #19455 ) ;
#17507=CIRCLE ( 'NONE', #12079, 2.649999999999998579 ) ;
#17509=CARTESIAN_POINT ( 'NONE',  ( 2.222972771497741640, 11.17563879704982988, -13.84410899935257788 ) ) ;
#17511=CARTESIAN_POINT ( 'NONE',  ( 1.343451552857795099E-09, 11.17563879731704723, 16.43864024971319893 ) ) ;
#17514=DIRECTION ( 'NONE',  ( -0.000000000000000000, -0.000000000000000000, 1.000000000000000000 ) ) ;
#17522=CARTESIAN_POINT ( 'NONE',  ( -12.72792205982779912, 12.72792206288790950, -19.83042499981968732 ) ) ;
#17535=CARTESIAN_POINT ( 'NONE',  ( 16.62983158437509346, -6.888301784570737496, -25.13198749981969371 ) ) ;
#17539=CARTESIAN_POINT ( 'NONE',  ( 4.248408729364576253, -6.358192988180015881, 11.27145625018030906 ) ) ;
#17545=CARTESIAN_POINT ( 'NONE',  ( -9.015947181032835626E-10, -7.500000000000007994, -0.4300499998196871676 ) ) ;
#17546=APPLICATION_CONTEXT ( 'automotive_design' ) ;
#17553=CARTESIAN_POINT ( 'NONE',  ( -15.25966317163203279, -10.19618095047498052, -10.56254374981968880 ) ) ;
#17563=CARTESIAN_POINT ( 'NONE',  ( 0.000000000000000000, 0.000000000000000000, 40.00000000000000000 ) ) ;
#17564=CARTESIAN_POINT ( 'NONE',  ( 2.943691925285398803, -14.79893867793684059, -19.89798933115845969 ) ) ;
#17566=CARTESIAN_POINT ( 'NONE',  ( 7.500000000000000000, -1.491842755816076060, -18.18166874991221249 ) ) ;
#17570=CARTESIAN_POINT ( 'NONE',  ( 6.358192988180014993, 4.248408729364578917, -19.35979374981969769 ) ) ;
#17577=ORIENTED_EDGE ( 'NONE', *, *, #16034, .F. ) ;
#17580=FACE_OUTER_BOUND ( 'NONE', #16879, .T. ) ;
#17581=EDGE_LOOP ( 'NONE', ( #11231, #9775, #16916, #69 ) ) ;
#17586=CARTESIAN_POINT ( 'NONE',  ( -3.580422610670018990, 18.00000000043041481, -17.04223124981969306 ) ) ;
#17590=CARTESIAN_POINT ( 'NONE',  ( 10.46442989454075168, 10.46442989202483886, 18.36908308151907576 ) ) ;
#17608=CARTESIAN_POINT ( 'NONE',  ( 4.276731812588570492, -10.32494394809439697, -10.01520274935256971 ) ) ;
#17609=CARTESIAN_POINT ( 'NONE',  ( -11.17563879704981922, 2.222972771497742972, 14.37692149971319999 ) ) ;
#17616=CARTESIAN_POINT ( 'NONE',  ( -18.00000000043041126, -3.580422610670022543, -21.30308124981969087 ) ) ;
#17618=ORIENTED_EDGE ( 'NONE', *, *, #6690, .T. ) ;
#17619=DIRECTION ( 'NONE',  ( -0.000000000000000000, -0.000000000000000000, 1.000000000000000000 ) ) ;
#17628=DIRECTION ( 'NONE',  ( -0.000000000000000000, -0.000000000000000000, 1.000000000000000000 ) ) ;
#17633=EDGE_CURVE ( 'NONE', #9351, #12808, #5807, .T. ) ;
#17634=VERTEX_POINT ( 'NONE', #8755 ) ;
#17638=AXIS2_PLACEMENT_3D ( 'NONE', #4267, #7656, #17208 ) ;
#17659=CARTESIAN_POINT ( 'NONE',  ( 1.779017513685136568E-09, 14.79893867758297610, -14.89095808115845720 ) ) ;
#17666=CARTESIAN_POINT ( 'NONE',  ( -15.25966316918061771, 10.19618095414378622, 19.47964375018031546 ) ) ;
#17675=AXIS2_PLACEMENT_3D ( 'NONE', #2303, #15125, #928 ) ;
#17679=CYLINDRICAL_SURFACE ( 'NONE', #8910, 17.50000000000000355 ) ;
#17683=AXIS2_PLACEMENT_3D ( 'NONE', #5917, #2953, #18858 ) ;
#17688=CARTESIAN_POINT ( 'NONE',  ( 2.163825119083639947E-09, 18.00000000000000355, -7.322699999819691108 ) ) ;
#17691=CARTESIAN_POINT ( 'NONE',  ( -8.382925371439625906, -12.54593441562639988, -5.487948168480926370 ) ) ;
#17698=CARTESIAN_POINT ( 'NONE',  ( 1.491842756249030399, 7.499999999820669672, 23.42698125018031519 ) ) ;
#17703=ORIENTED_EDGE ( 'NONE', *, *, #2089, .F. ) ;
#17714=PRESENTATION_STYLE_ASSIGNMENT (( #8368 ) ) ;
#17715=CARTESIAN_POINT ( 'NONE',  ( 5.303300859536635770, 5.303300858261589923, 24.31057500018031803 ) ) ;
#17717=CARTESIAN_POINT ( 'NONE',  ( 6.330490856366289165, -9.474249098604506258, 1.417546499713196795 ) ) ;
#17721=CIRCLE ( 'NONE', #9261, 16.99999999999995381 ) ;
#17725=CARTESIAN_POINT ( 'NONE',  ( -12.72792205982779912, 12.72792206288790950, 19.77417500018031404 ) ) ;
#17729=AXIS2_PLACEMENT_3D ( 'NONE', #570, #7020, #11794 ) ;
#17746=CARTESIAN_POINT ( 'NONE',  ( 3.599999999999902833, -10.82531754730554496, 43.00000000000000000 ) ) ;
#17766=CARTESIAN_POINT ( 'NONE',  ( 7.902369978624329327, 7.902369976724401113, 24.73948475064743135 ) ) ;
#17792=CARTESIAN_POINT ( 'NONE',  ( 17.99999999956958519, -3.580422614997676778, -4.671918749819693240 ) ) ;
#17793=EDGE_CURVE ( 'NONE', #2751, #20518, #10889, .T. ) ;
#17794=ORIENTED_EDGE ( 'NONE', *, *, #13625, .T. ) ;
#17797=CARTESIAN_POINT ( 'NONE',  ( -12.54593441764187034, -8.382925368423267187, -14.32388566848092992 ) ) ;
#17811=CARTESIAN_POINT ( 'NONE',  ( -17.99999999999999645, 2.163826221265758470E-09, 16.69145000018031055 ) ) ;
#17816=CARTESIAN_POINT ( 'NONE',  ( 6.250000000000054179, 10.82531754730546147, 40.00000000000000000 ) ) ;
#17823=CARTESIAN_POINT ( 'NONE',  ( 9.015937996181842420E-10, 7.500000000000007994, 13.70745000018031590 ) ) ;
#17824=CARTESIAN_POINT ( 'NONE',  ( 11.17563879704981566, -2.222972771497744304, 0.2394214997131979827 ) ) ;
#17829=ORIENTED_EDGE ( 'NONE', *, *, #5834, .F. ) ;
#17832=CARTESIAN_POINT ( 'NONE',  ( 2.163825119083639534E-09, 18.00000000000000000, 20.95230000018031546 ) ) ;
#17836=AXIS2_PLACEMENT_3D ( 'NONE', #4755, #9643, #1494 ) ;
#17849=LINE ( 'NONE', #11264, #1506 ) ;
#17852=CARTESIAN_POINT ( 'NONE',  ( 6.358192988180013216, 4.248408729364577141, 18.34020625018030870 ) ) ;
#17859=CARTESIAN_POINT ( 'NONE',  ( 15.25966317163202746, 10.19618095047498407, 20.52035625018031695 ) ) ;
#17874=CARTESIAN_POINT ( 'NONE',  ( -8.382925371439629458, -12.54593441562640876, -18.71986433115845827 ) ) ;
#17892=EDGE_CURVE ( 'NONE', #3529, #1354, #6819, .T. ) ;
#17896=CARTESIAN_POINT ( 'NONE',  ( 6.888301780572508193, -16.62983158603122291, -22.04926249981969377 ) ) ;
#17898=CARTESIAN_POINT ( 'NONE',  ( 9.015937996181835182E-10, 7.500000000000002665, 7.442550000180307990 ) ) ;
#17901=CARTESIAN_POINT ( 'NONE',  ( 8.382925368423265411, -12.54593441764187034, 2.169864331519073097 ) ) ;
#17906=CARTESIAN_POINT ( 'NONE',  ( -7.500000000000007994, -4.022542210876018231E-17, 20.77620000000231570 ) ) ;
#17915=ORIENTED_EDGE ( 'NONE', *, *, #4167, .F. ) ;
#17923=CARTESIAN_POINT ( 'NONE',  ( -7.499999999820669672, 1.491842756249032620, 11.64573125018031519 ) ) ;
#17924=CARTESIAN_POINT ( 'NONE',  ( 7.902369978624323110, 7.902369976724394895, -1.233234750286801296 ) ) ;
#17926=CARTESIAN_POINT ( 'NONE',  ( 0.000000000000000000, 0.000000000000000000, 40.00000000000000000 ) ) ;
#17929=CARTESIAN_POINT ( 'NONE',  ( -6.888301780572501976, 16.62983158603122291, 20.36323750018031475 ) ) ;
#17932=EDGE_CURVE ( 'NONE', #10000, #1316, #16792, .T. ) ;
#17934=ORIENTED_EDGE ( 'NONE', *, *, #16745, .F. ) ;
#17938=ORIENTED_EDGE ( 'NONE', *, *, #1398, .T. ) ;
#17945=CARTESIAN_POINT ( 'NONE',  ( 5.303300858261588147, -5.303300859536636658, -1.608174999819685702 ) ) ;
#17952=DIRECTION ( 'NONE',  ( 1.000000000000000000, 0.000000000000000000, 0.000000000000000000 ) ) ;
#17953=CIRCLE ( 'NONE', #1381, 7.500000000000000000 ) ;
#17963=CARTESIAN_POINT ( 'NONE',  ( 8.382925368423272516, -12.54593441764187745, -20.48705183115845685 ) ) ;
#17966=CARTESIAN_POINT ( 'NONE',  ( -12.50000000000000533, 0.000000000000000000, -40.00000000000000000 ) ) ;
#17972=CARTESIAN_POINT ( 'NONE',  ( -12.72792206288791128, -12.72792205982779912, 17.41792500018031475 ) ) ;
#17985=CARTESIAN_POINT ( 'NONE',  ( 2.163825119083639947E-09, 18.00000000000000355, -16.74769999981969093 ) ) ;
#17988=CARTESIAN_POINT ( 'NONE',  ( -6.929096493489627306, 2.870125743571138699, 5.675362500180308523 ) ) ;
#17991=CARTESIAN_POINT ( 'NONE',  ( -14.79893867758296544, 1.779018419858780125E-09, -13.44029191848092708 ) ) ;
#18004=CARTESIAN_POINT ( 'NONE',  ( 2.163825119083639120E-09, 17.99999999999999645, 19.04770000018030984 ) ) ;
#18012=( LENGTH_UNIT ( ) NAMED_UNIT ( * ) SI_UNIT ( .MILLI., .METRE. ) );
#18013=CARTESIAN_POINT ( 'NONE',  ( -2.870125743571144028, -6.929096493489630859, 9.584012500180316252 ) ) ;
#18016=CARTESIAN_POINT ( 'NONE',  ( -4.276731812588563386, 10.32494394809438987, 6.424577749713199282 ) ) ;
#18024=CARTESIAN_POINT ( 'NONE',  ( 15.25966317163202746, 10.19618095047498407, 22.42495625018031191 ) ) ;
#18034=ORIENTED_EDGE ( 'NONE', *, *, #355, .T. ) ;
#18043=ORIENTED_EDGE ( 'NONE', *, *, #3165, .F. ) ;
#18049=CYLINDRICAL_SURFACE ( 'NONE', #5551, 7.500000000000000000 ) ;
#18071=CARTESIAN_POINT ( 'NONE',  ( -1.343452921478824119E-09, -11.17563879731705789, 9.423859750647428868 ) ) ;
#18095=CARTESIAN_POINT ( 'NONE',  ( -13.67243654778936168, -5.663308646854336992, 19.86372941884154741 ) ) ;
#18097=CARTESIAN_POINT ( 'NONE',  ( 2.870125743571138255, 6.929096493489627306, 8.031612500180308700 ) ) ;
#18100=CARTESIAN_POINT ( 'NONE',  ( -13.67243654642775041, 5.663308650141531508, -3.426229418480926991 ) ) ;
#18111=CARTESIAN_POINT ( 'NONE',  ( -12.72792205982779556, 12.72792206288790773, 17.86957500018031197 ) ) ;
#18113=EDGE_LOOP ( 'NONE', ( #17618, #16906, #6498, #8761 ) ) ;
#18117=FACE_OUTER_BOUND ( 'NONE', #4816, .T. ) ;
#18122=CARTESIAN_POINT ( 'NONE',  ( -7.500000000179346316, -1.491842754445844355, 11.05666875018031625 ) ) ;
#18124=CARTESIAN_POINT ( 'NONE',  ( 9.474249098604504482, 6.330490856366291830, 8.486296499713199992 ) ) ;
#18125=PRODUCT_DEFINITION_SHAPE ( 'NONE', 'NONE',  #20880 ) ;
#18130=CARTESIAN_POINT ( 'NONE',  ( -6.888301784570738384, -16.62983158437509346, 7.403862500180314221 ) ) ;
#18145=CARTESIAN_POINT ( 'NONE',  ( -7.500000000000000888, 9.015942588607330751E-10, 5.086300000180312253 ) ) ;
#18154=ORIENTED_EDGE ( 'NONE', *, *, #15854, .F. ) ;
#18175=CARTESIAN_POINT ( 'NONE',  ( -11.17563879758428769, -2.222972768810840272, 11.48557850064743135 ) ) ;
#18185=CARTESIAN_POINT ( 'NONE',  ( 18.00000000043041126, 3.580422610670019434, 4.164018750180312090 ) ) ;
#18198=ADVANCED_FACE ( 'NONE', ( #14762 ), #18049, .T. ) ;
#18201=CARTESIAN_POINT ( 'NONE',  ( -1.779019326032424922E-09, -14.79893867758297610, 18.09654191884154883 ) ) ;
#18206=CARTESIAN_POINT ( 'NONE',  ( -8.382925368423267187, 12.54593441764186856, -21.39263566848092424 ) ) ;
#18212=CARTESIAN_POINT ( 'NONE',  ( -6.358192987158592047, 4.248408730893246776, 15.39489375018031048 ) ) ;
#18217=CARTESIAN_POINT ( 'NONE',  ( 18.00000000043040771, 3.580422610670018546, 11.68441875018030984 ) ) ;
#18223=CARTESIAN_POINT ( 'NONE',  ( 12.72792206288791128, 12.72792205982780267, 22.13042500018031333 ) ) ;
#18226=CARTESIAN_POINT ( 'NONE',  ( 2.870125743571140475, 6.929096493489632635, 4.871512500180315008 ) ) ;
#18228=CARTESIAN_POINT ( 'NONE',  ( 11.17563879731704723, -1.343450868547281106E-09, -18.90510975028680818 ) ) ;
#18234=CARTESIAN_POINT ( 'NONE',  ( -18.00000000000000000, 2.163826221265758884E-09, -9.678949999819687733 ) ) ;
#18254=CARTESIAN_POINT ( 'NONE',  ( 16.62983158603122291, 6.888301780572502864, 20.81488750018031553 ) ) ;
#18261=CARTESIAN_POINT ( 'NONE',  ( 18.00000000000000000, -2.163824016901520184E-09, -24.76874999981969339 ) ) ;
#18266=CARTESIAN_POINT ( 'NONE',  ( -16.62983158437509701, 6.888301784570728614, -1.569487499819690379 ) ) ;
#18269=CARTESIAN_POINT ( 'NONE',  ( 6.249999999999902300, -10.82531754730554496, 43.00000000000000000 ) ) ;
#18270=CARTESIAN_POINT ( 'NONE',  ( -2.222972768810837607, 11.17563879758428769, 13.84182850064743064 ) ) ;
#18276=VERTEX_POINT ( 'NONE', #3217 ) ;
#18277=CARTESIAN_POINT ( 'NONE',  ( -10.19618095047498052, 15.25966317163203101, 1.218706250180313866 ) ) ;
#18293=CARTESIAN_POINT ( 'NONE',  ( 14.79893867722910450, -2.943691928843438443, 16.03482316884154812 ) ) ;
#18297=ORIENTED_EDGE ( 'NONE', *, *, #1323, .T. ) ;
#18300=CARTESIAN_POINT ( 'NONE',  ( 10.46442989202483531, -10.46442989454075168, -26.39966691848093561 ) ) ;
#18307=CARTESIAN_POINT ( 'NONE',  ( -5.303300858261584594, 5.303300859536631329, 15.68942500018031083 ) ) ;
#18309=CARTESIAN_POINT ( 'NONE',  ( -6.929096494179684207, -2.870125741905212635, 10.76213750018031590 ) ) ;
#18312=CARTESIAN_POINT ( 'NONE',  ( 10.19618095047497697, -15.25966317163202923, 13.45160625018031197 ) ) ;
#18320=CARTESIAN_POINT ( 'NONE',  ( -7.500000000000009770, 9.706494107251932559E-15, -16.92379999999768359 ) ) ;
#18323=CARTESIAN_POINT ( 'NONE',  ( 7.500000000179346316, 1.491842754445843244, -3.080831249819684814 ) ) ;
#18326=CARTESIAN_POINT ( 'NONE',  ( 9.474249097082495297, -6.330490858644137298, -18.02151600028679823 ) ) ;
#18333=CARTESIAN_POINT ( 'NONE',  ( 15.25966316918061416, -10.19618095414378622, 5.342143750180314399 ) ) ;
#18347=VECTOR ( 'NONE', #849, 1000.000000000000000 ) ;
#18350=CARTESIAN_POINT ( 'NONE',  ( 6.929096493489624642, -2.870125743571141363, 0.9628625001803121641 ) ) ;
#18357=CARTESIAN_POINT ( 'NONE',  ( 12.72792206288790950, 12.72792205982780089, 10.80082500018031411 ) ) ;
#18363=ORIENTED_EDGE ( 'NONE', *, *, #7266, .T. ) ;
#18372=CARTESIAN_POINT ( 'NONE',  ( 3.580422610670019878, -18.00000000043040771, -14.23433124981968767 ) ) ;
#18375=CARTESIAN_POINT ( 'NONE',  ( 1.343451552857795926E-09, 11.17563879731705789, 14.13635975064743100 ) ) ;
#18385=CARTESIAN_POINT ( 'NONE',  ( -3.580422610670018546, 18.00000000043041126, 1.807768750180311468 ) ) ;
#18392=CARTESIAN_POINT ( 'NONE',  ( 6.929096494179683319, 2.870125741905213079, 15.47463750018031625 ) ) ;
#18394=VECTOR ( 'NONE', #19642, 1000.000000000000000 ) ;
#18400=SHAPE_DEFINITION_REPRESENTATION ( #18125, #9416 ) ;
#18402=CARTESIAN_POINT ( 'NONE',  ( -5.663308646854337880, 13.67243654778935991, 12.79497941884154777 ) ) ;
#18411=CARTESIAN_POINT ( 'NONE',  ( 16.62983158603121936, 6.888301780572501976, 20.81488750018031197 ) ) ;
#18417=DIRECTION ( 'NONE',  ( 0.000000000000000000, 0.000000000000000000, 1.000000000000000000 ) ) ;
#18420=ORIENTED_EDGE ( 'NONE', *, *, #7210, .F. ) ;
#18424=CARTESIAN_POINT ( 'NONE',  ( 3.580422614997667896, 17.99999999956958163, 0.4922312501803097207 ) ) ;
#18433=EDGE_CURVE ( 'NONE', #10000, #19384, #8473, .T. ) ;
#18435=CARTESIAN_POINT ( 'NONE',  ( -2.870125743571144028, -6.929096493489630859, 0.1590125001803138760 ) ) ;
#18436=CARTESIAN_POINT ( 'NONE',  ( -2.870125743571144028, -6.929096493489630859, 19.00901250018031519 ) ) ;
#18437=CARTESIAN_POINT ( 'NONE',  ( 9.474249098604504482, 6.330490856366291830, -19.78870350028680747 ) ) ;
#18443=CARTESIAN_POINT ( 'NONE',  ( 17.99999999956958163, -3.580422614997676334, -4.671918749819689687 ) ) ;
#18445=ORIENTED_EDGE ( 'NONE', *, *, #2175, .F. ) ;
#18457=CARTESIAN_POINT ( 'NONE',  ( -5.303300859536631329, -5.303300858261583706, -14.94182499981969237 ) ) ;
#18467=CARTESIAN_POINT ( 'NONE',  ( -16.62983158437510056, 6.888301784570729502, 7.855512500180314106 ) ) ;
#18479=CARTESIAN_POINT ( 'NONE',  ( 3.580422614997667896, 17.99999999956958163, -18.35776874981969442 ) ) ;
#18484=CARTESIAN_POINT ( 'NONE',  ( 4.276731815070943910, 10.32494394706616703, 14.72542225064742993 ) ) ;
#18494=CARTESIAN_POINT ( 'NONE',  ( -12.72792206288791128, -12.72792205982779912, 7.992925000180314044 ) ) ;
#18502=CARTESIAN_POINT ( 'NONE',  ( -1.491842754445842800, 7.500000000179346316, 13.41291875018031554 ) ) ;
#18506=CARTESIAN_POINT ( 'NONE',  ( 7.500000000000000888, -9.015933403756337545E-10, 19.22380000018031154 ) ) ;
#18513=CARTESIAN_POINT ( 'NONE',  ( 12.54593441764187567, 8.382925368423276069, 14.85669816884154848 ) ) ;
#18519=CIRCLE ( 'NONE', #240, 2.649999999999999467 ) ;
#18520=CARTESIAN_POINT ( 'NONE',  ( -17.99999999999999645, 2.163826221265758470E-09, 16.69145000018031055 ) ) ;
#18525=CARTESIAN_POINT ( 'NONE',  ( 6.929096494179677990, 2.870125741905210859, 18.63473750018030728 ) ) ;
#18532=CARTESIAN_POINT ( 'NONE',  ( -15.25966317163202923, -10.19618095047497874, 6.382856250180309665 ) ) ;
#18544=CARTESIAN_POINT ( 'NONE',  ( -6.929096493489632635, 2.870125743571140919, -16.33473749981968837 ) ) ;
#18546=CARTESIAN_POINT ( 'NONE',  ( -1.491842754445842800, 7.500000000179346316, 3.987918750180313054 ) ) ;
#18548=CARTESIAN_POINT ( 'NONE',  ( 1.343451552857795099E-09, 11.17563879731704723, -11.83635975028680498 ) ) ;
#18552=ORIENTED_EDGE ( 'NONE', *, *, #4341, .F. ) ;
#18554=CARTESIAN_POINT ( 'NONE',  ( 6.888301784570728614, 16.62983158437510056, 2.691362500180312978 ) ) ;
#18557=EDGE_CURVE ( 'NONE', #6717, #20518, #16219, .T. ) ;
#18566=EDGE_CURVE ( 'NONE', #9811, #8208, #17223, .T. ) ;
#18569=CARTESIAN_POINT ( 'NONE',  ( 7.500000000179339210, 1.491842754445841690, -9.345731249819689168 ) ) ;
#18575=EDGE_CURVE ( 'NONE', #1825, #9811, #1088, .T. ) ;
#18578=ORIENTED_EDGE ( 'NONE', *, *, #6484, .T. ) ;
#18579=CARTESIAN_POINT ( 'NONE',  ( -15.25966316918061771, 10.19618095414378622, -1.274956249819686471 ) ) ;
#18590=CARTESIAN_POINT ( 'NONE',  ( -18.00000000043040771, -3.580422610670021211, -11.87808124981969016 ) ) ;
#18593=CARTESIAN_POINT ( 'NONE',  ( -9.474249098604513364, -6.330490856366295382, -7.953483999352573441 ) ) ;
#18600=CARTESIAN_POINT ( 'NONE',  ( -16.62983158603122291, -6.888301780572501087, 8.581987500180312978 ) ) ;
#18606=CARTESIAN_POINT ( 'NONE',  ( 5.303300859536635770, 5.303300858261589923, 14.88557500018031554 ) ) ;
#18614=CARTESIAN_POINT ( 'NONE',  ( 12.54593441764187567, 8.382925368423276069, -3.993301831158456050 ) ) ;
#18619=CARTESIAN_POINT ( 'NONE',  ( 12.54593441562639988, -8.382925371439625906, -17.26919816848092637 ) ) ;
#18628=CARTESIAN_POINT ( 'NONE',  ( 15.25966317163202568, 10.19618095047498230, 1.670356250180308422 ) ) ;
#18629=EDGE_LOOP ( 'NONE', ( #16044, #7441, #1056, #19282 ) ) ;
#18639=CARTESIAN_POINT ( 'NONE',  ( 9.015937996181842420E-10, 7.500000000000007994, -5.142549999819685524 ) ) ;
#18643=CARTESIAN_POINT ( 'NONE',  ( -9.474249098604506258, -6.330490856366290053, -24.50120350028680960 ) ) ;
#18648=CARTESIAN_POINT ( 'NONE',  ( 18.00000000043041126, 3.580422610670019434, 4.164018750180312090 ) ) ;
#18665=CARTESIAN_POINT ( 'NONE',  ( 2.870125743571137811, 6.929096493489625530, -1.393387499819688458 ) ) ;
#18676=CARTESIAN_POINT ( 'NONE',  ( 6.888301784570728614, 16.62983158437510056, 0.7867625001803136842 ) ) ;
#18692=CARTESIAN_POINT ( 'NONE',  ( -3.580422610670017658, 18.00000000043040771, -0.09683124981969132294 ) ) ;
#18696=CARTESIAN_POINT ( 'NONE',  ( 11.17563879704982632, -2.222972771497745637, -2.062858999352573441 ) ) ;
#18703=CARTESIAN_POINT ( 'NONE',  ( 7.575000000000064126, 13.12028486733421850, -43.00000000000000000 ) ) ;
#18707=CARTESIAN_POINT ( 'NONE',  ( 16.62983158603122291, 6.888301780572502864, -5.555512499819688088 ) ) ;
#18723=CARTESIAN_POINT ( 'NONE',  ( 13.67243654778935991, 5.663308646854338768, -3.698770581158455695 ) ) ;
#18730=CARTESIAN_POINT ( 'NONE',  ( 10.19618095047497697, -15.25966317163202923, 4.026606250180309488 ) ) ;
#18731=CARTESIAN_POINT ( 'NONE',  ( 0.000000000000000000, 0.000000000000000000, -40.00000000000000000 ) ) ;
#18743=CARTESIAN_POINT ( 'NONE',  ( -1.491842756249031954, -7.499999999820663454, 3.024581250180308434 ) ) ;
#18744=CARTESIAN_POINT ( 'NONE',  ( -6.888301780572500199, 16.62983158603121936, -9.816362499819691223 ) ) ;
#18747=ORIENTED_EDGE ( 'NONE', *, *, #15037, .F. ) ;
#18755=CARTESIAN_POINT ( 'NONE',  ( -15.25966316918061949, 10.19618095414378800, 10.05464375018031120 ) ) ;
#18759=ORIENTED_EDGE ( 'NONE', *, *, #16034, .T. ) ;
#18761=CARTESIAN_POINT ( 'NONE',  ( -1.779019326032424095E-09, -14.79893867758296544, 12.47845808151907754 ) ) ;
#18782=CARTESIAN_POINT ( 'NONE',  ( -5.303300858261583706, 5.303300859536630441, -12.58557499981968775 ) ) ;
#18783=DIRECTION ( 'NONE',  ( -0.000000000000000000, -0.000000000000000000, 1.000000000000000000 ) ) ;
#18789=CARTESIAN_POINT ( 'NONE',  ( -2.163827323447878234E-09, -18.00000000000000000, -23.36479999981968803 ) ) ;
#18795=CARTESIAN_POINT ( 'NONE',  ( -7.500000000000004441, -1.491842754878798916, -4.633231249912213023 ) ) ;
#18797=CARTESIAN_POINT ( 'NONE',  ( -7.500000000000000888, 1.491842755816075172, -4.044168749912214089 ) ) ;
#18803=CARTESIAN_POINT ( 'NONE',  ( -17.99999999956958163, 3.580422614997673669, -20.71401874981969371 ) ) ;
#18806=ADVANCED_FACE ( 'NONE', ( #16421 ), #1909, .T. ) ;
#18811=VERTEX_POINT ( 'NONE', #10072 ) ;
#18816=CARTESIAN_POINT ( 'NONE',  ( -18.00000000043041126, -3.580422610670022099, -19.39848124981969235 ) ) ;
#18833=CARTESIAN_POINT ( 'NONE',  ( 2.943691925285398803, -14.79893867793684059, -1.047989331158453830 ) ) ;
#18838=CARTESIAN_POINT ( 'NONE',  ( 16.62983158603121936, 6.888301780572501976, 11.38988750018031126 ) ) ;
#18850=CARTESIAN_POINT ( 'NONE',  ( -3.580422614997674557, -17.99999999956957808, -13.64526874981969407 ) ) ;
#18858=DIRECTION ( 'NONE',  ( 1.000000000000000000, 0.000000000000000000, 0.000000000000000000 ) ) ;
#18861=CARTESIAN_POINT ( 'NONE',  ( -10.19618095047498230, 15.25966317163203279, 1.218706250180310313 ) ) ;
#18868=CARTESIAN_POINT ( 'NONE',  ( 2.943691928843430450, 14.79893867722910095, 8.060489331519073986 ) ) ;
#18872=CARTESIAN_POINT ( 'NONE',  ( 7.500000000000000000, -9.015933403756343749E-10, 25.48870000018031590 ) ) ;
#18874=CARTESIAN_POINT ( 'NONE',  ( -12.72792206288791128, -12.72792205982779912, -20.28207499981969164 ) ) ;
#18894=CARTESIAN_POINT ( 'NONE',  ( 11.17563879758427525, 2.222972768810836719, 18.50035899971319608 ) ) ;
#18896=CARTESIAN_POINT ( 'NONE',  ( 17.50000000000000355, 2.143131898507868643E-15, 43.00000000000000000 ) ) ;
#18901=CARTESIAN_POINT ( 'NONE',  ( 6.888301780572507305, -16.62983158603121936, -23.95386249981968874 ) ) ;
#18907=DIRECTION ( 'NONE',  ( -0.000000000000000000, -0.000000000000000000, -1.000000000000000000 ) ) ;
#18908=CARTESIAN_POINT ( 'NONE',  ( 7.500000000000000888, 4.207617034106124418E-15, 0.3738000000023073421 ) ) ;
#18912=CARTESIAN_POINT ( 'NONE',  ( -6.888301784570736608, -16.62983158437509346, -22.77573749981969087 ) ) ;
#18924=CARTESIAN_POINT ( 'NONE',  ( 3.580422610670020322, -18.00000000043041126, -21.75473124981968809 ) ) ;
#18925=FACE_OUTER_BOUND ( 'NONE', #11017, .T. ) ;
#18935=CARTESIAN_POINT ( 'NONE',  ( -8.382925371439629458, -12.54593441562640876, -9.294864331158457560 ) ) ;
#18941=CARTESIAN_POINT ( 'NONE',  ( 6.888301784570727726, 16.62983158437509701, 0.7867625001803102425 ) ) ;
#18943=DIRECTION ( 'NONE',  ( 1.000000000000000000, 0.000000000000000000, 0.000000000000000000 ) ) ;
#18951=CARTESIAN_POINT ( 'NONE',  ( -5.303300859536632217, -5.303300858261584594, 3.908175000180308611 ) ) ;
#18952=CARTESIAN_POINT ( 'NONE',  ( 15.25966316918061239, -10.19618095414378445, -5.987456249819691045 ) ) ;
#18960=CARTESIAN_POINT ( 'NONE',  ( -15.25966317163203456, -10.19618095047498230, 8.287456250180309070 ) ) ;
#18963=CARTESIAN_POINT ( 'NONE',  ( 1.491842756249030622, 7.499999999820669672, -14.27301874981968943 ) ) ;
#18966=CARTESIAN_POINT ( 'NONE',  ( -13.67243654642775041, 5.663308650141531508, 15.42377058151907754 ) ) ;
#18972=CARTESIAN_POINT ( 'NONE',  ( -6.888301780572501976, 16.62983158603122291, -17.33676249981968809 ) ) ;
#18986=CARTESIAN_POINT ( 'NONE',  ( 9.015937996181834148E-10, 7.500000000000000888, -20.83244999981968704 ) ) ;
#18988=FACE_OUTER_BOUND ( 'NONE', #20040, .T. ) ;
#18994=CARTESIAN_POINT ( 'NONE',  ( -12.72792205982779912, 12.72792206288790950, -10.40542499981968483 ) ) ;
#19000=CARTESIAN_POINT ( 'NONE',  ( -6.358192988180015881, -4.248408729364577141, -5.222293749819692188 ) ) ;
#19002=CARTESIAN_POINT ( 'NONE',  ( 6.929096494179677990, 2.870125741905210859, -0.2152624998196933648 ) ) ;
#19007=CARTESIAN_POINT ( 'NONE',  ( -10.19618095414378445, -15.25966316918061239, -22.48120624981969229 ) ) ;
#19013=DIRECTION ( 'NONE',  ( -0.000000000000000000, -0.000000000000000000, 1.000000000000000000 ) ) ;
#19021=CARTESIAN_POINT ( 'NONE',  ( 15.25966316918061416, -10.19618095414378622, -4.082856249819688088 ) ) ;
#19036=CARTESIAN_POINT ( 'NONE',  ( -8.382925368423274293, 12.54593441764187745, -6.349551831158453119 ) ) ;
#19038=AXIS2_PLACEMENT_3D ( 'NONE', #20555, #8894, #12507 ) ;
#19040=CARTESIAN_POINT ( 'NONE',  ( -7.500000000000004441, 9.706494115430842424E-15, -13.76369999999769256 ) ) ;
#19045=CARTESIAN_POINT ( 'NONE',  ( 3.580422614997667896, 17.99999999956958163, 0.4922312501803097207 ) ) ;
#19048=ORIENTED_EDGE ( 'NONE', *, *, #20190, .T. ) ;
#19054=CARTESIAN_POINT ( 'NONE',  ( 5.303300858261583706, -5.303300859536632217, 1.551925000180306213 ) ) ;
#19055=CARTESIAN_POINT ( 'NONE',  ( -16.62983158437509701, 6.888301784570728614, -10.99448749981968909 ) ) ;
#19063=DIRECTION ( 'NONE',  ( 1.000000000000000000, 0.000000000000000000, 0.000000000000000000 ) ) ;
#19066=CARTESIAN_POINT ( 'NONE',  ( 10.19618095414378978, 15.25966316918061771, 2.985893750180310224 ) ) ;
#19073=CARTESIAN_POINT ( 'NONE',  ( 5.663308650141530620, 13.67243654642775041, 17.78002058151907860 ) ) ;
#19096=DIRECTION ( 'NONE',  ( -0.000000000000000000, -0.000000000000000000, -1.000000000000000000 ) ) ;
#19097=CARTESIAN_POINT ( 'NONE',  ( -2.222972768810837607, 11.17563879758428769, -5.008171499352571665 ) ) ;
#19100=CARTESIAN_POINT ( 'NONE',  ( 6.929096493489624642, -2.870125743571141363, -17.88713749981969059 ) ) ;
#19108=CARTESIAN_POINT ( 'NONE',  ( -18.00000000000000000, 2.163826221265758884E-09, -11.58354999981968803 ) ) ;
#19120=CARTESIAN_POINT ( 'NONE',  ( -15.25966317163202923, -10.19618095047497874, -21.89214374981969513 ) ) ;
#19123=CARTESIAN_POINT ( 'NONE',  ( -2.870125743571141808, -6.929096493489625530, 12.74411250018030906 ) ) ;
#19133=CARTESIAN_POINT ( 'NONE',  ( -10.19618095414378622, -15.25966316918061416, -20.57660624981969377 ) ) ;
#19137=DIRECTION ( 'NONE',  ( -0.000000000000000000, -0.000000000000000000, -1.000000000000000000 ) ) ;
#19145=CARTESIAN_POINT ( 'NONE',  ( -10.46442989454075878, -10.46442989202484242, -18.42533308115845969 ) ) ;
#19147=CARTESIAN_POINT ( 'NONE',  ( 4.248408729364576253, -6.358192988180015881, -17.00354374981969130 ) ) ;
#19154=EDGE_LOOP ( 'NONE', ( #20810, #11426, #2158, #6783 ) ) ;
#19161=CARTESIAN_POINT ( 'NONE',  ( -10.19618095414378445, -15.25966316918061239, -22.48120624981969584 ) ) ;
#19166=CARTESIAN_POINT ( 'NONE',  ( 16.62983158437509701, -6.888301784570740161, 14.47261250018030942 ) ) ;
#19168=CARTESIAN_POINT ( 'NONE',  ( 7.500000000179346316, 1.491842754445843244, -12.50583124981968908 ) ) ;
#19173=CARTESIAN_POINT ( 'NONE',  ( 14.79893867758296544, -1.779016607511491977E-09, 10.12220808151907470 ) ) ;
#19185=VERTEX_POINT ( 'NONE', #370 ) ;
#19187=DIRECTION ( 'NONE',  ( 1.000000000000000000, 0.000000000000000000, 0.000000000000000000 ) ) ;
#19196=CARTESIAN_POINT ( 'NONE',  ( -7.902369976724401113, 7.902369978624329327, -15.31676524935257078 ) ) ;
#19198=CARTESIAN_POINT ( 'NONE',  ( 11.17563879731704723, -1.343450868547281106E-09, 18.79489024971320177 ) ) ;
#19202=CARTESIAN_POINT ( 'NONE',  ( 6.249999999999902300, -10.82531754730554496, -40.00000000000000000 ) ) ;
#19209=CARTESIAN_POINT ( 'NONE',  ( -10.19618095047498052, 15.25966317163203101, -19.53589374981968518 ) ) ;
#19214=DIRECTION ( 'NONE',  ( 0.000000000000000000, 0.000000000000000000, -1.000000000000000000 ) ) ;
#19215=CARTESIAN_POINT ( 'NONE',  ( -7.500000000000004441, 9.706494107352906755E-15, -4.338699999997692736 ) ) ;
#19239=ORIENTED_EDGE ( 'NONE', *, *, #11818, .T. ) ;
#19243=CARTESIAN_POINT ( 'NONE',  ( 6.249999999999902300, -10.82531754730554496, -43.00000000000000000 ) ) ;
#19244=CARTESIAN_POINT ( 'NONE',  ( 2.943691928843431782, 14.79893867722910628, -14.59642683115845863 ) ) ;
#19252=EDGE_LOOP ( 'NONE', ( #11072, #5426 ) ) ;
#19259=DIRECTION ( 'NONE',  ( -0.000000000000000000, -0.000000000000000000, 1.000000000000000000 ) ) ;
#19262=CARTESIAN_POINT ( 'NONE',  ( 9.470358143689558972, -1.138454911109687490E-09, -38.52172829718890057 ) ) ;
#19266=CARTESIAN_POINT ( 'NONE',  ( -16.62983158603122646, -6.888301780572501976, -10.26801249981969200 ) ) ;
#19269=CARTESIAN_POINT ( 'NONE',  ( 12.54593441764186679, 8.382925368423272516, -9.611385668480929567 ) ) ;
#19273=CARTESIAN_POINT ( 'NONE',  ( 2.870125743571140475, 6.929096493489632635, 23.72151250018031732 ) ) ;
#19282=ORIENTED_EDGE ( 'NONE', *, *, #6484, .F. ) ;
#19287=CARTESIAN_POINT ( 'NONE',  ( 11.17563879731705789, -1.343450868547281933E-09, -2.357390249352570688 ) ) ;
#19288=CARTESIAN_POINT ( 'NONE',  ( -7.902369978624323110, -7.902369976724391343, 3.479265249713199282 ) ) ;
#19297=CARTESIAN_POINT ( 'NONE',  ( 18.00000000000000000, -2.163824016901520184E-09, 13.88355000018031404 ) ) ;
#19308=CYLINDRICAL_SURFACE ( 'NONE', #14308, 2.650000000000000355 ) ;
#19310=EDGE_CURVE ( 'NONE', #19185, #2818, #4994, .T. ) ;
#19317=CARTESIAN_POINT ( 'NONE',  ( -7.500000000000004441, 9.706494115430842424E-15, -13.76369999999769256 ) ) ;
#19339=CARTESIAN_POINT ( 'NONE',  ( 1.343451552857795926E-09, 11.17563879731705789, 23.56135975064743349 ) ) ;
#19359=CARTESIAN_POINT ( 'NONE',  ( 7.500000000000009770, -8.788009017158368372E-15, -2.786299999997682519 ) ) ;
#19365=CARTESIAN_POINT ( 'NONE',  ( -18.00000000000000355, 2.163826221265759298E-09, -19.10394999981969377 ) ) ;
#19369=CARTESIAN_POINT ( 'NONE',  ( -5.663308646854335215, 13.67243654778934925, -11.67310441848092673 ) ) ;
#19383=CARTESIAN_POINT ( 'NONE',  ( 18.00000000043040771, 3.580422610670018546, 21.10941875018031055 ) ) ;
#19384=VERTEX_POINT ( 'NONE', #8739 ) ;
#19393=CARTESIAN_POINT ( 'NONE',  ( 1.491842756249030622, 7.499999999820669672, 23.42698125018031519 ) ) ;
#19394=CARTESIAN_POINT ( 'NONE',  ( 4.276731812588566939, -10.32494394809438809, 11.13707774971319964 ) ) ;
#19404=CARTESIAN_POINT ( 'NONE',  ( -12.72792206288791128, -12.72792205982779912, 17.41792500018031475 ) ) ;
#19407=ORIENTED_EDGE ( 'NONE', *, *, #9724, .T. ) ;
#19425=CARTESIAN_POINT ( 'NONE',  ( 2.870125743571137811, 6.929096493489625530, 17.45661250018031296 ) ) ;
#19426=CARTESIAN_POINT ( 'NONE',  ( 7.500000000000009770, -8.788009017158368372E-15, -2.786299999997682519 ) ) ;
#19431=CARTESIAN_POINT ( 'NONE',  ( -18.00000000043041126, -3.580422610670022543, 16.39691875018031908 ) ) ;
#19445=CARTESIAN_POINT ( 'NONE',  ( -10.32494394809439875, -4.276731812588566051, 20.61604725064743704 ) ) ;
#19447=DIRECTION ( 'NONE',  ( -0.000000000000000000, -0.000000000000000000, 1.000000000000000000 ) ) ;
#19449=ORIENTED_EDGE ( 'NONE', *, *, #20065, .F. ) ;
#19453=CARTESIAN_POINT ( 'NONE',  ( -3.580422614997675002, -17.99999999956958163, 16.53433125018031191 ) ) ;
#19455=DIRECTION ( 'NONE',  ( 1.000000000000000000, 0.000000000000000000, 0.000000000000000000 ) ) ;
#19464=CARTESIAN_POINT ( 'NONE',  ( -1.491842754445842800, 7.500000000179346316, -5.437081249819685880 ) ) ;
#19471=CARTESIAN_POINT ( 'NONE',  ( -18.00000000043041481, -3.580422610670022987, -19.39848124981969590 ) ) ;
#19473=DIRECTION ( 'NONE',  ( 0.000000000000000000, 0.000000000000000000, 1.000000000000000000 ) ) ;
#19474=CARTESIAN_POINT ( 'NONE',  ( 0.000000000000000000, 0.000000000000000000, 0.000000000000000000 ) ) ;
#19476=CARTESIAN_POINT ( 'NONE',  ( 8.382925371439627682, 12.54593441562639988, -10.20044816848092673 ) ) ;
#19483=CARTESIAN_POINT ( 'NONE',  ( 9.015937996181842420E-10, 7.500000000000007994, 23.13245000018031661 ) ) ;
#19489=CARTESIAN_POINT ( 'NONE',  ( -12.72792206288790950, -12.72792205982779556, 15.51332500018031268 ) ) ;
#19499=CARTESIAN_POINT ( 'NONE',  ( 2.870125743571140475, 6.929096493489632635, 14.29651250018031661 ) ) ;
#19500=CARTESIAN_POINT ( 'NONE',  ( 2.222972771497739419, 11.17563879704981922, 7.308171499713199459 ) ) ;
#19507=CARTESIAN_POINT ( 'NONE',  ( -2.163827323447878234E-09, -18.00000000000000000, 6.814800000180313511 ) ) ;
#19529=CARTESIAN_POINT ( 'NONE',  ( -1.491842756249031510, -7.499999999820660790, 12.44958125018031225 ) ) ;
#19536=ORIENTED_EDGE ( 'NONE', *, *, #17633, .T. ) ;
#19537=CARTESIAN_POINT ( 'NONE',  ( -10.19618095414378622, -15.25966316918061416, 15.21879375018031411 ) ) ;
#19550=CARTESIAN_POINT ( 'NONE',  ( 5.663308650141532397, 13.67243654642775574, -14.30189558115846182 ) ) ;
#19551=ADVANCED_FACE ( 'NONE', ( #18925 ), #17329, .F. ) ;
#19559=CARTESIAN_POINT ( 'NONE',  ( 6.888301784570728614, 16.62983158437510056, 21.54136250018031618 ) ) ;
#19568=CARTESIAN_POINT ( 'NONE',  ( 16.62983158437509346, -6.888301784570737496, -25.13198749981969371 ) ) ;
#19572=CARTESIAN_POINT ( 'NONE',  ( 12.72792206288791128, 12.72792205982780267, -6.144574999819692351 ) ) ;
#19579=CARTESIAN_POINT ( 'NONE',  ( -2.943691925285395694, 14.79893867793683349, -11.37857316848092637 ) ) ;
#19602=CARTESIAN_POINT ( 'NONE',  ( -4.248408729364580694, 6.358192988180020322, 22.24885625018031732 ) ) ;
#19603=CARTESIAN_POINT ( 'NONE',  ( -4.276731815070945686, -10.32494394706615637, 12.31520274971320106 ) ) ;
#19608=CARTESIAN_POINT ( 'NONE',  ( -10.19618095047498052, 15.25966317163203101, 20.06870625018031262 ) ) ;
#19617=DIRECTION ( 'NONE',  ( -1.000000000000000000, 0.000000000000000000, 0.000000000000000000 ) ) ;
#19618=( NAMED_UNIT ( * ) SI_UNIT ( $, .STERADIAN. ) SOLID_ANGLE_UNIT ( ) );
#19622=CARTESIAN_POINT ( 'NONE',  ( -7.500000000179339210, -1.491842754445842800, 14.21676875018031261 ) ) ;
#19630=EDGE_LOOP ( 'NONE', ( #16509, #19796 ) ) ;
#19642=DIRECTION ( 'NONE',  ( 0.000000000000000000, 0.000000000000000000, -1.000000000000000000 ) ) ;
#19644=CARTESIAN_POINT ( 'NONE',  ( 7.902369978624329327, 7.902369976724401113, 15.31448475064743242 ) ) ;
#19652=CARTESIAN_POINT ( 'NONE',  ( -2.163827323447878234E-09, -18.00000000000000000, 16.23980000018031333 ) ) ;
#19661=CARTESIAN_POINT ( 'NONE',  ( -6.929096494179684207, -2.870125741905212635, -17.51286249981968979 ) ) ;
#19666=( BOUNDED_CURVE ( )  B_SPLINE_CURVE ( 2, ( #710, #5270, #18525, #5470, #10467, #300, #16605, #2308, #3573, #11743, #10150, #6751, #18307, #18212, #13229, #8656, #2197 ),
 .UNSPECIFIED., .F., .T. ) 
 B_SPLINE_CURVE_WITH_KNOTS ( ( 3, 2, 2, 2, 2, 2, 2, 2, 3 ),
 ( 0.000000000000000000, 0.01250000000048139860, 0.02500000000096279720, 0.03750000000144419060, 0.05000000000192559441, 0.06250000000240699127, 0.07500000000288838120, 0.08750000000336977113, 0.1000000000038511888 ),
 .UNSPECIFIED. ) 
 CURVE ( )  GEOMETRIC_REPRESENTATION_ITEM ( )  RATIONAL_B_SPLINE_CURVE ( ( 1.000000000000000000, 0.9807852804032304306, 1.000000000000000000, 0.9807852804032304306, 1.000000000000000000, 0.9807852804032304306, 1.000000000000000000, 0.9807852804032304306, 1.000000000000000000, 0.9807852804032304306, 1.000000000000000000, 0.9807852804032304306, 1.000000000000000000, 0.9807852804032304306, 1.000000000000000000, 0.9807852803973104994, 1.000000000005919931 ) ) 
 REPRESENTATION_ITEM ( '' )  );
#19667=CARTESIAN_POINT ( 'NONE',  ( -8.382925368423274293, 12.54593441764187745, 12.50044816884154564 ) ) ;
#19671=CARTESIAN_POINT ( 'NONE',  ( -2.870125741905210415, 6.929096494179677990, 6.853487500180309056 ) ) ;
#19673=CARTESIAN_POINT ( 'NONE',  ( 2.943691925285397470, -14.79893867793683349, 2.758926831519074696 ) ) ;
#19687=CARTESIAN_POINT ( 'NONE',  ( -3.580422610670017658, 18.00000000043040771, 18.75316875018031126 ) ) ;
#19689=EDGE_LOOP ( 'NONE', ( #3674, #3667, #16209, #13454 ) ) ;
#19699=CARTESIAN_POINT ( 'NONE',  ( 7.500000000000007994, -9.015933403756345817E-10, 25.48870000018031590 ) ) ;
#19701=AXIS2_PLACEMENT_3D ( 'NONE', #11861, #8579, #20010 ) ;
#19702=CARTESIAN_POINT ( 'NONE',  ( 2.222972768810837163, -11.17563879758427525, 11.43160899971319822 ) ) ;
#19709=CARTESIAN_POINT ( 'NONE',  ( -6.888301784570738384, -16.62983158437509346, 16.82886250018031404 ) ) ;
#19724=ADVANCED_FACE ( 'NONE', ( #6704 ), #11697, .F. ) ;
#19727=SHAPE_REPRESENTATION_RELATIONSHIP ( 'NONE' , 'NONE' ,  #9416, #7446 ) ;
#19731=CARTESIAN_POINT ( 'NONE',  ( -1.491842754445841246, 7.500000000179339210, 7.148018750180312963 ) ) ;
#19742=CARTESIAN_POINT ( 'NONE',  ( -6.888301784570738384, -16.62983158437509346, 14.92426250018031375 ) ) ;
#19751=DIRECTION ( 'NONE',  ( 0.000000000000000000, 0.000000000000000000, -1.000000000000000000 ) ) ;
#19756=CARTESIAN_POINT ( 'NONE',  ( -7.902369978624331104, -7.902369976724401113, 1.176984750647428468 ) ) ;
#19758=DIRECTION ( 'NONE',  ( 1.202124453834178081E-10, 1.000000000000000000, 0.000000000000000000 ) ) ;
#19763=CARTESIAN_POINT ( 'NONE',  ( 15.25966316918061416, -10.19618095414378622, 5.342143750180314399 ) ) ;
#19765=CARTESIAN_POINT ( 'NONE',  ( 6.250000000000054179, 10.82531754730546147, 43.00000000000000000 ) ) ;
#19768=AXIS2_PLACEMENT_3D ( 'NONE', #16255, #10101, #17952 ) ;
#19779=CARTESIAN_POINT ( 'NONE',  ( -10.46442989454075878, -10.46442989202484242, 19.27466691884154670 ) ) ;
#19784=CARTESIAN_POINT ( 'NONE',  ( -15.25966316918061416, 10.19618095414378445, 17.57504375018031340 ) ) ;
#19785=VERTEX_POINT ( 'NONE', #17176 ) ;
#19790=CARTESIAN_POINT ( 'NONE',  ( -1.491842756249033286, -7.499999999820668783, 9.289481250180315897 ) ) ;
#19793=CARTESIAN_POINT ( 'NONE',  ( -6.888301784570736608, -16.62983158437509346, 14.92426250018031020 ) ) ;
#19796=ORIENTED_EDGE ( 'NONE', *, *, #8285, .T. ) ;
#19801=CARTESIAN_POINT ( 'NONE',  ( -2.163827323447878648E-09, -18.00000000000000355, 16.23980000018031333 ) ) ;
#19804=CARTESIAN_POINT ( 'NONE',  ( 7.902369976724399336, -7.902369978624331104, -20.02926524935257646 ) ) ;
#19807=CARTESIAN_POINT ( 'NONE',  ( -10.32494394809439164, -4.276731812588563386, -14.78167225028680676 ) ) ;
#19814=CARTESIAN_POINT ( 'NONE',  ( 12.72792205982779734, -12.72792206288791128, -3.788324999819688177 ) ) ;
#19841=CARTESIAN_POINT ( 'NONE',  ( -2.870125741905213079, 6.929096494179683319, 3.693387500180313143 ) ) ;
#19857=CARTESIAN_POINT ( 'NONE',  ( -10.19618095414378445, -15.25966316918061239, -13.05620624981969513 ) ) ;
#19859=ADVANCED_FACE ( 'NONE', ( #13228 ), #5160, .F. ) ;
#19862=CARTESIAN_POINT ( 'NONE',  ( -6.330490858644140850, -9.474249097082498849, 0.8824535006474282239 ) ) ;
#19872=CARTESIAN_POINT ( 'NONE',  ( -12.72792206288791128, -12.72792205982779912, -1.432074999819687333 ) ) ;
#19887=CARTESIAN_POINT ( 'NONE',  ( 5.663308650141532397, 13.67243654642775574, 13.97310441884154564 ) ) ;
#19892=CARTESIAN_POINT ( 'NONE',  ( -10.19618095047497874, 15.25966317163202746, 18.16410625018031411 ) ) ;
#19894=ORIENTED_EDGE ( 'NONE', *, *, #1806, .T. ) ;
#19895=EDGE_CURVE ( 'NONE', #1438, #9255, #12510, .T. ) ;
#19901=CARTESIAN_POINT ( 'NONE',  ( -15.25966316918061416, 10.19618095414378445, -1.274956249819690024 ) ) ;
#19907=CARTESIAN_POINT ( 'NONE',  ( -6.358192987158597376, 4.248408730893249441, -16.04020624981968624 ) ) ;
#19908=CARTESIAN_POINT ( 'NONE',  ( 5.303300859536635770, 5.303300858261589923, -3.964424999819686324 ) ) ;
#19909=AXIS2_PLACEMENT_3D ( 'NONE', #17296, #4362, #15589 ) ;
#19910=CARTESIAN_POINT ( 'NONE',  ( 9.474249097082495297, -6.330490858644137298, -8.596516000286802850 ) ) ;
#19916=CARTESIAN_POINT ( 'NONE',  ( 16.62983158603122291, 6.888301780572502864, 3.869487500180311734 ) ) ;
#19918=ORIENTED_EDGE ( 'NONE', *, *, #6643, .F. ) ;
#19926=EDGE_CURVE ( 'NONE', #100, #1825, #11393, .T. ) ;
#19927=( NAMED_UNIT ( * ) PLANE_ANGLE_UNIT ( ) SI_UNIT ( $, .RADIAN. ) );
#19930=CARTESIAN_POINT ( 'NONE',  ( 4.248408729364575365, -6.358192988180014993, 1.846456250180310565 ) ) ;
#19933=DIRECTION ( 'NONE',  ( -0.5000000000000037748, -0.8660254037844364872, 0.000000000000000000 ) ) ;
#19935=VERTEX_POINT ( 'NONE', #13754 ) ;
#19938=CARTESIAN_POINT ( 'NONE',  ( 18.00000000043041126, 3.580422610670019434, 2.259418750180313129 ) ) ;
#19943=CARTESIAN_POINT ( 'NONE',  ( 6.249999999999902300, -10.82531754730554496, -43.00000000000000000 ) ) ;
#19949=CARTESIAN_POINT ( 'NONE',  ( 6.888301784570727726, 16.62983158437509701, -8.638237499819693355 ) ) ;
#19955=CARTESIAN_POINT ( 'NONE',  ( -4.276731812588566939, 10.32494394809439875, 4.122297250647427802 ) ) ;
#19957=DIRECTION ( 'NONE',  ( -1.000000000000000000, 1.202124453834178081E-10, 0.000000000000000000 ) ) ;
#19960=ORIENTED_EDGE ( 'NONE', *, *, #12128, .T. ) ;
#19961=CARTESIAN_POINT ( 'NONE',  ( 6.888301780572507305, -16.62983158603121936, -3.199262499819687022 ) ) ;
#19976=CARTESIAN_POINT ( 'NONE',  ( -14.79893867722910628, 2.943691928843437111, 20.74732316884154670 ) ) ;
#19981=CARTESIAN_POINT ( 'NONE',  ( 8.382925368423265411, -12.54593441764187034, -16.68013566848092566 ) ) ;
#19989=CARTESIAN_POINT ( 'NONE',  ( 4.248408729364579806, -6.358192988180021210, 8.111356250180314476 ) ) ;
#19992=CARTESIAN_POINT ( 'NONE',  ( 12.72792206288790773, 12.72792205982779912, 1.375825000180311175 ) ) ;
#20000=CARTESIAN_POINT ( 'NONE',  ( 1.491842756249030399, 7.499999999820669672, -14.27301874981969121 ) ) ;
#20004=CARTESIAN_POINT ( 'NONE',  ( -9.015947181032835626E-10, -7.500000000000007994, -9.855049999819689432 ) ) ;
#20005=CARTESIAN_POINT ( 'NONE',  ( -7.902369976724391343, 7.902369978624323110, -22.43948475028680889 ) ) ;
#20010=DIRECTION ( 'NONE',  ( -1.000000000000000000, 0.000000000000000000, 0.000000000000000000 ) ) ;
#20011=CARTESIAN_POINT ( 'NONE',  ( -16.62983158437510056, 6.888301784570729502, 0.3351125001803123560 ) ) ;
#20019=ORIENTED_EDGE ( 'NONE', *, *, #7645, .F. ) ;
#20025=CIRCLE ( 'NONE', #10573, 2.650000000000000355 ) ;
#20028=CARTESIAN_POINT ( 'NONE',  ( 6.249999999999902300, -10.82531754730554496, 43.00000000000000000 ) ) ;
#20029=CARTESIAN_POINT ( 'NONE',  ( -6.929096494179677101, -2.870125741905209527, -14.35276249981968988 ) ) ;
#20035=CARTESIAN_POINT ( 'NONE',  ( 7.500000000000007105, 4.207617034055637320E-15, 6.638700000002313750 ) ) ;
#20036=VERTEX_POINT ( 'NONE', #13648 ) ;
#20037=CARTESIAN_POINT ( 'NONE',  ( 15.25966317163202746, 10.19618095047498407, 11.09535625018031446 ) ) ;
#20040=EDGE_LOOP ( 'NONE', ( #8192, #11983, #10572, #4350 ) ) ;
#20043=ORIENTED_EDGE ( 'NONE', *, *, #11853, .F. ) ;
#20052=CARTESIAN_POINT ( 'NONE',  ( 12.72792206288790773, 12.72792205982779912, -17.47417499981969513 ) ) ;
#20055=CARTESIAN_POINT ( 'NONE',  ( 2.222972768810839383, -11.17563879758428769, -0.2956714993525706436 ) ) ;
#20065=EDGE_CURVE ( 'NONE', #10032, #20507, #18519, .T. ) ;
#20066=CARTESIAN_POINT ( 'NONE',  ( 17.99999999956958163, -3.580422614997676334, 4.753081250180313688 ) ) ;
#20082=CARTESIAN_POINT ( 'NONE',  ( 5.663308646854342321, -13.67243654778935635, 17.50747941884155168 ) ) ;
#20087=AXIS2_PLACEMENT_3D ( 'NONE', #20028, #4026, #16962 ) ;
#20090=CARTESIAN_POINT ( 'NONE',  ( 2.163825119083639120E-09, 17.99999999999999645, 19.04770000018030984 ) ) ;
#20103=CARTESIAN_POINT ( 'NONE',  ( 10.19618095047497697, -15.25966317163202923, 4.026606250180309488 ) ) ;
#20112=CARTESIAN_POINT ( 'NONE',  ( -12.72792205982780089, 12.72792206288791128, 19.77417500018031049 ) ) ;
#20116=CARTESIAN_POINT ( 'NONE',  ( 7.499999999820668783, -1.491842756249033508, 6.933231250180315719 ) ) ;
#20118=CARTESIAN_POINT ( 'NONE',  ( -4.276731815070945686, -10.32494394706615637, -6.534797250286804804 ) ) ;
#20124=CARTESIAN_POINT ( 'NONE',  ( -16.62983158603122291, -6.888301780572501087, -10.26801249981968844 ) ) ;
#20128=ORIENTED_EDGE ( 'NONE', *, *, #9370, .F. ) ;
#20131=ORIENTED_EDGE ( 'NONE', *, *, #16960, .T. ) ;
#20137=CARTESIAN_POINT ( 'NONE',  ( 9.015937996181834148E-10, 7.500000000000000888, -1.982449999819689612 ) ) ;
#20142=CARTESIAN_POINT ( 'NONE',  ( -4.248408729364580694, 6.358192988180020322, 3.398856250180316341 ) ) ;
#20145=CARTESIAN_POINT ( 'NONE',  ( 6.888301780572507305, -16.62983158603121936, 4.321137500180313396 ) ) ;
#20151=CIRCLE ( 'NONE', #11030, 2.649999999999999467 ) ;
#20159=CARTESIAN_POINT ( 'NONE',  ( 17.99999999999999645, -2.163824016901520184E-09, -16.29604999981969371 ) ) ;
#20162=CIRCLE ( 'NONE', #2588, 2.649999999999999467 ) ;
#20164=CARTESIAN_POINT ( 'NONE',  ( -4.276731815070949239, -10.32494394706616347, -18.26207774935257078 ) ) ;
#20174=CARTESIAN_POINT ( 'NONE',  ( 10.19618095047497874, -15.25966317163203279, 5.931206250180311557 ) ) ;
#20182=CARTESIAN_POINT ( 'NONE',  ( -5.303300858261589035, 5.303300859536635770, 12.52932500018031448 ) ) ;
#20190=EDGE_CURVE ( 'NONE', #1625, #17634, #15480, .T. ) ;
#20194=CARTESIAN_POINT ( 'NONE',  ( -5.663308646854337880, 13.67243654778935991, 3.369979418841543506 ) ) ;
#20202=CARTESIAN_POINT ( 'NONE',  ( -5.663308650141535949, -13.67243654642774686, -24.63247941848092637 ) ) ;
#20204=ORIENTED_EDGE ( 'NONE', *, *, #19895, .F. ) ;
#20212=CARTESIAN_POINT ( 'NONE',  ( -3.580422610670017658, 18.00000000043040771, 9.328168750180312330 ) ) ;
#20223=CARTESIAN_POINT ( 'NONE',  ( -15.25966317163203456, -10.19618095047498230, 17.71245625018031333 ) ) ;
#20227=CARTESIAN_POINT ( 'NONE',  ( 6.929096493489630859, -2.870125743571144472, -2.197237499819686857 ) ) ;
#20230=CARTESIAN_POINT ( 'NONE',  ( -2.222972771497743416, -11.17563879704981566, -6.829328500286805159 ) ) ;
#20234=CYLINDRICAL_SURFACE ( 'NONE', #76, 7.500000000000000000 ) ;
#20235=CARTESIAN_POINT ( 'NONE',  ( 3.580422614997668340, 17.99999999956958519, 2.396831250180312622 ) ) ;
#20251=CARTESIAN_POINT ( 'NONE',  ( 1.491842754445842134, -7.500000000179339210, -6.989481249819688102 ) ) ;
#20253=DIRECTION ( 'NONE',  ( -0.000000000000000000, -0.000000000000000000, 1.000000000000000000 ) ) ;
#20258=CARTESIAN_POINT ( 'NONE',  ( -10.19618095414378622, -15.25966316918061416, 5.793793750180313396 ) ) ;
#20269=CARTESIAN_POINT ( 'NONE',  ( 10.19618095414378622, 15.25966316918061239, -8.343706249819691223 ) ) ;
#20272=CARTESIAN_POINT ( 'NONE',  ( -1.343452921478824119E-09, -11.17563879731705789, -9.426140249352577882 ) ) ;
#20278=EDGE_LOOP ( 'NONE', ( #16087, #18445 ) ) ;
#20279=CARTESIAN_POINT ( 'NONE',  ( -6.888301780572501976, 16.62983158603122291, -7.911762499819688266 ) ) ;
#20291=CARTESIAN_POINT ( 'NONE',  ( -2.943691928843437999, -14.79893867722910450, -0.4589268311584565052 ) ) ;
#20297=CARTESIAN_POINT ( 'NONE',  ( 6.888301784570727726, 16.62983158437509701, 10.21176250018031162 ) ) ;
#20310=CARTESIAN_POINT ( 'NONE',  ( 15.25966316918061239, -10.19618095414378445, -15.41245624981969087 ) ) ;
#20319=CARTESIAN_POINT ( 'NONE',  ( -3.580422610670018990, 18.00000000043041481, 11.23276875018031085 ) ) ;
#20320=CARTESIAN_POINT ( 'NONE',  ( 4.248408730893249441, 6.358192987158595599, -13.68395624981969050 ) ) ;
#20322=ORIENTED_EDGE ( 'NONE', *, *, #7645, .T. ) ;
#20324=CARTESIAN_POINT ( 'NONE',  ( 14.79893867793683349, 2.943691925285396582, 19.25267683151907505 ) ) ;
#20328=LINE ( 'NONE', #15475, #3776 ) ;
#20330=CARTESIAN_POINT ( 'NONE',  ( -16.62983158437510056, 6.888301784570729502, -18.51488749981968951 ) ) ;
#20334=ORIENTED_EDGE ( 'NONE', *, *, #5970, .T. ) ;
#20340=EDGE_LOOP ( 'NONE', ( #12154, #14910 ) ) ;
#20341=DIRECTION ( 'NONE',  ( -0.4999999999999918954, 0.8660254037844433705, 0.000000000000000000 ) ) ;
#20350=CARTESIAN_POINT ( 'NONE',  ( 6.929096494179676213, 2.870125741905210415, -9.640262499819689523 ) ) ;
#20361=CARTESIAN_POINT ( 'NONE',  ( -6.888301780572501976, 16.62983158603122291, 9.033637500180313751 ) ) ;
#20372=CARTESIAN_POINT ( 'NONE',  ( 7.500000000000000000, -9.015933403756339613E-10, -21.63629999981969121 ) ) ;
#20377=CARTESIAN_POINT ( 'NONE',  ( -12.72792205982779556, 12.72792206288790773, -19.83042499981969087 ) ) ;
#20392=CARTESIAN_POINT ( 'NONE',  ( -6.888301784570738384, -16.62983158437509346, -11.44613749981969164 ) ) ;
#20399=ORIENTED_EDGE ( 'NONE', *, *, #16960, .F. ) ;
#20408=CARTESIAN_POINT ( 'NONE',  ( 8.382925371439633011, 12.54593441562640876, -4.582364331158456316 ) ) ;
#20415=CARTESIAN_POINT ( 'NONE',  ( -10.19618095047497874, 15.25966317163202746, 8.739106250180311619 ) ) ;
#20418=AXIS2_PLACEMENT_3D ( 'NONE', #17563, #6202, #12797 ) ;
#20428=CARTESIAN_POINT ( 'NONE',  ( 12.72792205982779379, -12.72792206288790950, -5.692924999819690690 ) ) ;
#20438=CARTESIAN_POINT ( 'NONE',  ( 18.00000000000000355, -2.163824016901520597E-09, 4.458550000180308892 ) ) ;
#20443=CARTESIAN_POINT ( 'NONE',  ( -7.500000000000007994, 9.015942588607339023E-10, -16.92379999981968908 ) ) ;
#20445=CARTESIAN_POINT ( 'NONE',  ( -1.491842756249033286, -7.499999999820668783, 18.71448125018031661 ) ) ;
#20446=CARTESIAN_POINT ( 'NONE',  ( -2.222972771497743416, -11.17563879704981566, -25.67932850028680747 ) ) ;
#20451=CARTESIAN_POINT ( 'NONE',  ( 18.00000000043041126, 3.580422610670019434, -14.68598124981969022 ) ) ;
#20466=CARTESIAN_POINT ( 'NONE',  ( -7.500000000179339210, -1.491842754445842800, -23.48323124981969201 ) ) ;
#20468=CARTESIAN_POINT ( 'NONE',  ( 9.470358143689576735, -1.138454911109686870E-09, -11.01577170245055370 ) ) ;
#20474=CARTESIAN_POINT ( 'NONE',  ( -16.62983158603122291, -6.888301780572501087, -12.17261249981968874 ) ) ;
#20489=ADVANCED_FACE ( 'NONE', ( #7657 ), #14033, .T. ) ;
#20492=VERTEX_POINT ( 'NONE', #20793 ) ;
#20502=CARTESIAN_POINT ( 'NONE',  ( 10.19618095047497874, -15.25966317163203279, -12.91879374981968631 ) ) ;
#20507=VERTEX_POINT ( 'NONE', #7764 ) ;
#20515=EDGE_CURVE ( 'NONE', #19384, #7136, #7978, .T. ) ;
#20517=CARTESIAN_POINT ( 'NONE',  ( 12.54593441764187567, 8.382925368423276069, 5.431698168841543328 ) ) ;
#20518=VERTEX_POINT ( 'NONE', #10839 ) ;
#20523=CARTESIAN_POINT ( 'NONE',  ( -15.25966316918061416, 10.19618095414378445, 8.150043750180310909 ) ) ;
#20524=VECTOR ( 'NONE', #10722, 1000.000000000000000 ) ;
#20525=CARTESIAN_POINT ( 'NONE',  ( 1.491842756249029289, 7.499999999820664343, -20.53791874981969912 ) ) ;
#20534=CARTESIAN_POINT ( 'NONE',  ( 4.248408729364576253, -6.358192988180015881, 1.846456250180306791 ) ) ;
#20535=CARTESIAN_POINT ( 'NONE',  ( 12.72792205982779379, -12.72792206288790950, -15.11792499981969051 ) ) ;
#20545=CARTESIAN_POINT ( 'NONE',  ( -18.00000000043041481, -3.580422610670022987, 8.876518750180311557 ) ) ;
#20547=CARTESIAN_POINT ( 'NONE',  ( 6.358192988180019434, 4.248408729364581582, -13.09489374981968801 ) ) ;
#20550=CARTESIAN_POINT ( 'NONE',  ( -12.54593441764187034, -8.382925368423267187, 4.526114331519074163 ) ) ;
#20555=CARTESIAN_POINT ( 'NONE',  ( 0.000000000000000000, 0.000000000000000000, -40.00000000000000000 ) ) ;
#20557=CARTESIAN_POINT ( 'NONE',  ( 3.580422610670020322, -18.00000000043041126, -21.75473124981968809 ) ) ;
#20566=ORIENTED_EDGE ( 'NONE', *, *, #5075, .T. ) ;
#20570=CARTESIAN_POINT ( 'NONE',  ( -7.500000000000000000, 0.000000000000000000, 40.00000000000000000 ) ) ;
#20573=DIRECTION ( 'NONE',  ( -1.000000000000000000, 0.000000000000000000, 0.000000000000000000 ) ) ;
#20574=CARTESIAN_POINT ( 'NONE',  ( -9.474249098604506258, -6.330490856366290053, 13.19879649971320035 ) ) ;
#20578=ORIENTED_EDGE ( 'NONE', *, *, #9161, .F. ) ;
#20581=CARTESIAN_POINT ( 'NONE',  ( 16.62983158437509346, -6.888301784570739272, -15.70698749981968767 ) ) ;
#20586=EDGE_LOOP ( 'NONE', ( #4854, #4295, #10351, #9440 ) ) ;
#20593=CARTESIAN_POINT ( 'NONE',  ( -2.163827323447877821E-09, -17.99999999999999645, -23.36479999981969158 ) ) ;
#20603=CARTESIAN_POINT ( 'NONE',  ( 3.580422614997668340, 17.99999999956958519, -16.45316874981969235 ) ) ;
#20613=EDGE_CURVE ( 'NONE', #9255, #1354, #9661, .T. ) ;
#20616=CARTESIAN_POINT ( 'NONE',  ( -12.54593441764187745, -8.382925368423274293, 0.7191981688415456375 ) ) ;
#20618=CARTESIAN_POINT ( 'NONE',  ( 18.00000000000000000, -2.163824016901520184E-09, -23.81644999981969235 ) ) ;
#20623=CARTESIAN_POINT ( 'NONE',  ( 2.163825119083639120E-09, 17.99999999999999645, 9.622700000180310909 ) ) ;
#20624=LINE ( 'NONE', #2825, #2067 ) ;
#20635=CARTESIAN_POINT ( 'NONE',  ( -15.25966316918061416, 10.19618095414378445, -20.12495624981969300 ) ) ;
#20642=CARTESIAN_POINT ( 'NONE',  ( 10.19618095414378978, 15.25966316918061771, 12.41089375018030871 ) ) ;
#20647=CARTESIAN_POINT ( 'NONE',  ( 1.779017513685135741E-09, 14.79893867758296544, 17.19095808151907789 ) ) ;
#20665=FACE_OUTER_BOUND ( 'NONE', #19154, .T. ) ;
#20666=CARTESIAN_POINT ( 'NONE',  ( 6.330490856366294494, -9.474249098604513364, -10.30973399935257007 ) ) ;
#20667=CARTESIAN_POINT ( 'NONE',  ( 6.358192988180013216, 4.248408729364577141, -19.35979374981969059 ) ) ;
#20674=CARTESIAN_POINT ( 'NONE',  ( 12.72792206288790950, 12.72792205982780089, -17.47417499981969158 ) ) ;
#20700=CARTESIAN_POINT ( 'NONE',  ( 15.25966317163202746, 10.19618095047498407, -15.27504374981969093 ) ) ;
#20713=CARTESIAN_POINT ( 'NONE',  ( 14.79893867758297610, -1.779016607511492805E-09, -21.95970808115845685 ) ) ;
#20715=ORIENTED_EDGE ( 'NONE', *, *, #3539, .T. ) ;
#20726=DIRECTION ( 'NONE',  ( 1.000000000000000000, 0.000000000000000000, 0.000000000000000000 ) ) ;
#20733=CARTESIAN_POINT ( 'NONE',  ( 10.19618095047497697, -15.25966317163202923, -5.398393749819690335 ) ) ;
#20742=CARTESIAN_POINT ( 'NONE',  ( -16.62983158437510411, 6.888301784570731279, 9.760112500180310846 ) ) ;
#20745=CARTESIAN_POINT ( 'NONE',  ( 4.248408729364579806, -6.358192988180021210, -10.73864374981968517 ) ) ;
#20749=CARTESIAN_POINT ( 'NONE',  ( 10.46442989454075168, 10.46442989202483886, 8.944083081519076828 ) ) ;
#20758=VECTOR ( 'NONE', #17290, 1000.000000000000000 ) ;
#20762=CARTESIAN_POINT ( 'NONE',  ( 6.249999999999902300, -10.82531754730554496, 40.00000000000000000 ) ) ;
#20775=CARTESIAN_POINT ( 'NONE',  ( 7.575000000000064126, 13.12028486733421850, -40.00000000000000000 ) ) ;
#20776=CARTESIAN_POINT ( 'NONE',  ( -10.32494394706616703, 4.276731815070943910, -15.90582774935257682 ) ) ;
#20779=CARTESIAN_POINT ( 'NONE',  ( -7.902369976724391343, 7.902369978624323110, 15.26051524971320283 ) ) ;
#20787=CARTESIAN_POINT ( 'NONE',  ( 10.19618095047497874, -15.25966317163203279, -14.82339374981968483 ) ) ;
#20790=LINE ( 'NONE', #6273, #11305 ) ;
#20793=CARTESIAN_POINT ( 'NONE',  ( 3.600000000000054712, 10.82531754730546147, 40.00000000000000000 ) ) ;
#20794=DIRECTION ( 'NONE',  ( -0.000000000000000000, -0.000000000000000000, 1.000000000000000000 ) ) ;
#20799=DIRECTION ( 'NONE',  ( -0.000000000000000000, -0.000000000000000000, 1.000000000000000000 ) ) ;
#20801=CARTESIAN_POINT ( 'NONE',  ( 0.000000000000000000, 0.000000000000000000, 43.00000000000000000 ) ) ;
#20803=CARTESIAN_POINT ( 'NONE',  ( 7.500000000000000000, 9.184850993605147944E-16, 40.00000000000000000 ) ) ;
#20810=ORIENTED_EDGE ( 'NONE', *, *, #18575, .F. ) ;
#20825=CARTESIAN_POINT ( 'NONE',  ( 2.222972771497741640, 11.17563879704982988, 23.85589100064743207 ) ) ;
#20829=FACE_BOUND ( 'NONE', #20278, .T. ) ;
#20831=CARTESIAN_POINT ( 'NONE',  ( -2.870125743571141808, -6.929096493489625530, -24.95588749981969201 ) ) ;
#20835=ORIENTED_EDGE ( 'NONE', *, *, #294, .T. ) ;
#20844=CARTESIAN_POINT ( 'NONE',  ( 15.25966316918061239, -10.19618095414378445, -24.83745624981969513 ) ) ;
#20846=CARTESIAN_POINT ( 'NONE',  ( 5.303300858261588147, -5.303300859536636658, -11.03317499981968552 ) ) ;
#20850=CARTESIAN_POINT ( 'NONE',  ( 6.888301780572508193, -16.62983158603122291, -12.62426249981968951 ) ) ;
#20853=CARTESIAN_POINT ( 'NONE',  ( 7.500000000000003553, 1.491842754878801580, 9.504268750087788931 ) ) ;
#20857=CARTESIAN_POINT ( 'NONE',  ( 13.67243654778934925, 5.663308646854335215, -9.316854418480929212 ) ) ;
#20880=PRODUCT_DEFINITION ( 'UNKNOWN', '', #3877, #8995 ) ;
#20881=CARTESIAN_POINT ( 'NONE',  ( -11.17563879758428769, -2.222972768810840272, -16.78942149935257788 ) ) ;
#20883=CARTESIAN_POINT ( 'NONE',  ( -2.870125741905209971, 6.929096494179676213, -21.42151249981968775 ) ) ;
#20894=CARTESIAN_POINT ( 'NONE',  ( 18.00000000043041126, 3.580422610670019434, -7.165581249819687137 ) ) ;
#20899=CARTESIAN_POINT ( 'NONE',  ( 7.500000000000000000, -1.491842755816076060, -8.756668749912215333 ) ) ;
#20912=CARTESIAN_POINT ( 'NONE',  ( -7.500000000000009770, -1.491842754878800248, 1.631668750087792663 ) ) ;
#20929=CARTESIAN_POINT ( 'NONE',  ( 4.276731815070943910, 10.32494394706616703, 24.15042225064743420 ) ) ;
#20931=CARTESIAN_POINT ( 'NONE',  ( 7.500000000000004441, -8.788009009181406898E-15, -18.47619999999769647 ) ) ;
#20935=CARTESIAN_POINT ( 'NONE',  ( -6.888301780572501976, 16.62983158603122291, 20.36323750018031475 ) ) ;
#20940=FACE_BOUND ( 'NONE', #4393, .T. ) ;
ENDSEC;
END-ISO-10303-21;
